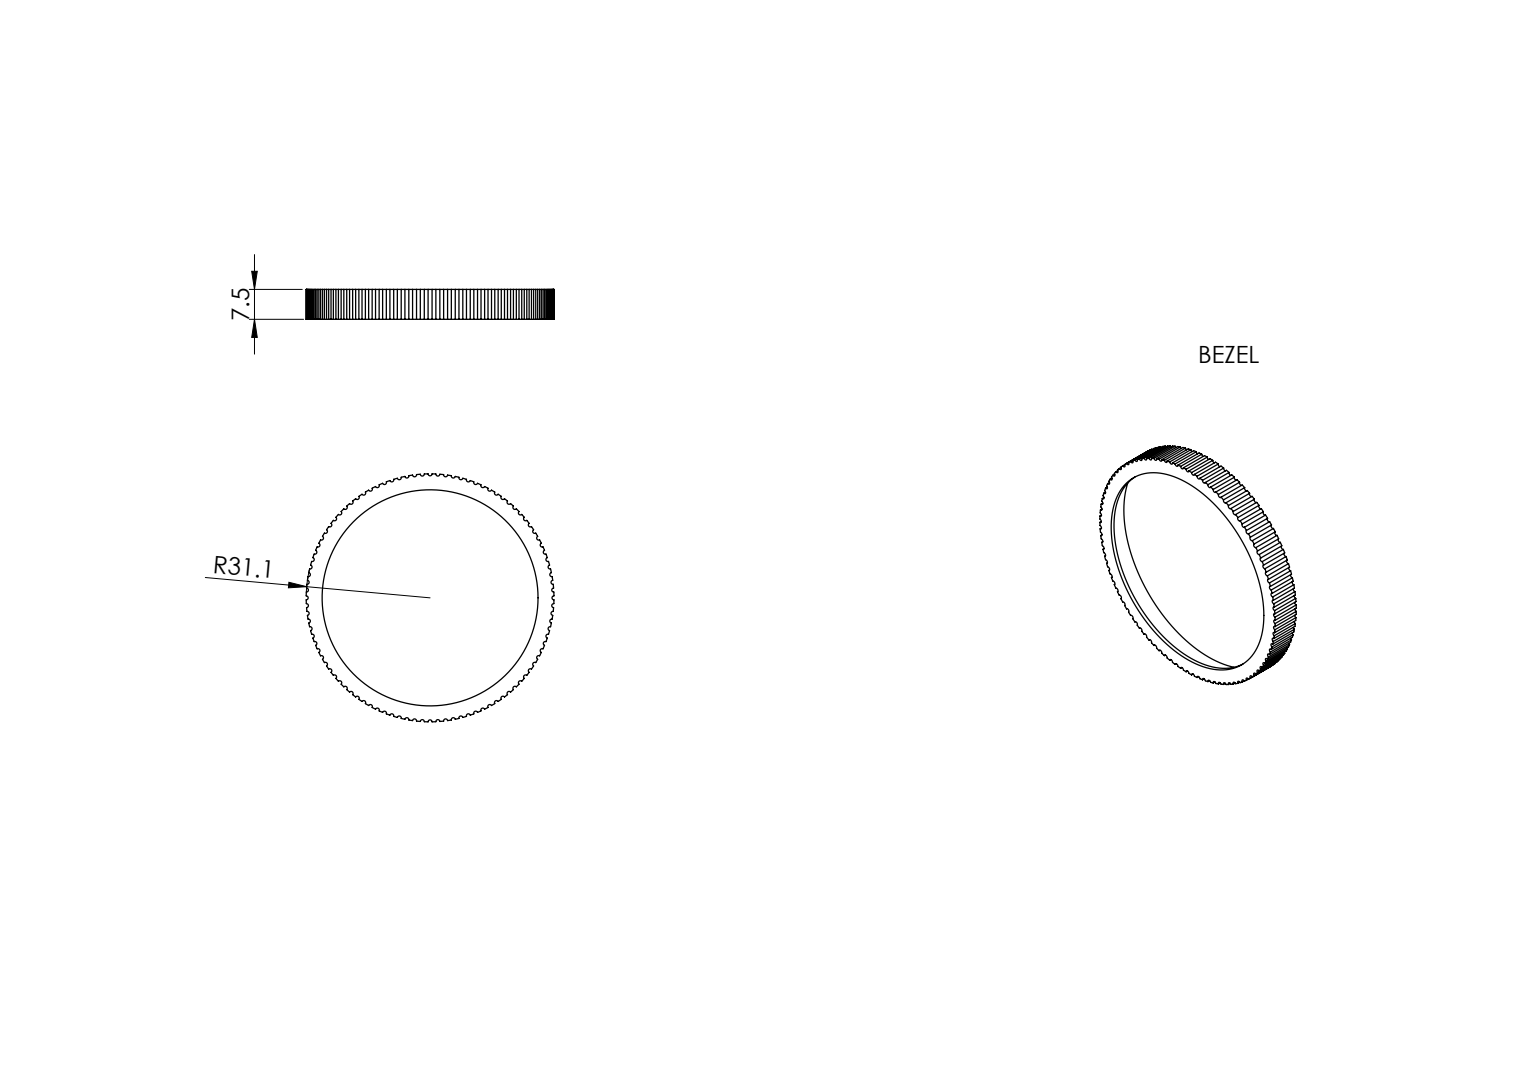
ISO-10303-21;
HEADER;
FILE_DESCRIPTION (('STEP AP214'),
    '1' );
FILE_NAME ('bezel.step',
    '2026-10-26T12:50:16',
    ( '' ),
    ( '' ),
    'SwSTEP 2.0',
    'SolidWorks 2026',
    '' );
FILE_SCHEMA (( 'AUTOMOTIVE_DESIGN' ));
ENDSEC;

DATA;
#1=AXIS2_PLACEMENT_3D ( 'NONE', #24942, #2719, #13181 ) ;
#6=AXIS2_PLACEMENT_3D ( 'NONE', #4398, #870, #8851 ) ;
#12=DIRECTION ( 'NONE',  ( 1.000000000000000000, 0.000000000000000000, 0.000000000000000000 ) ) ;
#17=CIRCLE ( 'NONE', #17974, 0.5000000000000003331 ) ;
#18=CARTESIAN_POINT ( 'NONE',  ( 0.000000000000000000, 0.000000000000000000, 1.000000000000000000 ) ) ;
#20=ORIENTED_EDGE ( 'NONE', *, *, #7327, .F. ) ;
#25=ORIENTED_EDGE ( 'NONE', *, *, #21709, .F. ) ;
#27=VERTEX_POINT ( 'NONE', #19559 ) ;
#31=AXIS2_PLACEMENT_3D ( 'NONE', #2511, #8267, #24218 ) ;
#35=CIRCLE ( 'NONE', #17990, 0.5000000000000006661 ) ;
#39=CIRCLE ( 'NONE', #22153, 31.10000000000000142 ) ;
#47=CIRCLE ( 'NONE', #3373, 31.10000000000000142 ) ;
#49=CARTESIAN_POINT ( 'NONE',  ( -10.98232076577242466, -29.09636799667071116, 1.000000000000000000 ) ) ;
#51=VERTEX_POINT ( 'NONE', #10384 ) ;
#54=EDGE_CURVE ( 'NONE', #21865, #6150, #14230, .T. ) ;
#55=CIRCLE ( 'NONE', #14670, 0.5000000000000005551 ) ;
#60=CARTESIAN_POINT ( 'NONE',  ( -9.610428525061097460, -29.57785765677920509, -6.500000000000000000 ) ) ;
#63=VECTOR ( 'NONE', #7567, 1000.000000000000000 ) ;
#66=DIRECTION ( 'NONE',  ( 0.000000000000000000, 0.000000000000000000, 1.000000000000000000 ) ) ;
#70=AXIS2_PLACEMENT_3D ( 'NONE', #11835, #22027, #12224 ) ;
#72=DIRECTION ( 'NONE',  ( 1.000000000000000000, 0.000000000000000000, 0.000000000000000000 ) ) ;
#79=AXIS2_PLACEMENT_3D ( 'NONE', #15726, #13515, #3680 ) ;
#81=DIRECTION ( 'NONE',  ( 0.000000000000000000, 0.000000000000000000, 1.000000000000000000 ) ) ;
#83=CARTESIAN_POINT ( 'NONE',  ( -23.01025686871652809, -20.92219106202034595, 1.000000000000000000 ) ) ;
#86=CIRCLE ( 'NONE', #1339, 31.10000000000000142 ) ;
#89=VERTEX_POINT ( 'NONE', #21923 ) ;
#95=AXIS2_PLACEMENT_3D ( 'NONE', #9918, #10180, #22078 ) ;
#97=CYLINDRICAL_SURFACE ( 'NONE', #3366, 0.5000000000000004441 ) ;
#98=ORIENTED_EDGE ( 'NONE', *, *, #19921, .T. ) ;
#99=ORIENTED_EDGE ( 'NONE', *, *, #21927, .F. ) ;
#100=ADVANCED_FACE ( 'NONE', ( #14466 ), #6356, .T. ) ;
#105=EDGE_CURVE ( 'NONE', #8835, #13216, #4631, .T. ) ;
#106=CIRCLE ( 'NONE', #18070, 0.4999999999999998890 ) ;
#107=EDGE_CURVE ( 'NONE', #585, #4269, #18005, .T. ) ;
#112=AXIS2_PLACEMENT_3D ( 'NONE', #10691, #2608, #22745 ) ;
#117=ORIENTED_EDGE ( 'NONE', *, *, #18852, .F. ) ;
#129=DIRECTION ( 'NONE',  ( 1.000000000000000000, 0.000000000000000000, 0.000000000000000000 ) ) ;
#131=ORIENTED_EDGE ( 'NONE', *, *, #19522, .T. ) ;
#132=VERTEX_POINT ( 'NONE', #22432 ) ;
#134=DIRECTION ( 'NONE',  ( 0.2486898871648519360, -0.9685831611286318532, 0.000000000000000000 ) ) ;
#135=LINE ( 'NONE', #23787, #14039 ) ;
#136=EDGE_CURVE ( 'NONE', #11885, #9403, #6717, .T. ) ;
#138=CARTESIAN_POINT ( 'NONE',  ( 22.67092431280594056, 21.28941499438218088, 1.000000000000000000 ) ) ;
#145=DIRECTION ( 'NONE',  ( 0.000000000000000000, 0.000000000000000000, -1.000000000000000000 ) ) ;
#146=LINE ( 'NONE', #8118, #8436 ) ;
#147=CIRCLE ( 'NONE', #18512, 0.4999999999999997224 ) ;
#151=DIRECTION ( 'NONE',  ( -0.000000000000000000, 0.000000000000000000, 1.000000000000000000 ) ) ;
#154=AXIS2_PLACEMENT_3D ( 'NONE', #12888, #20866, #10658 ) ;
#157=ORIENTED_EDGE ( 'NONE', *, *, #19996, .F. ) ;
#158=DIRECTION ( 'NONE',  ( 0.4817536741017267032, 0.8763066800438573667, 0.000000000000000000 ) ) ;
#161=VERTEX_POINT ( 'NONE', #10530 ) ;
#163=ORIENTED_EDGE ( 'NONE', *, *, #23989, .T. ) ;
#164=ORIENTED_EDGE ( 'NONE', *, *, #21623, .F. ) ;
#169=CIRCLE ( 'NONE', #23535, 31.10000000000000142 ) ;
#170=EDGE_CURVE ( 'NONE', #5115, #14942, #12104, .T. ) ;
#179=DIRECTION ( 'NONE',  ( -0.000000000000000000, 0.000000000000000000, -1.000000000000000000 ) ) ;
#183=ORIENTED_EDGE ( 'NONE', *, *, #8865, .T. ) ;
#184=VERTEX_POINT ( 'NONE', #16301 ) ;
#187=DIRECTION ( 'NONE',  ( -0.000000000000000000, -0.000000000000000000, 1.000000000000000000 ) ) ;
#190=DIRECTION ( 'NONE',  ( -0.2486898871648584586, -0.9685831611286301879, 0.000000000000000000 ) ) ;
#191=ORIENTED_EDGE ( 'NONE', *, *, #21291, .T. ) ;
#193=ORIENTED_EDGE ( 'NONE', *, *, #13144, .T. ) ;
#199=DIRECTION ( 'NONE',  ( 0.000000000000000000, 0.000000000000000000, 1.000000000000000000 ) ) ;
#207=CARTESIAN_POINT ( 'NONE',  ( -30.85476721088022600, 3.897863563850190616, 1.000000000000000000 ) ) ;
#208=EDGE_CURVE ( 'NONE', #13339, #3186, #993, .T. ) ;
#209=DIRECTION ( 'NONE',  ( 0.000000000000000000, -0.000000000000000000, -1.000000000000000000 ) ) ;
#211=DIRECTION ( 'NONE',  ( 0.000000000000000000, -0.000000000000000000, 1.000000000000000000 ) ) ;
#226=DIRECTION ( 'NONE',  ( 0.000000000000000000, 0.000000000000000000, 1.000000000000000000 ) ) ;
#232=CARTESIAN_POINT ( 'NONE',  ( -30.12293631110050995, -7.734255490826679846, 1.000000000000000000 ) ) ;
#233=DIRECTION ( 'NONE',  ( 1.000000000000000000, 0.000000000000000000, 0.000000000000000000 ) ) ;
#239=EDGE_CURVE ( 'NONE', #21040, #20500, #15911, .T. ) ;
#240=ORIENTED_EDGE ( 'NONE', *, *, #11799, .T. ) ;
#242=FACE_OUTER_BOUND ( 'NONE', #14530, .T. ) ;
#244=ADVANCED_FACE ( 'NONE', ( #5041 ), #15120, .T. ) ;
#246=VERTEX_POINT ( 'NONE', #19148 ) ;
#250=ORIENTED_EDGE ( 'NONE', *, *, #20339, .T. ) ;
#252=CARTESIAN_POINT ( 'NONE',  ( 13.69242354489153080, 27.92360179968372691, -6.500000000000000000 ) ) ;
#254=DIRECTION ( 'NONE',  ( 0.000000000000000000, 0.000000000000000000, 1.000000000000000000 ) ) ;
#255=ORIENTED_EDGE ( 'NONE', *, *, #13059, .F. ) ;
#257=ORIENTED_EDGE ( 'NONE', *, *, #741, .T. ) ;
#259=CIRCLE ( 'NONE', #6931, 0.4999999999999998335 ) ;
#260=ORIENTED_EDGE ( 'NONE', *, *, #5301, .F. ) ;
#261=CARTESIAN_POINT ( 'NONE',  ( -10.08469938919519926, -29.41953157733083302, -6.500000000000000000 ) ) ;
#268=CARTESIAN_POINT ( 'NONE',  ( -29.57785765677917311, 9.610428525061202265, -6.500000000000000000 ) ) ;
#272=CARTESIAN_POINT ( 'NONE',  ( -23.96296185032681336, 19.82388608118453632, 1.000000000000000000 ) ) ;
#273=CARTESIAN_POINT ( 'NONE',  ( -19.82388608118446527, -23.96296185032687376, -6.500000000000000000 ) ) ;
#276=DIRECTION ( 'NONE',  ( 1.000000000000000000, 0.000000000000000000, 0.000000000000000000 ) ) ;
#281=ORIENTED_EDGE ( 'NONE', *, *, #13641, .F. ) ;
#286=ORIENTED_EDGE ( 'NONE', *, *, #2780, .F. ) ;
#289=CARTESIAN_POINT ( 'NONE',  ( 29.09636799667075024, -10.98232076577232519, -2.750000000000000000 ) ) ;
#296=LINE ( 'NONE', #16630, #5040 ) ;
#297=DIRECTION ( 'NONE',  ( 0.000000000000000000, -0.000000000000000000, 1.000000000000000000 ) ) ;
#299=DIRECTION ( 'NONE',  ( 1.000000000000000000, 0.000000000000000000, 0.000000000000000000 ) ) ;
#303=DIRECTION ( 'NONE',  ( 1.000000000000000000, 0.000000000000000000, 0.000000000000000000 ) ) ;
#306=EDGE_LOOP ( 'NONE', ( #6770, #6578, #10344, #18560 ) ) ;
#308=EDGE_CURVE ( 'NONE', #5737, #11616, #8580, .T. ) ;
#309=ORIENTED_EDGE ( 'NONE', *, *, #9443, .F. ) ;
#310=DIRECTION ( 'NONE',  ( 0.000000000000000000, -0.000000000000000000, 1.000000000000000000 ) ) ;
#313=ORIENTED_EDGE ( 'NONE', *, *, #21775, .T. ) ;
#317=DIRECTION ( 'NONE',  ( -0.000000000000000000, -0.000000000000000000, 1.000000000000000000 ) ) ;
#320=DIRECTION ( 'NONE',  ( 0.000000000000000000, 0.000000000000000000, 1.000000000000000000 ) ) ;
#321=FACE_OUTER_BOUND ( 'NONE', #5229, .T. ) ;
#326=CYLINDRICAL_SURFACE ( 'NONE', #16421, 0.5000000000000004441 ) ;
#327=DIRECTION ( 'NONE',  ( -0.000000000000000000, -0.000000000000000000, 1.000000000000000000 ) ) ;
#330=EDGE_CURVE ( 'NONE', #22681, #23712, #2540, .T. ) ;
#332=CARTESIAN_POINT ( 'NONE',  ( 0.000000000000000000, 0.000000000000000000, -6.500000000000000000 ) ) ;
#343=AXIS2_PLACEMENT_3D ( 'NONE', #22234, #14397, #10312 ) ;
#346=ORIENTED_EDGE ( 'NONE', *, *, #25545, .F. ) ;
#349=DIRECTION ( 'NONE',  ( -0.000000000000000000, -0.000000000000000000, 1.000000000000000000 ) ) ;
#351=ADVANCED_FACE ( 'NONE', ( #18768 ), #8839, .F. ) ;
#354=CARTESIAN_POINT ( 'NONE',  ( 18.68225429291731743, 24.86329371854767700, -2.750000000000000000 ) ) ;
#357=CARTESIAN_POINT ( 'NONE',  ( 0.000000000000000000, 0.000000000000000000, 0.000000000000000000 ) ) ;
#359=CARTESIAN_POINT ( 'NONE',  ( -28.41604871112473418, -11.44867358849319849, 1.000000000000000000 ) ) ;
#362=EDGE_CURVE ( 'NONE', #3397, #1343, #25563, .T. ) ;
#364=VERTEX_POINT ( 'NONE', #23208 ) ;
#366=CYLINDRICAL_SURFACE ( 'NONE', #12999, 31.10000000000000142 ) ;
#372=ORIENTED_EDGE ( 'NONE', *, *, #5336, .T. ) ;
#376=CARTESIAN_POINT ( 'NONE',  ( 0.000000000000000000, 0.000000000000000000, 1.000000000000000000 ) ) ;
#379=AXIS2_PLACEMENT_3D ( 'NONE', #21267, #11325, #1788 ) ;
#382=AXIS2_PLACEMENT_3D ( 'NONE', #14480, #16700, #6759 ) ;
#383=VERTEX_POINT ( 'NONE', #19283 ) ;
#387=CIRCLE ( 'NONE', #2056, 31.10000000000000142 ) ;
#390=EDGE_CURVE ( 'NONE', #22273, #20492, #21386, .T. ) ;
#394=CARTESIAN_POINT ( 'NONE',  ( 15.41874213889396117, -27.00874656207311020, 1.000000000000000000 ) ) ;
#395=AXIS2_PLACEMENT_3D ( 'NONE', #11615, #6002, #7707 ) ;
#396=CARTESIAN_POINT ( 'NONE',  ( 0.000000000000000000, 31.10000000000000142, -6.500000000000000000 ) ) ;
#399=DIRECTION ( 'NONE',  ( 1.000000000000000000, 0.000000000000000000, 0.000000000000000000 ) ) ;
#402=FACE_OUTER_BOUND ( 'NONE', #9294, .T. ) ;
#403=AXIS2_PLACEMENT_3D ( 'NONE', #22410, #18239, #9988 ) ;
#405=AXIS2_PLACEMENT_3D ( 'NONE', #13535, #2006, #15875 ) ;
#406=LINE ( 'NONE', #6283, #17518 ) ;
#407=CARTESIAN_POINT ( 'NONE',  ( -22.17092431280563503, 21.28941499438250062, -6.500000000000000000 ) ) ;
#411=ORIENTED_EDGE ( 'NONE', *, *, #12740, .F. ) ;
#414=VERTEX_POINT ( 'NONE', #11303 ) ;
#416=ORIENTED_EDGE ( 'NONE', *, *, #10693, .T. ) ;
#417=ORIENTED_EDGE ( 'NONE', *, *, #13846, .T. ) ;
#419=CIRCLE ( 'NONE', #13349, 31.10000000000000142 ) ;
#420=AXIS2_PLACEMENT_3D ( 'NONE', #4845, #24723, #6933 ) ;
#422=EDGE_CURVE ( 'NONE', #16170, #9403, #21906, .T. ) ;
#425=AXIS2_PLACEMENT_3D ( 'NONE', #20340, #2434, #1117 ) ;
#427=AXIS2_PLACEMENT_3D ( 'NONE', #1473, #13891, #21596 ) ;
#431=EDGE_CURVE ( 'NONE', #13647, #11427, #23332, .T. ) ;
#432=DIRECTION ( 'NONE',  ( -0.000000000000000000, -0.000000000000000000, 1.000000000000000000 ) ) ;
#433=AXIS2_PLACEMENT_3D ( 'NONE', #24646, #6868, #8833 ) ;
#436=LINE ( 'NONE', #14425, #4662 ) ;
#438=CIRCLE ( 'NONE', #9607, 0.4999999999999996114 ) ;
#441=VECTOR ( 'NONE', #4538, 1000.000000000000000 ) ;
#442=CARTESIAN_POINT ( 'NONE',  ( -3.897863563849436552, 30.85476721088031482, -6.500000000000000000 ) ) ;
#443=ORIENTED_EDGE ( 'NONE', *, *, #15873, .T. ) ;
#444=ORIENTED_EDGE ( 'NONE', *, *, #3058, .F. ) ;
#448=EDGE_LOOP ( 'NONE', ( #16828, #9714, #24335, #4332 ) ) ;
#450=ORIENTED_EDGE ( 'NONE', *, *, #18741, .F. ) ;
#451=DIRECTION ( 'NONE',  ( 0.7705132427757999114, 0.6374239897486768669, 0.000000000000000000 ) ) ;
#452=CARTESIAN_POINT ( 'NONE',  ( -31.03863125411922752, 1.952785157361987878, -6.500000000000000000 ) ) ;
#453=AXIS2_PLACEMENT_3D ( 'NONE', #20208, #10264, #5925 ) ;
#456=ADVANCED_FACE ( 'NONE', ( #9600 ), #3466, .T. ) ;
#460=EDGE_CURVE ( 'NONE', #51, #5651, #19861, .T. ) ;
#464=DIRECTION ( 'NONE',  ( -0.000000000000000000, -0.000000000000000000, 1.000000000000000000 ) ) ;
#472=VECTOR ( 'NONE', #23351, 1000.000000000000000 ) ;
#474=CIRCLE ( 'NONE', #15093, 0.4999999999999989453 ) ;
#480=ORIENTED_EDGE ( 'NONE', *, *, #22688, .F. ) ;
#483=CIRCLE ( 'NONE', #7586, 0.4999999999999987232 ) ;
#484=DIRECTION ( 'NONE',  ( -0.9685831611286283005, 0.2486898871648657861, 0.000000000000000000 ) ) ;
#485=VERTEX_POINT ( 'NONE', #25421 ) ;
#489=FACE_OUTER_BOUND ( 'NONE', #1615, .T. ) ;
#490=CYLINDRICAL_SURFACE ( 'NONE', #24782, 0.5000000000000004441 ) ;
#491=AXIS2_PLACEMENT_3D ( 'NONE', #8684, #8567, #22819 ) ;
#492=CIRCLE ( 'NONE', #3822, 0.5000000000000004441 ) ;
#493=ADVANCED_FACE ( 'NONE', ( #21765 ), #11688, .F. ) ;
#497=VECTOR ( 'NONE', #179, 1000.000000000000000 ) ;
#498=DIRECTION ( 'NONE',  ( 1.000000000000000000, 0.000000000000000000, 0.000000000000000000 ) ) ;
#500=CARTESIAN_POINT ( 'NONE',  ( -10.08469938919507847, -29.41953157733087565, 1.000000000000000000 ) ) ;
#507=ORIENTED_EDGE ( 'NONE', *, *, #9146, .T. ) ;
#510=EDGE_LOOP ( 'NONE', ( #14113, #25279, #16262, #2593 ) ) ;
#512=LINE ( 'NONE', #2595, #15256 ) ;
#515=ORIENTED_EDGE ( 'NONE', *, *, #15269, .F. ) ;
#516=AXIS2_PLACEMENT_3D ( 'NONE', #10572, #16873, #22870 ) ;
#519=ORIENTED_EDGE ( 'NONE', *, *, #19200, .F. ) ;
#521=ORIENTED_EDGE ( 'NONE', *, *, #2339, .F. ) ;
#527=CIRCLE ( 'NONE', #22224, 31.10000000000000142 ) ;
#532=EDGE_CURVE ( 'NONE', #18639, #8603, #9423, .T. ) ;
#533=DIRECTION ( 'NONE',  ( 1.000000000000000000, 0.000000000000000000, 0.000000000000000000 ) ) ;
#534=CARTESIAN_POINT ( 'NONE',  ( -6.317933499822993682, 30.45149776762736593, -6.500000000000000000 ) ) ;
#538=DIRECTION ( 'NONE',  ( 0.000000000000000000, 0.000000000000000000, 1.000000000000000000 ) ) ;
#539=EDGE_CURVE ( 'NONE', #19632, #14821, #9847, .T. ) ;
#541=CARTESIAN_POINT ( 'NONE',  ( -25.75859848311247902, 16.66421332384710752, -6.500000000000000000 ) ) ;
#547=CARTESIAN_POINT ( 'NONE',  ( -3.401318489840662540, 30.91344420362552015, -2.750000000000000000 ) ) ;
#549=ORIENTED_EDGE ( 'NONE', *, *, #7631, .F. ) ;
#550=ORIENTED_EDGE ( 'NONE', *, *, #1133, .T. ) ;
#552=ORIENTED_EDGE ( 'NONE', *, *, #7442, .T. ) ;
#553=ORIENTED_EDGE ( 'NONE', *, *, #15758, .T. ) ;
#554=ORIENTED_EDGE ( 'NONE', *, *, #16174, .F. ) ;
#560=CIRCLE ( 'NONE', #21439, 0.5000000000000005551 ) ;
#562=CARTESIAN_POINT ( 'NONE',  ( -8.217531866530787710, 29.99470236596041772, -2.750000000000000000 ) ) ;
#564=CARTESIAN_POINT ( 'NONE',  ( -28.91604871112448549, 11.44867358849382910, -6.500000000000000000 ) ) ;
#565=AXIS2_PLACEMENT_3D ( 'NONE', #15634, #17845, #20049 ) ;
#571=DIRECTION ( 'NONE',  ( 1.000000000000000000, 0.000000000000000000, 0.000000000000000000 ) ) ;
#575=ORIENTED_EDGE ( 'NONE', *, *, #4755, .F. ) ;
#576=EDGE_CURVE ( 'NONE', #5530, #3462, #15285, .T. ) ;
#577=EDGE_LOOP ( 'NONE', ( #12034, #4407, #15009, #19434 ) ) ;
#579=EDGE_CURVE ( 'NONE', #21691, #25452, #21965, .T. ) ;
#583=VERTEX_POINT ( 'NONE', #20304 ) ;
#585=VERTEX_POINT ( 'NONE', #10235 ) ;
#588=CARTESIAN_POINT ( 'NONE',  ( 22.67092431280578779, -21.28941499438234786, -6.500000000000000000 ) ) ;
#593=DIRECTION ( 'NONE',  ( -0.000000000000000000, 0.000000000000000000, 1.000000000000000000 ) ) ;
#595=( GEOMETRIC_REPRESENTATION_CONTEXT ( 3 ) GLOBAL_UNCERTAINTY_ASSIGNED_CONTEXT ( ( #8894 ) ) GLOBAL_UNIT_ASSIGNED_CONTEXT ( ( #1543, #19329, #25603 ) ) REPRESENTATION_CONTEXT ( 'NONE', 'WORKASPACE' ) );
#606=ORIENTED_EDGE ( 'NONE', *, *, #13099, .F. ) ;
#610=ORIENTED_EDGE ( 'NONE', *, *, #15078, .F. ) ;
#612=DIRECTION ( 'NONE',  ( 0.000000000000000000, 0.000000000000000000, 1.000000000000000000 ) ) ;
#615=ORIENTED_EDGE ( 'NONE', *, *, #13996, .T. ) ;
#616=ORIENTED_EDGE ( 'NONE', *, *, #17721, .F. ) ;
#624=FACE_OUTER_BOUND ( 'NONE', #15797, .T. ) ;
#625=DIRECTION ( 'NONE',  ( 1.000000000000000000, 0.000000000000000000, 0.000000000000000000 ) ) ;
#634=CARTESIAN_POINT ( 'NONE',  ( -18.68225429291695860, 24.86329371854795056, -2.750000000000000000 ) ) ;
#635=ORIENTED_EDGE ( 'NONE', *, *, #10538, .T. ) ;
#641=CYLINDRICAL_SURFACE ( 'NONE', #13338, 0.5000000000000004441 ) ;
#642=EDGE_CURVE ( 'NONE', #8421, #20150, #12769, .T. ) ;
#643=ORIENTED_EDGE ( 'NONE', *, *, #9008, .T. ) ;
#647=DIRECTION ( 'NONE',  ( -0.000000000000000000, 0.000000000000000000, -1.000000000000000000 ) ) ;
#648=DIRECTION ( 'NONE',  ( -0.000000000000000000, -0.000000000000000000, 1.000000000000000000 ) ) ;
#650=CIRCLE ( 'NONE', #19423, 31.10000000000000142 ) ;
#655=LINE ( 'NONE', #10968, #1709 ) ;
#659=CARTESIAN_POINT ( 'NONE',  ( -28.91604871112473418, -11.44867358849319849, -6.500000000000000000 ) ) ;
#662=DIRECTION ( 'NONE',  ( -0.000000000000000000, -0.000000000000000000, 1.000000000000000000 ) ) ;
#666=ORIENTED_EDGE ( 'NONE', *, *, #17227, .T. ) ;
#672=VERTEX_POINT ( 'NONE', #12072 ) ;
#674=VERTEX_POINT ( 'NONE', #20047 ) ;
#675=CARTESIAN_POINT ( 'NONE',  ( 0.000000000000000000, 0.000000000000000000, -6.500000000000000000 ) ) ;
#678=AXIS2_PLACEMENT_3D ( 'NONE', #25811, #10355, #2014 ) ;
#679=ADVANCED_FACE ( 'NONE', ( #8163 ), #16144, .T. ) ;
#680=CARTESIAN_POINT ( 'NONE',  ( 0.000000000000000000, 0.000000000000000000, -6.500000000000000000 ) ) ;
#685=ADVANCED_FACE ( 'NONE', ( #14177 ), #22147, .F. ) ;
#690=FACE_OUTER_BOUND ( 'NONE', #16797, .T. ) ;
#691=CARTESIAN_POINT ( 'NONE',  ( -18.28012134629613783, -25.16042852506070560, -6.500000000000000000 ) ) ;
#692=CYLINDRICAL_SURFACE ( 'NONE', #17204, 0.5000000000000002220 ) ;
#693=DIRECTION ( 'NONE',  ( 0.000000000000000000, 0.000000000000000000, 1.000000000000000000 ) ) ;
#700=EDGE_LOOP ( 'NONE', ( #21687, #12958, #18424, #6447 ) ) ;
#701=DIRECTION ( 'NONE',  ( 0.06279051952932236669, 0.9980267284282710039, 0.000000000000000000 ) ) ;
#703=ORIENTED_EDGE ( 'NONE', *, *, #17786, .T. ) ;
#707=EDGE_CURVE ( 'NONE', #19701, #5616, #22374, .T. ) ;
#722=EDGE_LOOP ( 'NONE', ( #1470, #16759, #21538, #23056 ) ) ;
#725=DIRECTION ( 'NONE',  ( -0.000000000000000000, -0.000000000000000000, -1.000000000000000000 ) ) ;
#726=ORIENTED_EDGE ( 'NONE', *, *, #19375, .T. ) ;
#727=ORIENTED_EDGE ( 'NONE', *, *, #13164, .F. ) ;
#730=ORIENTED_EDGE ( 'NONE', *, *, #5993, .T. ) ;
#732=LINE ( 'NONE', #6998, #10114 ) ;
#733=DIRECTION ( 'NONE',  ( 0.000000000000000000, 0.000000000000000000, 1.000000000000000000 ) ) ;
#736=ADVANCED_FACE ( 'NONE', ( #18500 ), #8555, .F. ) ;
#740=CARTESIAN_POINT ( 'NONE',  ( -28.91604871112473418, -11.44867358849319849, -6.500000000000000000 ) ) ;
#741=EDGE_CURVE ( 'NONE', #14667, #12275, #23629, .T. ) ;
#742=CARTESIAN_POINT ( 'NONE',  ( -30.54913349766215802, 5.827558883616378083, -6.500000000000000000 ) ) ;
#743=FACE_OUTER_BOUND ( 'NONE', #23538, .T. ) ;
#750=DIRECTION ( 'NONE',  ( 0.000000000000000000, 0.000000000000000000, -1.000000000000000000 ) ) ;
#754=DIRECTION ( 'NONE',  ( 0.9921147013144777649, -0.1253332335643050077, 0.000000000000000000 ) ) ;
#757=CARTESIAN_POINT ( 'NONE',  ( -23.96296185032722548, -19.82388608118403539, -6.500000000000000000 ) ) ;
#758=EDGE_LOOP ( 'NONE', ( #1820, #6628, #21819, #13928 ) ) ;
#762=EDGE_LOOP ( 'NONE', ( #22709, #20677, #24398, #5708 ) ) ;
#766=AXIS2_PLACEMENT_3D ( 'NONE', #19619, #9699, #1586 ) ;
#771=LINE ( 'NONE', #23004, #7188 ) ;
#773=DIRECTION ( 'NONE',  ( 0.000000000000000000, 0.000000000000000000, 1.000000000000000000 ) ) ;
#781=DIRECTION ( 'NONE',  ( -0.8763066800438602533, 0.4817536741017213187, 0.000000000000000000 ) ) ;
#782=EDGE_CURVE ( 'NONE', #17013, #7673, #14861, .T. ) ;
#787=DIRECTION ( 'NONE',  ( 0.000000000000000000, 0.000000000000000000, 1.000000000000000000 ) ) ;
#788=DIRECTION ( 'NONE',  ( -0.000000000000000000, -0.000000000000000000, 1.000000000000000000 ) ) ;
#789=VERTEX_POINT ( 'NONE', #1451 ) ;
#791=ORIENTED_EDGE ( 'NONE', *, *, #22163, .F. ) ;
#793=ORIENTED_EDGE ( 'NONE', *, *, #4739, .F. ) ;
#795=ORIENTED_EDGE ( 'NONE', *, *, #23095, .F. ) ;
#800=AXIS2_PLACEMENT_3D ( 'NONE', #15650, #15525, #5578 ) ;
#802=AXIS2_PLACEMENT_3D ( 'NONE', #2935, #3450, #11424 ) ;
#807=AXIS2_PLACEMENT_3D ( 'NONE', #14101, #23650, #10169 ) ;
#812=CARTESIAN_POINT ( 'NONE',  ( 0.000000000000000000, 0.000000000000000000, -6.500000000000000000 ) ) ;
#817=ORIENTED_EDGE ( 'NONE', *, *, #17018, .F. ) ;
#818=ORIENTED_EDGE ( 'NONE', *, *, #7336, .T. ) ;
#821=AXIS2_PLACEMENT_3D ( 'NONE', #376, #22462, #6254 ) ;
#822=VERTEX_POINT ( 'NONE', #12458 ) ;
#823=DIRECTION ( 'NONE',  ( -0.1873813145857119722, 0.9822872507286911636, 0.000000000000000000 ) ) ;
#824=ORIENTED_EDGE ( 'NONE', *, *, #17375, .F. ) ;
#826=EDGE_LOOP ( 'NONE', ( #3312, #6963, #2563, #11339 ) ) ;
#829=VECTOR ( 'NONE', #20995, 1000.000000000000000 ) ;
#831=FACE_OUTER_BOUND ( 'NONE', #14793, .T. ) ;
#838=AXIS2_PLACEMENT_3D ( 'NONE', #8930, #15201, #10864 ) ;
#840=AXIS2_PLACEMENT_3D ( 'NONE', #2316, #10272, #20617 ) ;
#844=ORIENTED_EDGE ( 'NONE', *, *, #18813, .T. ) ;
#846=EDGE_CURVE ( 'NONE', #3229, #3397, #21536, .T. ) ;
#853=EDGE_CURVE ( 'NONE', #12237, #5263, #24888, .T. ) ;
#854=DIRECTION ( 'NONE',  ( 0.000000000000000000, 0.000000000000000000, 1.000000000000000000 ) ) ;
#858=AXIS2_PLACEMENT_3D ( 'NONE', #20378, #18188, #10066 ) ;
#859=AXIS2_PLACEMENT_3D ( 'NONE', #19011, #19263, #3062 ) ;
#868=CARTESIAN_POINT ( 'NONE',  ( -29.07785765677936851, -9.610428525060582317, 1.000000000000000000 ) ) ;
#869=AXIS2_PLACEMENT_3D ( 'NONE', #5265, #13243, #18616 ) ;
#870=DIRECTION ( 'NONE',  ( -0.000000000000000000, -0.000000000000000000, 1.000000000000000000 ) ) ;
#873=CARTESIAN_POINT ( 'NONE',  ( 0.000000000000000000, 0.000000000000000000, -6.500000000000000000 ) ) ;
#875=DIRECTION ( 'NONE',  ( 0.000000000000000000, 0.000000000000000000, 1.000000000000000000 ) ) ;
#878=VECTOR ( 'NONE', #2181, 1000.000000000000000 ) ;
#880=CYLINDRICAL_SURFACE ( 'NONE', #7552, 0.5000000000000000000 ) ;
#886=ORIENTED_EDGE ( 'NONE', *, *, #2903, .T. ) ;
#887=CARTESIAN_POINT ( 'NONE',  ( -25.75859848311247902, 16.66421332384710752, -6.500000000000000000 ) ) ;
#890=ADVANCED_FACE ( 'NONE', ( #11377 ), #19355, .T. ) ;
#892=ORIENTED_EDGE ( 'NONE', *, *, #8937, .F. ) ;
#893=DIRECTION ( 'NONE',  ( -0.000000000000000000, 0.000000000000000000, 1.000000000000000000 ) ) ;
#894=ADVANCED_FACE ( 'NONE', ( #19093 ), #20431, .F. ) ;
#895=EDGE_LOOP ( 'NONE', ( #13145, #10145, #12923, #16753 ) ) ;
#898=ORIENTED_EDGE ( 'NONE', *, *, #3464, .T. ) ;
#899=DIRECTION ( 'NONE',  ( 1.000000000000000000, 0.000000000000000000, 0.000000000000000000 ) ) ;
#900=EDGE_CURVE ( 'NONE', #1141, #6126, #5120, .T. ) ;
#901=CIRCLE ( 'NONE', #10903, 0.5000000000000009992 ) ;
#903=VECTOR ( 'NONE', #4470, 1000.000000000000000 ) ;
#904=DIRECTION ( 'NONE',  ( 0.000000000000000000, 0.000000000000000000, 1.000000000000000000 ) ) ;
#906=VECTOR ( 'NONE', #5433, 1000.000000000000000 ) ;
#907=EDGE_CURVE ( 'NONE', #21795, #24486, #23214, .T. ) ;
#915=DIRECTION ( 'NONE',  ( 0.000000000000000000, -0.000000000000000000, -1.000000000000000000 ) ) ;
#922=AXIS2_PLACEMENT_3D ( 'NONE', #15072, #2899, #7219 ) ;
#923=DIRECTION ( 'NONE',  ( -0.000000000000000000, -0.000000000000000000, 1.000000000000000000 ) ) ;
#928=LINE ( 'NONE', #2364, #18787 ) ;
#929=CARTESIAN_POINT ( 'NONE',  ( 23.96296185032708337, 19.82388608118420237, -6.500000000000000000 ) ) ;
#931=CIRCLE ( 'NONE', #15119, 0.5000000000000019984 ) ;
#932=EDGE_CURVE ( 'NONE', #17398, #3560, #135, .T. ) ;
#937=CARTESIAN_POINT ( 'NONE',  ( 0.000000000000000000, 0.000000000000000000, -6.500000000000000000 ) ) ;
#938=CIRCLE ( 'NONE', #13461, 31.10000000000000142 ) ;
#942=AXIS2_PLACEMENT_3D ( 'NONE', #11479, #21672, #15167 ) ;
#943=CIRCLE ( 'NONE', #12616, 0.4999999999999999445 ) ;
#944=ADVANCED_FACE ( 'NONE', ( #7714 ), #1569, .T. ) ;
#955=CARTESIAN_POINT ( 'NONE',  ( -8.217531866530787710, 29.99470236596041772, 1.000000000000000000 ) ) ;
#956=CARTESIAN_POINT ( 'NONE',  ( 0.000000000000000000, 0.000000000000000000, 1.000000000000000000 ) ) ;
#959=DIRECTION ( 'NONE',  ( 1.000000000000000000, 0.000000000000000000, 0.000000000000000000 ) ) ;
#962=VERTEX_POINT ( 'NONE', #2085 ) ;
#964=ORIENTED_EDGE ( 'NONE', *, *, #14508, .T. ) ;
#968=CIRCLE ( 'NONE', #10980, 0.5000000000000004441 ) ;
#974=DIRECTION ( 'NONE',  ( 0.000000000000000000, 0.000000000000000000, -1.000000000000000000 ) ) ;
#975=CARTESIAN_POINT ( 'NONE',  ( 0.000000000000000000, 0.000000000000000000, -6.500000000000000000 ) ) ;
#977=DIRECTION ( 'NONE',  ( -0.000000000000000000, 0.000000000000000000, 1.000000000000000000 ) ) ;
#980=DIRECTION ( 'NONE',  ( 0.000000000000000000, 0.000000000000000000, 1.000000000000000000 ) ) ;
#985=DIRECTION ( 'NONE',  ( -0.000000000000000000, -0.000000000000000000, 1.000000000000000000 ) ) ;
#989=ORIENTED_EDGE ( 'NONE', *, *, #6792, .F. ) ;
#992=ADVANCED_FACE ( 'NONE', ( #17662 ), #3650, .T. ) ;
#993=LINE ( 'NONE', #11166, #22178 ) ;
#997=CARTESIAN_POINT ( 'NONE',  ( -3.897863563850083146, -30.85476721088024021, 1.000000000000000000 ) ) ;
#998=EDGE_CURVE ( 'NONE', #132, #22067, #11624, .T. ) ;
#999=DIRECTION ( 'NONE',  ( 0.000000000000000000, 0.000000000000000000, 1.000000000000000000 ) ) ;
#1001=EDGE_CURVE ( 'NONE', #24168, #16234, #15818, .T. ) ;
#1002=CIRCLE ( 'NONE', #15623, 0.4999999999999998335 ) ;
#1006=DIRECTION ( 'NONE',  ( -0.000000000000000000, -0.000000000000000000, 1.000000000000000000 ) ) ;
#1007=CARTESIAN_POINT ( 'NONE',  ( 27.25313774936409317, -14.98253926456347074, -6.500000000000000000 ) ) ;
#1012=CARTESIAN_POINT ( 'NONE',  ( -14.48253926456356666, -27.25313774936403988, 1.000000000000000000 ) ) ;
#1014=CARTESIAN_POINT ( 'NONE',  ( -15.41874213889422940, -27.00874656207295743, 1.000000000000000000 ) ) ;
#1018=DIRECTION ( 'NONE',  ( -0.000000000000000000, -0.000000000000000000, 1.000000000000000000 ) ) ;
#1023=DIRECTION ( 'NONE',  ( 0.000000000000000000, 0.000000000000000000, 1.000000000000000000 ) ) ;
#1024=ORIENTED_EDGE ( 'NONE', *, *, #18629, .T. ) ;
#1032=ADVANCED_FACE ( 'NONE', ( #13862, #15695 ), #16085, .F. ) ;
#1033=LINE ( 'NONE', #20513, #7659 ) ;
#1038=ADVANCED_FACE ( 'NONE', ( #8228 ), #2609, .F. ) ;
#1039=DIRECTION ( 'NONE',  ( 1.000000000000000000, 0.000000000000000000, 0.000000000000000000 ) ) ;
#1043=CARTESIAN_POINT ( 'NONE',  ( -5.827558883615604479, 30.54913349766230724, -6.500000000000000000 ) ) ;
#1045=DIRECTION ( 'NONE',  ( 0.000000000000000000, 0.000000000000000000, 1.000000000000000000 ) ) ;
#1050=DIRECTION ( 'NONE',  ( 0.000000000000000000, 0.000000000000000000, 1.000000000000000000 ) ) ;
#1051=VERTEX_POINT ( 'NONE', #12533 ) ;
#1052=CARTESIAN_POINT ( 'NONE',  ( -21.28941499438192864, 22.67092431280617859, -6.500000000000000000 ) ) ;
#1053=LINE ( 'NONE', #8910, #8748 ) ;
#1055=VERTEX_POINT ( 'NONE', #16202 ) ;
#1056=EDGE_LOOP ( 'NONE', ( #14111, #12304, #8307, #3326 ) ) ;
#1058=ORIENTED_EDGE ( 'NONE', *, *, #2728, .F. ) ;
#1060=CARTESIAN_POINT ( 'NONE',  ( 0.000000000000000000, 0.000000000000000000, -6.500000000000000000 ) ) ;
#1061=ORIENTED_EDGE ( 'NONE', *, *, #5924, .T. ) ;
#1069=CARTESIAN_POINT ( 'NONE',  ( 3.401318489840877923, -30.91344420362549528, -6.500000000000000000 ) ) ;
#1071=DIRECTION ( 'NONE',  ( 0.9048270524660195768, -0.4257792915650726040, 0.000000000000000000 ) ) ;
#1076=DIRECTION ( 'NONE',  ( 0.000000000000000000, 0.000000000000000000, 1.000000000000000000 ) ) ;
#1078=EDGE_LOOP ( 'NONE', ( #22669, #22210, #8277, #12671 ) ) ;
#1080=EDGE_LOOP ( 'NONE', ( #4196, #7067, #16369, #11365 ) ) ;
#1081=DIRECTION ( 'NONE',  ( 0.000000000000000000, 0.000000000000000000, 1.000000000000000000 ) ) ;
#1083=AXIS2_PLACEMENT_3D ( 'NONE', #15502, #9739, #17213 ) ;
#1086=DIRECTION ( 'NONE',  ( 1.000000000000000000, 0.000000000000000000, 0.000000000000000000 ) ) ;
#1088=CARTESIAN_POINT ( 'NONE',  ( 18.28012134629577190, -25.16042852506097205, 1.000000000000000000 ) ) ;
#1090=CARTESIAN_POINT ( 'NONE',  ( -31.03863125411927371, -1.952785157361310198, -6.500000000000000000 ) ) ;
#1099=ORIENTED_EDGE ( 'NONE', *, *, #1162, .T. ) ;
#1102=ADVANCED_FACE ( 'NONE', ( #24794 ), #25186, .F. ) ;
#1107=ORIENTED_EDGE ( 'NONE', *, *, #2812, .T. ) ;
#1109=LINE ( 'NONE', #15243, #13742 ) ;
#1117=DIRECTION ( 'NONE',  ( 0.9685831611286301879, -0.2486898871648584586, 0.000000000000000000 ) ) ;
#1121=LINE ( 'NONE', #3476, #23861 ) ;
#1122=EDGE_CURVE ( 'NONE', #18910, #5387, #12620, .T. ) ;
#1133=EDGE_CURVE ( 'NONE', #25152, #672, #3440, .T. ) ;
#1134=ORIENTED_EDGE ( 'NONE', *, *, #19392, .F. ) ;
#1141=VERTEX_POINT ( 'NONE', #3084 ) ;
#1145=ORIENTED_EDGE ( 'NONE', *, *, #19132, .F. ) ;
#1149=DIRECTION ( 'NONE',  ( 1.000000000000000000, 0.000000000000000000, 0.000000000000000000 ) ) ;
#1157=CYLINDRICAL_SURFACE ( 'NONE', #15557, 0.5000000000000004441 ) ;
#1158=DIRECTION ( 'NONE',  ( 0.8443279255020205154, 0.5358267949789882190, 0.000000000000000000 ) ) ;
#1162=EDGE_CURVE ( 'NONE', #7703, #23505, #732, .T. ) ;
#1165=ORIENTED_EDGE ( 'NONE', *, *, #15711, .T. ) ;
#1166=DIRECTION ( 'NONE',  ( 0.000000000000000000, 0.000000000000000000, 1.000000000000000000 ) ) ;
#1167=DIRECTION ( 'NONE',  ( 0.000000000000000000, 0.000000000000000000, 1.000000000000000000 ) ) ;
#1176=LINE ( 'NONE', #19354, #17236 ) ;
#1178=EDGE_CURVE ( 'NONE', #12169, #3229, #4908, .T. ) ;
#1179=AXIS2_PLACEMENT_3D ( 'NONE', #659, #8628, #6530 ) ;
#1186=VECTOR ( 'NONE', #9407, 1000.000000000000000 ) ;
#1189=CIRCLE ( 'NONE', #25014, 0.5000000000000002220 ) ;
#1190=DIRECTION ( 'NONE',  ( 0.000000000000000000, 0.000000000000000000, -1.000000000000000000 ) ) ;
#1195=AXIS2_PLACEMENT_3D ( 'NONE', #2275, #8944, #823 ) ;
#1196=DIRECTION ( 'NONE',  ( 1.000000000000000000, 0.000000000000000000, 0.000000000000000000 ) ) ;
#1200=DIRECTION ( 'NONE',  ( -0.000000000000000000, -0.000000000000000000, 1.000000000000000000 ) ) ;
#1202=ORIENTED_EDGE ( 'NONE', *, *, #12840, .F. ) ;
#1203=CARTESIAN_POINT ( 'NONE',  ( -30.63887302793240508, 5.335677986745117174, -6.500000000000000000 ) ) ;
#1204=ORIENTED_EDGE ( 'NONE', *, *, #21065, .F. ) ;
#1206=EDGE_CURVE ( 'NONE', #10563, #17279, #13544, .T. ) ;
#1207=EDGE_LOOP ( 'NONE', ( #8391, #20008, #11792, #25836 ) ) ;
#1211=VECTOR ( 'NONE', #750, 1000.000000000000000 ) ;
#1212=ORIENTED_EDGE ( 'NONE', *, *, #17247, .T. ) ;
#1213=FACE_OUTER_BOUND ( 'NONE', #5482, .T. ) ;
#1215=EDGE_CURVE ( 'NONE', #17650, #15811, #15635, .T. ) ;
#1220=DIRECTION ( 'NONE',  ( 0.000000000000000000, -0.000000000000000000, 1.000000000000000000 ) ) ;
#1222=DIRECTION ( 'NONE',  ( 0.000000000000000000, 0.000000000000000000, 1.000000000000000000 ) ) ;
#1226=AXIS2_PLACEMENT_3D ( 'NONE', #21445, #15428, #23533 ) ;
#1227=ORIENTED_EDGE ( 'NONE', *, *, #15608, .T. ) ;
#1230=AXIS2_PLACEMENT_3D ( 'NONE', #16542, #15612, #7365 ) ;
#1231=DIRECTION ( 'NONE',  ( 1.000000000000000000, 0.000000000000000000, 0.000000000000000000 ) ) ;
#1232=AXIS2_PLACEMENT_3D ( 'NONE', #10906, #22821, #1231 ) ;
#1236=EDGE_LOOP ( 'NONE', ( #16558, #5111, #1058, #21230 ) ) ;
#1237=CARTESIAN_POINT ( 'NONE',  ( -3.397863563850083146, -30.85476721088024021, 1.000000000000000000 ) ) ;
#1239=CARTESIAN_POINT ( 'NONE',  ( 0.000000000000000000, 0.000000000000000000, 1.000000000000000000 ) ) ;
#1243=CARTESIAN_POINT ( 'NONE',  ( -27.25313774936397948, 14.98253926456367502, -6.500000000000000000 ) ) ;
#1246=VECTOR ( 'NONE', #15657, 1000.000000000000000 ) ;
#1250=EDGE_CURVE ( 'NONE', #6185, #21954, #25154, .T. ) ;
#1251=DIRECTION ( 'NONE',  ( -0.000000000000000000, 0.000000000000000000, 1.000000000000000000 ) ) ;
#1253=CARTESIAN_POINT ( 'NONE',  ( -9.610428525061097460, -29.57785765677920509, 1.000000000000000000 ) ) ;
#1254=DIRECTION ( 'NONE',  ( 1.000000000000000000, 0.000000000000000000, 0.000000000000000000 ) ) ;
#1256=CIRCLE ( 'NONE', #21720, 0.5000000000000002220 ) ;
#1260=CARTESIAN_POINT ( 'NONE',  ( 31.06601413805602263, -1.453535542772716793, -2.750000000000000000 ) ) ;
#1262=CIRCLE ( 'NONE', #5428, 0.5000000000000003331 ) ;
#1264=AXIS2_PLACEMENT_3D ( 'NONE', #25584, #5697, #1523 ) ;
#1267=ORIENTED_EDGE ( 'NONE', *, *, #17537, .T. ) ;
#1271=DIRECTION ( 'NONE',  ( 0.000000000000000000, 0.000000000000000000, 1.000000000000000000 ) ) ;
#1272=ORIENTED_EDGE ( 'NONE', *, *, #18531, .T. ) ;
#1281=CIRCLE ( 'NONE', #10881, 0.5000000000000002220 ) ;
#1282=ADVANCED_FACE ( 'NONE', ( #25814 ), #7386, .T. ) ;
#1286=DIRECTION ( 'NONE',  ( 0.000000000000000000, 0.000000000000000000, 1.000000000000000000 ) ) ;
#1289=AXIS2_PLACEMENT_3D ( 'NONE', #7040, #4829, #16993 ) ;
#1295=CARTESIAN_POINT ( 'NONE',  ( 9.610428525060671134, -29.57785765677934009, -6.500000000000000000 ) ) ;
#1304=CARTESIAN_POINT ( 'NONE',  ( -29.41953157733080104, 10.08469938919530584, -2.750000000000000000 ) ) ;
#1307=FACE_OUTER_BOUND ( 'NONE', #12729, .T. ) ;
#1309=VERTEX_POINT ( 'NONE', #5680 ) ;
#1311=EDGE_LOOP ( 'NONE', ( #346, #6595, #13086, #8643 ) ) ;
#1314=EDGE_CURVE ( 'NONE', #16500, #21799, #19529, .T. ) ;
#1315=VERTEX_POINT ( 'NONE', #13659 ) ;
#1317=CIRCLE ( 'NONE', #12586, 0.4999999999999993894 ) ;
#1319=EDGE_CURVE ( 'NONE', #14821, #23630, #19800, .T. ) ;
#1329=CIRCLE ( 'NONE', #21778, 0.5000000000000003331 ) ;
#1330=FACE_OUTER_BOUND ( 'NONE', #4234, .T. ) ;
#1335=DIRECTION ( 'NONE',  ( -0.000000000000000000, -0.000000000000000000, 1.000000000000000000 ) ) ;
#1336=ADVANCED_FACE ( 'NONE', ( #1988 ), #4458, .F. ) ;
#1339=AXIS2_PLACEMENT_3D ( 'NONE', #7048, #20294, #10224 ) ;
#1343=VERTEX_POINT ( 'NONE', #15994 ) ;
#1344=CARTESIAN_POINT ( 'NONE',  ( 16.66421332384682685, 26.25859848311265310, -6.500000000000000000 ) ) ;
#1345=VERTEX_POINT ( 'NONE', #15853 ) ;
#1346=ORIENTED_EDGE ( 'NONE', *, *, #22021, .T. ) ;
#1347=FACE_OUTER_BOUND ( 'NONE', #5617, .T. ) ;
#1354=ORIENTED_EDGE ( 'NONE', *, *, #17162, .T. ) ;
#1355=AXIS2_PLACEMENT_3D ( 'NONE', #6744, #12886, #22834 ) ;
#1361=CARTESIAN_POINT ( 'NONE',  ( -22.17092431280609333, -21.28941499438201745, 1.000000000000000000 ) ) ;
#1364=AXIS2_PLACEMENT_3D ( 'NONE', #21070, #13486, #3400 ) ;
#1369=DIRECTION ( 'NONE',  ( 1.000000000000000000, 0.000000000000000000, 0.000000000000000000 ) ) ;
#1370=ORIENTED_EDGE ( 'NONE', *, *, #24143, .T. ) ;
#1375=DIRECTION ( 'NONE',  ( 0.000000000000000000, 0.000000000000000000, 1.000000000000000000 ) ) ;
#1379=ORIENTED_EDGE ( 'NONE', *, *, #17227, .F. ) ;
#1380=DIRECTION ( 'NONE',  ( 0.000000000000000000, 0.000000000000000000, 1.000000000000000000 ) ) ;
#1387=VECTOR ( 'NONE', #11364, 1000.000000000000000 ) ;
#1388=DIRECTION ( 'NONE',  ( -0.000000000000000000, -0.000000000000000000, 1.000000000000000000 ) ) ;
#1390=CIRCLE ( 'NONE', #16014, 31.10000000000000142 ) ;
#1391=EDGE_CURVE ( 'NONE', #132, #18031, #4665, .T. ) ;
#1393=CARTESIAN_POINT ( 'NONE',  ( 1.453535542772391942, -31.06601413805603329, -2.750000000000000000 ) ) ;
#1401=CARTESIAN_POINT ( 'NONE',  ( -27.49048467073869517, -14.54246377227329212, -2.750000000000000000 ) ) ;
#1413=ADVANCED_FACE ( 'NONE', ( #20019 ), #14291, .F. ) ;
#1421=DIRECTION ( 'NONE',  ( 1.000000000000000000, 0.000000000000000000, 0.000000000000000000 ) ) ;
#1428=DIRECTION ( 'NONE',  ( 0.9297764858882561212, 0.3681245526846659843, 0.000000000000000000 ) ) ;
#1429=DIRECTION ( 'NONE',  ( -0.000000000000000000, -0.000000000000000000, 1.000000000000000000 ) ) ;
#1432=DIRECTION ( 'NONE',  ( -0.8090169943749498938, -0.5877852522924696954, 0.000000000000000000 ) ) ;
#1441=CARTESIAN_POINT ( 'NONE',  ( -23.46296185032681336, 19.82388608118453632, -6.500000000000000000 ) ) ;
#1442=DIRECTION ( 'NONE',  ( -0.000000000000000000, -0.000000000000000000, 1.000000000000000000 ) ) ;
#1444=ADVANCED_FACE ( 'NONE', ( #12962 ), #2501, .F. ) ;
#1446=VERTEX_POINT ( 'NONE', #22777 ) ;
#1447=ORIENTED_EDGE ( 'NONE', *, *, #54, .T. ) ;
#1451=CARTESIAN_POINT ( 'NONE',  ( -20.78941499438242246, -22.67092431280570963, -6.500000000000000000 ) ) ;
#1452=FACE_OUTER_BOUND ( 'NONE', #21387, .T. ) ;
#1457=DIRECTION ( 'NONE',  ( 1.000000000000000000, 0.000000000000000000, 0.000000000000000000 ) ) ;
#1461=FACE_OUTER_BOUND ( 'NONE', #21531, .T. ) ;
#1467=CARTESIAN_POINT ( 'NONE',  ( 0.000000000000000000, 0.000000000000000000, -6.500000000000000000 ) ) ;
#1470=ORIENTED_EDGE ( 'NONE', *, *, #18126, .F. ) ;
#1473=CARTESIAN_POINT ( 'NONE',  ( 29.57785765677931167, 9.610428525060783045, -6.500000000000000000 ) ) ;
#1474=ORIENTED_EDGE ( 'NONE', *, *, #20091, .T. ) ;
#1476=ORIENTED_EDGE ( 'NONE', *, *, #12495, .F. ) ;
#1479=EDGE_CURVE ( 'NONE', #12855, #15503, #7340, .T. ) ;
#1483=CARTESIAN_POINT ( 'NONE',  ( -19.43607991388954304, 24.27856662945528399, -6.500000000000000000 ) ) ;
#1491=ORIENTED_EDGE ( 'NONE', *, *, #14009, .T. ) ;
#1492=VERTEX_POINT ( 'NONE', #8776 ) ;
#1495=ORIENTED_EDGE ( 'NONE', *, *, #8498, .T. ) ;
#1498=CARTESIAN_POINT ( 'NONE',  ( 1.453535542772518951, -31.06601413805602618, 1.000000000000000000 ) ) ;
#1499=EDGE_LOOP ( 'NONE', ( #15805, #18809, #521, #10617 ) ) ;
#1501=ORIENTED_EDGE ( 'NONE', *, *, #9500, .F. ) ;
#1508=EDGE_CURVE ( 'NONE', #21865, #6673, #1909, .T. ) ;
#1509=VECTOR ( 'NONE', #25750, 1000.000000000000000 ) ;
#1510=CARTESIAN_POINT ( 'NONE',  ( 31.00322564728513086, -2.451530025009243108, -6.500000000000000000 ) ) ;
#1513=CARTESIAN_POINT ( 'NONE',  ( 0.000000000000000000, 0.000000000000000000, 1.000000000000000000 ) ) ;
#1519=CYLINDRICAL_SURFACE ( 'NONE', #14271, 31.10000000000000142 ) ;
#1523=DIRECTION ( 'NONE',  ( 1.000000000000000000, 0.000000000000000000, 0.000000000000000000 ) ) ;
#1524=VERTEX_POINT ( 'NONE', #6549 ) ;
#1539=ADVANCED_FACE ( 'NONE', ( #20678 ), #14668, .T. ) ;
#1540=LINE ( 'NONE', #25464, #24379 ) ;
#1541=EDGE_CURVE ( 'NONE', #17200, #10079, #20708, .T. ) ;
#1543=( LENGTH_UNIT ( ) NAMED_UNIT ( * ) SI_UNIT ( .MILLI., .METRE. ) );
#1544=DIRECTION ( 'NONE',  ( 0.000000000000000000, 0.000000000000000000, 1.000000000000000000 ) ) ;
#1547=CARTESIAN_POINT ( 'NONE',  ( -28.34936733434208733, -12.78762572734038727, 1.000000000000000000 ) ) ;
#1548=CYLINDRICAL_SURFACE ( 'NONE', #6201, 31.10000000000000142 ) ;
#1551=ORIENTED_EDGE ( 'NONE', *, *, #2804, .T. ) ;
#1553=CARTESIAN_POINT ( 'NONE',  ( 9.133673601486252736, -29.72853858738288935, -2.750000000000000000 ) ) ;
#1560=CYLINDRICAL_SURFACE ( 'NONE', #1671, 31.10000000000000142 ) ;
#1561=CARTESIAN_POINT ( 'NONE',  ( 10.08469938919487419, 29.41953157733095026, 1.000000000000000000 ) ) ;
#1562=ORIENTED_EDGE ( 'NONE', *, *, #23060, .F. ) ;
#1563=ORIENTED_EDGE ( 'NONE', *, *, #22830, .F. ) ;
#1565=ORIENTED_EDGE ( 'NONE', *, *, #10538, .F. ) ;
#1566=ORIENTED_EDGE ( 'NONE', *, *, #6970, .T. ) ;
#1567=EDGE_CURVE ( 'NONE', #21040, #583, #8647, .T. ) ;
#1568=CARTESIAN_POINT ( 'NONE',  ( 0.000000000000000000, 0.000000000000000000, 1.000000000000000000 ) ) ;
#1569=CYLINDRICAL_SURFACE ( 'NONE', #24050, 31.10000000000000142 ) ;
#1570=EDGE_CURVE ( 'NONE', #23781, #19322, #259, .T. ) ;
#1575=EDGE_CURVE ( 'NONE', #17398, #7608, #650, .T. ) ;
#1577=CARTESIAN_POINT ( 'NONE',  ( -25.45105997952938637, -17.87326343783915306, -6.500000000000000000 ) ) ;
#1580=DIRECTION ( 'NONE',  ( 0.9685831611286337406, 0.2486898871648445808, 0.000000000000000000 ) ) ;
#1581=CARTESIAN_POINT ( 'NONE',  ( -23.46296185032681336, 19.82388608118453632, -6.500000000000000000 ) ) ;
#1582=DIRECTION ( 'NONE',  ( 1.000000000000000000, 0.000000000000000000, 0.000000000000000000 ) ) ;
#1586=DIRECTION ( 'NONE',  ( -0.5358267949789882190, 0.8443279255020205154, 0.000000000000000000 ) ) ;
#1587=VECTOR ( 'NONE', #14038, 1000.000000000000000 ) ;
#1588=DIRECTION ( 'NONE',  ( 0.000000000000000000, 0.000000000000000000, 1.000000000000000000 ) ) ;
#1590=VERTEX_POINT ( 'NONE', #18171 ) ;
#1592=ORIENTED_EDGE ( 'NONE', *, *, #22431, .T. ) ;
#1595=CARTESIAN_POINT ( 'NONE',  ( 11.44867358849329619, -28.91604871112469510, -6.500000000000000000 ) ) ;
#1596=CIRCLE ( 'NONE', #343, 0.5000000000000002220 ) ;
#1601=DIRECTION ( 'NONE',  ( 0.000000000000000000, 0.000000000000000000, 1.000000000000000000 ) ) ;
#1609=AXIS2_PLACEMENT_3D ( 'NONE', #14552, #22398, #2146 ) ;
#1615=EDGE_LOOP ( 'NONE', ( #1947, #4726, #1491, #22145 ) ) ;
#1622=DIRECTION ( 'NONE',  ( 1.000000000000000000, 0.000000000000000000, 0.000000000000000000 ) ) ;
#1624=ORIENTED_EDGE ( 'NONE', *, *, #20661, .F. ) ;
#1626=CIRCLE ( 'NONE', #4553, 31.10000000000000142 ) ;
#1627=VERTEX_POINT ( 'NONE', #252 ) ;
#1628=EDGE_CURVE ( 'NONE', #22817, #8694, #10042, .T. ) ;
#1632=CARTESIAN_POINT ( 'NONE',  ( 25.16042852506090810, 18.28012134629586072, 1.000000000000000000 ) ) ;
#1634=EDGE_CURVE ( 'NONE', #16116, #24580, #512, .T. ) ;
#1639=CIRCLE ( 'NONE', #19592, 31.10000000000000142 ) ;
#1642=AXIS2_PLACEMENT_3D ( 'NONE', #24457, #22361, #22882 ) ;
#1646=EDGE_CURVE ( 'NONE', #3229, #12524, #24873, .T. ) ;
#1647=DIRECTION ( 'NONE',  ( 1.000000000000000000, 0.000000000000000000, 0.000000000000000000 ) ) ;
#1650=DIRECTION ( 'NONE',  ( 1.000000000000000000, 0.000000000000000000, 0.000000000000000000 ) ) ;
#1651=VECTOR ( 'NONE', #15719, 1000.000000000000000 ) ;
#1656=CARTESIAN_POINT ( 'NONE',  ( 0.000000000000000000, 0.000000000000000000, -6.500000000000000000 ) ) ;
#1659=CIRCLE ( 'NONE', #10826, 31.10000000000000142 ) ;
#1660=ADVANCED_FACE ( 'NONE', ( #10583 ), #20663, .F. ) ;
#1662=AXIS2_PLACEMENT_3D ( 'NONE', #11194, #1271, #8727 ) ;
#1663=ORIENTED_EDGE ( 'NONE', *, *, #22246, .F. ) ;
#1664=CARTESIAN_POINT ( 'NONE',  ( -8.217531866531306406, -29.99470236596026851, 1.000000000000000000 ) ) ;
#1666=VERTEX_POINT ( 'NONE', #16745 ) ;
#1669=AXIS2_PLACEMENT_3D ( 'NONE', #5031, #11432, #22947 ) ;
#1671=AXIS2_PLACEMENT_3D ( 'NONE', #23266, #1166, #21180 ) ;
#1672=DIRECTION ( 'NONE',  ( 1.000000000000000000, 0.000000000000000000, 0.000000000000000000 ) ) ;
#1673=SURFACE_SIDE_STYLE ('',( #11477 ) ) ;
#1674=CARTESIAN_POINT ( 'NONE',  ( 16.23990935651698564, -26.52310962334756184, -6.500000000000000000 ) ) ;
#1678=DIRECTION ( 'NONE',  ( 0.000000000000000000, 0.000000000000000000, 1.000000000000000000 ) ) ;
#1681=CARTESIAN_POINT ( 'NONE',  ( 30.12293631110040693, -7.734255490827107948, 1.000000000000000000 ) ) ;
#1682=EDGE_CURVE ( 'NONE', #8556, #23396, #14649, .T. ) ;
#1683=VERTEX_POINT ( 'NONE', #22237 ) ;
#1684=DIRECTION ( 'NONE',  ( 0.000000000000000000, 0.000000000000000000, 1.000000000000000000 ) ) ;
#1687=CIRCLE ( 'NONE', #2119, 31.10000000000000142 ) ;
#1692=ORIENTED_EDGE ( 'NONE', *, *, #9696, .F. ) ;
#1693=DIRECTION ( 'NONE',  ( 0.000000000000000000, 0.000000000000000000, 1.000000000000000000 ) ) ;
#1694=CARTESIAN_POINT ( 'NONE',  ( -23.46296185032722548, -19.82388608118403539, -6.500000000000000000 ) ) ;
#1696=EDGE_LOOP ( 'NONE', ( #4976, #21317, #11139, #14311 ) ) ;
#1697=EDGE_CURVE ( 'NONE', #25550, #4816, #12338, .T. ) ;
#1698=ORIENTED_EDGE ( 'NONE', *, *, #1206, .F. ) ;
#1699=CIRCLE ( 'NONE', #20903, 0.4999999999999992784 ) ;
#1700=ORIENTED_EDGE ( 'NONE', *, *, #14006, .F. ) ;
#1701=VERTEX_POINT ( 'NONE', #24190 ) ;
#1703=DIRECTION ( 'NONE',  ( 1.000000000000000000, 0.000000000000000000, 0.000000000000000000 ) ) ;
#1704=DIRECTION ( 'NONE',  ( -0.000000000000000000, -0.000000000000000000, 1.000000000000000000 ) ) ;
#1705=VECTOR ( 'NONE', #15383, 1000.000000000000000 ) ;
#1706=DIRECTION ( 'NONE',  ( 1.000000000000000000, 0.000000000000000000, 0.000000000000000000 ) ) ;
#1709=VECTOR ( 'NONE', #10698, 1000.000000000000000 ) ;
#1714=DIRECTION ( 'NONE',  ( 1.000000000000000000, 0.000000000000000000, 0.000000000000000000 ) ) ;
#1715=VECTOR ( 'NONE', #7862, 1000.000000000000000 ) ;
#1716=EDGE_CURVE ( 'NONE', #24486, #19788, #12550, .T. ) ;
#1719=DIRECTION ( 'NONE',  ( -0.7705132427757840352, 0.6374239897486960738, 0.000000000000000000 ) ) ;
#1722=AXIS2_PLACEMENT_3D ( 'NONE', #7012, #2971, #10938 ) ;
#1724=EDGE_CURVE ( 'NONE', #364, #9403, #2359, .T. ) ;
#1725=CIRCLE ( 'NONE', #17586, 0.5000000000000001110 ) ;
#1732=AXIS2_PLACEMENT_3D ( 'NONE', #24806, #16316, #18922 ) ;
#1733=ORIENTED_EDGE ( 'NONE', *, *, #2952, .T. ) ;
#1735=ORIENTED_EDGE ( 'NONE', *, *, #14508, .F. ) ;
#1737=ORIENTED_EDGE ( 'NONE', *, *, #16361, .T. ) ;
#1744=DIRECTION ( 'NONE',  ( 0.000000000000000000, 0.000000000000000000, 1.000000000000000000 ) ) ;
#1759=CIRCLE ( 'NONE', #16381, 0.5000000000000002220 ) ;
#1760=ORIENTED_EDGE ( 'NONE', *, *, #15178, .F. ) ;
#1763=ADVANCED_FACE ( 'NONE', ( #402 ), #8371, .F. ) ;
#1765=EDGE_LOOP ( 'NONE', ( #24272, #20790, #5968, #16322 ) ) ;
#1766=CARTESIAN_POINT ( 'NONE',  ( -26.25859848311282363, -16.66421332384654974, -6.500000000000000000 ) ) ;
#1774=CYLINDRICAL_SURFACE ( 'NONE', #5980, 31.10000000000000142 ) ;
#1775=CARTESIAN_POINT ( 'NONE',  ( 0.000000000000000000, 0.000000000000000000, -6.500000000000000000 ) ) ;
#1777=DIRECTION ( 'NONE',  ( 0.000000000000000000, 0.000000000000000000, 1.000000000000000000 ) ) ;
#1779=AXIS2_PLACEMENT_3D ( 'NONE', #11090, #1544, #9511 ) ;
#1780=AXIS2_PLACEMENT_3D ( 'NONE', #1681, #25346, #11485 ) ;
#1781=DIRECTION ( 'NONE',  ( 0.8090169943749474513, -0.5877852522924730261, 0.000000000000000000 ) ) ;
#1782=DIRECTION ( 'NONE',  ( -0.4257792915650642218, 0.9048270524660235736, 0.000000000000000000 ) ) ;
#1783=CARTESIAN_POINT ( 'NONE',  ( 0.000000000000000000, 0.000000000000000000, -6.500000000000000000 ) ) ;
#1784=DIRECTION ( 'NONE',  ( 1.000000000000000000, 0.000000000000000000, 0.000000000000000000 ) ) ;
#1787=CARTESIAN_POINT ( 'NONE',  ( -2.451530025009351910, -31.00322564728512020, -2.750000000000000000 ) ) ;
#1788=DIRECTION ( 'NONE',  ( 1.000000000000000000, 0.000000000000000000, 0.000000000000000000 ) ) ;
#1790=CYLINDRICAL_SURFACE ( 'NONE', #9593, 31.10000000000000142 ) ;
#1791=CARTESIAN_POINT ( 'NONE',  ( 20.20656826142283435, 23.64116323484230975, -6.500000000000000000 ) ) ;
#1795=DIRECTION ( 'NONE',  ( -0.9980267284282718920, -0.06279051952930848890, 0.000000000000000000 ) ) ;
#1796=VERTEX_POINT ( 'NONE', #541 ) ;
#1802=ORIENTED_EDGE ( 'NONE', *, *, #22163, .T. ) ;
#1803=ORIENTED_EDGE ( 'NONE', *, *, #15696, .F. ) ;
#1807=AXIS2_PLACEMENT_3D ( 'NONE', #12216, #16416, #18236 ) ;
#1810=CIRCLE ( 'NONE', #2223, 0.5000000000000007772 ) ;
#1812=( NAMED_UNIT ( * ) PLANE_ANGLE_UNIT ( ) SI_UNIT ( $, .RADIAN. ) );
#1813=CARTESIAN_POINT ( 'NONE',  ( -18.28012134629613783, -25.16042852506070560, 1.000000000000000000 ) ) ;
#1820=ORIENTED_EDGE ( 'NONE', *, *, #932, .T. ) ;
#1822=CARTESIAN_POINT ( 'NONE',  ( 0.000000000000000000, 0.000000000000000000, -6.500000000000000000 ) ) ;
#1824=CARTESIAN_POINT ( 'NONE',  ( -30.91344420362543843, 3.401318489841417048, -2.750000000000000000 ) ) ;
#1827=CARTESIAN_POINT ( 'NONE',  ( 0.000000000000000000, 0.000000000000000000, 1.000000000000000000 ) ) ;
#1830=LINE ( 'NONE', #7575, #21316 ) ;
#1831=DIRECTION ( 'NONE',  ( -0.6374239897486843054, 0.7705132427757935831, 0.000000000000000000 ) ) ;
#1832=ORIENTED_EDGE ( 'NONE', *, *, #6525, .F. ) ;
#1833=AXIS2_PLACEMENT_3D ( 'NONE', #14255, #20249, #2087 ) ;
#1834=ORIENTED_EDGE ( 'NONE', *, *, #13308, .F. ) ;
#1835=EDGE_CURVE ( 'NONE', #3169, #383, #19018, .T. ) ;
#1836=ORIENTED_EDGE ( 'NONE', *, *, #17614, .T. ) ;
#1837=ORIENTED_EDGE ( 'NONE', *, *, #14330, .T. ) ;
#1840=CARTESIAN_POINT ( 'NONE',  ( 30.54913349766223973, 5.827558883615938434, 1.000000000000000000 ) ) ;
#1841=DIRECTION ( 'NONE',  ( 1.000000000000000000, 0.000000000000000000, 0.000000000000000000 ) ) ;
#1842=EDGE_CURVE ( 'NONE', #7738, #14582, #13104, .T. ) ;
#1844=EDGE_CURVE ( 'NONE', #23396, #4202, #5165, .T. ) ;
#1850=DIRECTION ( 'NONE',  ( 1.000000000000000000, 0.000000000000000000, 0.000000000000000000 ) ) ;
#1852=DIRECTION ( 'NONE',  ( 1.000000000000000000, 0.000000000000000000, 0.000000000000000000 ) ) ;
#1854=LINE ( 'NONE', #9815, #15968 ) ;
#1860=ORIENTED_EDGE ( 'NONE', *, *, #20590, .T. ) ;
#1868=ORIENTED_EDGE ( 'NONE', *, *, #2700, .T. ) ;
#1870=EDGE_CURVE ( 'NONE', #14796, #13703, #23548, .T. ) ;
#1871=ORIENTED_EDGE ( 'NONE', *, *, #10098, .F. ) ;
#1873=DIRECTION ( 'NONE',  ( 0.000000000000000000, 0.000000000000000000, 1.000000000000000000 ) ) ;
#1876=CARTESIAN_POINT ( 'NONE',  ( -30.12293631110050995, -7.734255490826679846, -6.500000000000000000 ) ) ;
#1878=DIRECTION ( 'NONE',  ( 0.000000000000000000, 0.000000000000000000, 1.000000000000000000 ) ) ;
#1884=DIRECTION ( 'NONE',  ( 0.000000000000000000, 0.000000000000000000, 1.000000000000000000 ) ) ;
#1889=DIRECTION ( 'NONE',  ( -0.1253332335643051187, -0.9921147013144777649, 0.000000000000000000 ) ) ;
#1891=CARTESIAN_POINT ( 'NONE',  ( 0.000000000000000000, 0.000000000000000000, -6.500000000000000000 ) ) ;
#1892=FACE_OUTER_BOUND ( 'NONE', #19692, .T. ) ;
#1896=EDGE_LOOP ( 'NONE', ( #5864, #2010, #1837, #5903 ) ) ;
#1897=FACE_OUTER_BOUND ( 'NONE', #3841, .T. ) ;
#1898=EDGE_CURVE ( 'NONE', #6457, #14723, #11710, .T. ) ;
#1908=CYLINDRICAL_SURFACE ( 'NONE', #70, 31.10000000000000142 ) ;
#1909=CIRCLE ( 'NONE', #25701, 31.10000000000000142 ) ;
#1920=CARTESIAN_POINT ( 'NONE',  ( 8.217531866530997320, -29.99470236596036088, 1.000000000000000000 ) ) ;
#1921=ORIENTED_EDGE ( 'NONE', *, *, #17399, .T. ) ;
#1936=LINE ( 'NONE', #24027, #12005 ) ;
#1939=FACE_OUTER_BOUND ( 'NONE', #16075, .T. ) ;
#1946=DIRECTION ( 'NONE',  ( 1.000000000000000000, 0.000000000000000000, 0.000000000000000000 ) ) ;
#1947=ORIENTED_EDGE ( 'NONE', *, *, #3452, .F. ) ;
#1951=VERTEX_POINT ( 'NONE', #5960 ) ;
#1954=ORIENTED_EDGE ( 'NONE', *, *, #4739, .T. ) ;
#1955=LINE ( 'NONE', #10052, #15962 ) ;
#1957=DIRECTION ( 'NONE',  ( 0.6845471059286901694, -0.7289686274214101092, 0.000000000000000000 ) ) ;
#1968=DIRECTION ( 'NONE',  ( 0.000000000000000000, -0.000000000000000000, 1.000000000000000000 ) ) ;
#1975=DIRECTION ( 'NONE',  ( 1.000000000000000000, 0.000000000000000000, 0.000000000000000000 ) ) ;
#1981=ORIENTED_EDGE ( 'NONE', *, *, #20383, .F. ) ;
#1982=DIRECTION ( 'NONE',  ( 0.000000000000000000, 0.000000000000000000, 1.000000000000000000 ) ) ;
#1988=FACE_OUTER_BOUND ( 'NONE', #18323, .T. ) ;
#1993=DIRECTION ( 'NONE',  ( 1.000000000000000000, 0.000000000000000000, 0.000000000000000000 ) ) ;
#1997=CARTESIAN_POINT ( 'NONE',  ( 24.86329371854774806, 18.68225429291723216, -6.500000000000000000 ) ) ;
#1998=DIRECTION ( 'NONE',  ( -0.000000000000000000, -0.000000000000000000, 1.000000000000000000 ) ) ;
#2000=ORIENTED_EDGE ( 'NONE', *, *, #11892, .F. ) ;
#2002=VERTEX_POINT ( 'NONE', #10132 ) ;
#2005=ORIENTED_EDGE ( 'NONE', *, *, #107, .F. ) ;
#2006=DIRECTION ( 'NONE',  ( 0.000000000000000000, 0.000000000000000000, 1.000000000000000000 ) ) ;
#2010=ORIENTED_EDGE ( 'NONE', *, *, #20661, .T. ) ;
#2012=EDGE_CURVE ( 'NONE', #11918, #25564, #21586, .T. ) ;
#2014=DIRECTION ( 'NONE',  ( -0.9297764858882481276, 0.3681245526846864125, 0.000000000000000000 ) ) ;
#2019=CIRCLE ( 'NONE', #6193, 31.10000000000000142 ) ;
#2020=DIRECTION ( 'NONE',  ( 1.000000000000000000, 0.000000000000000000, 0.000000000000000000 ) ) ;
#2021=FACE_OUTER_BOUND ( 'NONE', #9736, .T. ) ;
#2026=AXIS2_PLACEMENT_3D ( 'NONE', #14786, #18694, #781 ) ;
#2027=AXIS2_PLACEMENT_3D ( 'NONE', #6618, #6887, #2580 ) ;
#2031=DIRECTION ( 'NONE',  ( -0.000000000000000000, 0.000000000000000000, -1.000000000000000000 ) ) ;
#2033=CIRCLE ( 'NONE', #10360, 0.5000000000000003331 ) ;
#2038=ORIENTED_EDGE ( 'NONE', *, *, #14019, .F. ) ;
#2045=CARTESIAN_POINT ( 'NONE',  ( 31.03863125411924173, -1.952785157361756951, 1.000000000000000000 ) ) ;
#2048=VERTEX_POINT ( 'NONE', #16429 ) ;
#2049=DIRECTION ( 'NONE',  ( -0.7289686274214168815, -0.6845471059286831750, 0.000000000000000000 ) ) ;
#2054=AXIS2_PLACEMENT_3D ( 'NONE', #23317, #25026, #25407 ) ;
#2056=AXIS2_PLACEMENT_3D ( 'NONE', #10382, #612, #6602 ) ;
#2067=DIRECTION ( 'NONE',  ( 0.000000000000000000, -0.000000000000000000, 1.000000000000000000 ) ) ;
#2073=ORIENTED_EDGE ( 'NONE', *, *, #8131, .F. ) ;
#2077=CARTESIAN_POINT ( 'NONE',  ( 0.000000000000000000, 0.000000000000000000, -6.500000000000000000 ) ) ;
#2078=VERTEX_POINT ( 'NONE', #2171 ) ;
#2079=AXIS2_PLACEMENT_3D ( 'NONE', #5171, #16819, #2941 ) ;
#2080=ORIENTED_EDGE ( 'NONE', *, *, #18735, .T. ) ;
#2081=ORIENTED_EDGE ( 'NONE', *, *, #7267, .T. ) ;
#2083=VERTEX_POINT ( 'NONE', #16289 ) ;
#2085=CARTESIAN_POINT ( 'NONE',  ( -20.92219106202026069, 23.01025686871660980, 1.000000000000000000 ) ) ;
#2086=CIRCLE ( 'NONE', #4169, 0.5000000000000005551 ) ;
#2087=DIRECTION ( 'NONE',  ( 1.000000000000000000, 0.000000000000000000, 0.000000000000000000 ) ) ;
#2090=CIRCLE ( 'NONE', #3756, 0.4999999999999998890 ) ;
#2096=DIRECTION ( 'NONE',  ( 1.000000000000000000, 0.000000000000000000, 0.000000000000000000 ) ) ;
#2098=CYLINDRICAL_SURFACE ( 'NONE', #17997, 0.5000000000000004441 ) ;
#2100=CARTESIAN_POINT ( 'NONE',  ( 0.000000000000000000, 0.000000000000000000, 1.000000000000000000 ) ) ;
#2103=DIRECTION ( 'NONE',  ( -0.06279051952930156388, 0.9980267284282724471, 0.000000000000000000 ) ) ;
#2106=DIRECTION ( 'NONE',  ( -0.000000000000000000, 0.000000000000000000, 1.000000000000000000 ) ) ;
#2111=AXIS2_PLACEMENT_3D ( 'NONE', #16330, #4155, #8480 ) ;
#2112=ADVANCED_FACE ( 'NONE', ( #10641 ), #21477, .T. ) ;
#2113=EDGE_LOOP ( 'NONE', ( #13094, #10552, #24464, #2081 ) ) ;
#2115=ORIENTED_EDGE ( 'NONE', *, *, #25617, .F. ) ;
#2119=AXIS2_PLACEMENT_3D ( 'NONE', #7456, #13612, #1457 ) ;
#2120=EDGE_CURVE ( 'NONE', #8878, #5837, #20859, .T. ) ;
#2121=EDGE_LOOP ( 'NONE', ( #9027, #1692, #19353, #14919 ) ) ;
#2123=CARTESIAN_POINT ( 'NONE',  ( -25.16042852506104666, -18.28012134629567598, -6.500000000000000000 ) ) ;
#2125=DIRECTION ( 'NONE',  ( -0.3681245526846803617, -0.9297764858882504591, 0.000000000000000000 ) ) ;
#2129=VECTOR ( 'NONE', #20230, 1000.000000000000000 ) ;
#2131=CIRCLE ( 'NONE', #16756, 31.10000000000000142 ) ;
#2136=AXIS2_PLACEMENT_3D ( 'NONE', #11970, #15915, #24406 ) ;
#2144=CIRCLE ( 'NONE', #20503, 0.5000000000000007772 ) ;
#2146=DIRECTION ( 'NONE',  ( 1.000000000000000000, 0.000000000000000000, 0.000000000000000000 ) ) ;
#2151=CIRCLE ( 'NONE', #16363, 30.10000000000000142 ) ;
#2154=DIRECTION ( 'NONE',  ( 0.000000000000000000, -0.000000000000000000, 1.000000000000000000 ) ) ;
#2156=DIRECTION ( 'NONE',  ( 0.9297764858882561212, 0.3681245526846659843, 0.000000000000000000 ) ) ;
#2157=AXIS2_PLACEMENT_3D ( 'NONE', #21135, #23345, #11317 ) ;
#2160=EDGE_CURVE ( 'NONE', #3679, #5799, #13370, .T. ) ;
#2161=EDGE_CURVE ( 'NONE', #17006, #8351, #10005, .T. ) ;
#2165=CIRCLE ( 'NONE', #18881, 31.10000000000000142 ) ;
#2166=CARTESIAN_POINT ( 'NONE',  ( 25.16042852506077665, -18.28012134629603835, -6.500000000000000000 ) ) ;
#2167=DIRECTION ( 'NONE',  ( 0.000000000000000000, 0.000000000000000000, 1.000000000000000000 ) ) ;
#2169=DIRECTION ( 'NONE',  ( -0.000000000000000000, -0.000000000000000000, 1.000000000000000000 ) ) ;
#2170=CARTESIAN_POINT ( 'NONE',  ( -15.41874213889376044, 27.00874656207322388, 1.000000000000000000 ) ) ;
#2171=CARTESIAN_POINT ( 'NONE',  ( -30.63887302793251521, -5.335677986744475021, -6.500000000000000000 ) ) ;
#2172=VECTOR ( 'NONE', #16285, 1000.000000000000000 ) ;
#2173=DIRECTION ( 'NONE',  ( -0.000000000000000000, -0.000000000000000000, 1.000000000000000000 ) ) ;
#2179=ORIENTED_EDGE ( 'NONE', *, *, #17336, .F. ) ;
#2181=DIRECTION ( 'NONE',  ( -0.000000000000000000, -0.000000000000000000, 1.000000000000000000 ) ) ;
#2182=DIRECTION ( 'NONE',  ( 0.000000000000000000, 0.000000000000000000, 1.000000000000000000 ) ) ;
#2183=ORIENTED_EDGE ( 'NONE', *, *, #9367, .F. ) ;
#2184=ORIENTED_EDGE ( 'NONE', *, *, #24522, .F. ) ;
#2186=VECTOR ( 'NONE', #23671, 1000.000000000000000 ) ;
#2190=ADVANCED_FACE ( 'NONE', ( #18636 ), #22697, .F. ) ;
#2192=VECTOR ( 'NONE', #21248, 1000.000000000000000 ) ;
#2198=AXIS2_PLACEMENT_3D ( 'NONE', #18811, #10567, #899 ) ;
#2199=CARTESIAN_POINT ( 'NONE',  ( -19.32388608118395013, 23.96296185032730364, -6.500000000000000000 ) ) ;
#2201=CARTESIAN_POINT ( 'NONE',  ( -5.335677986744340906, 30.63887302793254364, -2.750000000000000000 ) ) ;
#2204=EDGE_CURVE ( 'NONE', #2274, #9390, #19188, .T. ) ;
#2205=ORIENTED_EDGE ( 'NONE', *, *, #4303, .F. ) ;
#2211=CARTESIAN_POINT ( 'NONE',  ( -2.451530025009224456, -31.00322564728513086, 1.000000000000000000 ) ) ;
#2214=CARTESIAN_POINT ( 'NONE',  ( 0.000000000000000000, 0.000000000000000000, -6.500000000000000000 ) ) ;
#2220=VERTEX_POINT ( 'NONE', #21343 ) ;
#2222=DIRECTION ( 'NONE',  ( 1.000000000000000000, 0.000000000000000000, 0.000000000000000000 ) ) ;
#2223=AXIS2_PLACEMENT_3D ( 'NONE', #18502, #16537, #24500 ) ;
#2230=EDGE_CURVE ( 'NONE', #19514, #17747, #25386, .T. ) ;
#2231=LINE ( 'NONE', #16354, #4218 ) ;
#2232=DIRECTION ( 'NONE',  ( 0.000000000000000000, 0.000000000000000000, 1.000000000000000000 ) ) ;
#2235=CARTESIAN_POINT ( 'NONE',  ( -30.12293631110050995, -7.734255490826679846, -6.500000000000000000 ) ) ;
#2240=CARTESIAN_POINT ( 'NONE',  ( 0.000000000000000000, 0.000000000000000000, -6.500000000000000000 ) ) ;
#2244=VERTEX_POINT ( 'NONE', #15462 ) ;
#2245=CARTESIAN_POINT ( 'NONE',  ( -3.401318489841309578, -30.91344420362545264, -2.750000000000000000 ) ) ;
#2247=ORIENTED_EDGE ( 'NONE', *, *, #7336, .F. ) ;
#2250=ORIENTED_EDGE ( 'NONE', *, *, #3988, .T. ) ;
#2257=CIRCLE ( 'NONE', #16886, 31.10000000000000142 ) ;
#2261=DIRECTION ( 'NONE',  ( 0.3681245526846875782, 0.9297764858882475725, 0.000000000000000000 ) ) ;
#2263=FACE_OUTER_BOUND ( 'NONE', #14410, .T. ) ;
#2265=CARTESIAN_POINT ( 'NONE',  ( -0.4999838450259763700, 31.09598070739550124, -2.750000000000000000 ) ) ;
#2268=EDGE_CURVE ( 'NONE', #7474, #12702, #12622, .T. ) ;
#2272=ORIENTED_EDGE ( 'NONE', *, *, #6192, .F. ) ;
#2274=VERTEX_POINT ( 'NONE', #7473 ) ;
#2275=CARTESIAN_POINT ( 'NONE',  ( -30.54913349766228592, -5.827558883615738594, 1.000000000000000000 ) ) ;
#2279=ORIENTED_EDGE ( 'NONE', *, *, #13815, .F. ) ;
#2286=CARTESIAN_POINT ( 'NONE',  ( 29.09636799667075024, -10.98232076577232519, -6.500000000000000000 ) ) ;
#2287=CYLINDRICAL_SURFACE ( 'NONE', #22537, 31.10000000000000142 ) ;
#2289=DIRECTION ( 'NONE',  ( 0.000000000000000000, 0.000000000000000000, 1.000000000000000000 ) ) ;
#2293=DIRECTION ( 'NONE',  ( 0.000000000000000000, 0.000000000000000000, 1.000000000000000000 ) ) ;
#2294=EDGE_CURVE ( 'NONE', #2754, #246, #2086, .T. ) ;
#2302=EDGE_CURVE ( 'NONE', #2607, #25564, #21701, .T. ) ;
#2306=LINE ( 'NONE', #10528, #24599 ) ;
#2310=ORIENTED_EDGE ( 'NONE', *, *, #17345, .T. ) ;
#2314=CARTESIAN_POINT ( 'NONE',  ( -31.09598070739550835, -0.4999838450256507416, -2.750000000000000000 ) ) ;
#2316=CARTESIAN_POINT ( 'NONE',  ( 0.000000000000000000, 0.000000000000000000, 1.000000000000000000 ) ) ;
#2319=CARTESIAN_POINT ( 'NONE',  ( 25.98730014090442353, 17.08421000182768523, -2.750000000000000000 ) ) ;
#2321=DIRECTION ( 'NONE',  ( 0.000000000000000000, -0.000000000000000000, 1.000000000000000000 ) ) ;
#2325=DIRECTION ( 'NONE',  ( 0.000000000000000000, -0.000000000000000000, 1.000000000000000000 ) ) ;
#2326=DIRECTION ( 'NONE',  ( 1.000000000000000000, 0.000000000000000000, 0.000000000000000000 ) ) ;
#2333=CYLINDRICAL_SURFACE ( 'NONE', #9264, 0.5000000000000004441 ) ;
#2337=CARTESIAN_POINT ( 'NONE',  ( -28.72825533807120024, 11.91206721063071505, 1.000000000000000000 ) ) ;
#2339=EDGE_CURVE ( 'NONE', #3260, #21795, #3942, .T. ) ;
#2340=EDGE_LOOP ( 'NONE', ( #22044, #21766, #23462, #9916 ) ) ;
#2341=ORIENTED_EDGE ( 'NONE', *, *, #17195, .T. ) ;
#2343=ORIENTED_EDGE ( 'NONE', *, *, #9994, .F. ) ;
#2357=CARTESIAN_POINT ( 'NONE',  ( -22.32573188046936252, -21.65113613650319380, -6.500000000000000000 ) ) ;
#2359=LINE ( 'NONE', #20530, #3564 ) ;
#2364=CARTESIAN_POINT ( 'NONE',  ( -20.92219106202066925, -23.01025686871623321, -2.750000000000000000 ) ) ;
#2365=LINE ( 'NONE', #18198, #23752 ) ;
#2367=EDGE_CURVE ( 'NONE', #6766, #2636, #12028, .T. ) ;
#2368=ADVANCED_FACE ( 'NONE', ( #5645 ), #13625, .F. ) ;
#2371=ORIENTED_EDGE ( 'NONE', *, *, #8349, .T. ) ;
#2373=ORIENTED_EDGE ( 'NONE', *, *, #8900, .F. ) ;
#2374=DIRECTION ( 'NONE',  ( 1.000000000000000000, 0.000000000000000000, 0.000000000000000000 ) ) ;
#2385=DIRECTION ( 'NONE',  ( 0.000000000000000000, -0.000000000000000000, 1.000000000000000000 ) ) ;
#2386=CARTESIAN_POINT ( 'NONE',  ( -20.92219106202066925, -23.01025686871623321, -6.500000000000000000 ) ) ;
#2388=CARTESIAN_POINT ( 'NONE',  ( -27.49048467073837898, 14.54246377227389075, 1.000000000000000000 ) ) ;
#2397=ORIENTED_EDGE ( 'NONE', *, *, #1567, .T. ) ;
#2398=ORIENTED_EDGE ( 'NONE', *, *, #13996, .F. ) ;
#2406=EDGE_CURVE ( 'NONE', #13215, #25296, #17525, .T. ) ;
#2409=DIRECTION ( 'NONE',  ( -0.6374239897486843054, 0.7705132427757935831, 0.000000000000000000 ) ) ;
#2412=AXIS2_PLACEMENT_3D ( 'NONE', #12844, #7087, #15076 ) ;
#2413=DIRECTION ( 'NONE',  ( 1.000000000000000000, 0.000000000000000000, 0.000000000000000000 ) ) ;
#2420=DIRECTION ( 'NONE',  ( 0.000000000000000000, -0.000000000000000000, 1.000000000000000000 ) ) ;
#2424=AXIS2_PLACEMENT_3D ( 'NONE', #18763, #854, #12630 ) ;
#2429=CARTESIAN_POINT ( 'NONE',  ( 0.000000000000000000, 0.000000000000000000, -6.500000000000000000 ) ) ;
#2433=CIRCLE ( 'NONE', #22489, 31.10000000000000142 ) ;
#2434=DIRECTION ( 'NONE',  ( 0.000000000000000000, 0.000000000000000000, 1.000000000000000000 ) ) ;
#2436=EDGE_CURVE ( 'NONE', #10602, #22990, #928, .T. ) ;
#2438=CIRCLE ( 'NONE', #15040, 31.10000000000000142 ) ;
#2439=CYLINDRICAL_SURFACE ( 'NONE', #24268, 31.10000000000000142 ) ;
#2441=AXIS2_PLACEMENT_3D ( 'NONE', #4566, #24569, #2741 ) ;
#2442=DIRECTION ( 'NONE',  ( 1.000000000000000000, 0.000000000000000000, 0.000000000000000000 ) ) ;
#2451=CARTESIAN_POINT ( 'NONE',  ( -7.248980000274416469, -30.24338421796776544, -6.500000000000000000 ) ) ;
#2457=AXIS2_PLACEMENT_3D ( 'NONE', #17604, #13291, #19546 ) ;
#2460=ORIENTED_EDGE ( 'NONE', *, *, #7737, .F. ) ;
#2461=ORIENTED_EDGE ( 'NONE', *, *, #25604, .T. ) ;
#2462=CARTESIAN_POINT ( 'NONE',  ( -30.04913349766228592, -5.827558883615738594, 1.000000000000000000 ) ) ;
#2465=AXIS2_PLACEMENT_3D ( 'NONE', #20665, #18695, #2869 ) ;
#2471=ADVANCED_FACE ( 'NONE', ( #8377 ), #10321, .F. ) ;
#2472=DIRECTION ( 'NONE',  ( 0.000000000000000000, -0.000000000000000000, 1.000000000000000000 ) ) ;
#2474=CARTESIAN_POINT ( 'NONE',  ( -9.133673601486680838, -29.72853858738275434, 1.000000000000000000 ) ) ;
#2476=DIRECTION ( 'NONE',  ( 0.000000000000000000, 0.000000000000000000, 1.000000000000000000 ) ) ;
#2477=CARTESIAN_POINT ( 'NONE',  ( -9.610428525060479288, 29.57785765677940404, -6.500000000000000000 ) ) ;
#2483=VECTOR ( 'NONE', #15095, 1000.000000000000000 ) ;
#2485=CARTESIAN_POINT ( 'NONE',  ( -30.45149776762733751, -6.317933499823126908, 1.000000000000000000 ) ) ;
#2489=CARTESIAN_POINT ( 'NONE',  ( 27.10000000000000142, 3.318792825689327485E-15, 1.000000000000000000 ) ) ;
#2491=EDGE_LOOP ( 'NONE', ( #11578, #21763, #25653, #7166 ) ) ;
#2492=AXIS2_PLACEMENT_3D ( 'NONE', #24578, #787, #8762 ) ;
#2495=EDGE_LOOP ( 'NONE', ( #10958, #9083, #13510, #24271 ) ) ;
#2497=DIRECTION ( 'NONE',  ( 1.000000000000000000, 0.000000000000000000, 0.000000000000000000 ) ) ;
#2498=CIRCLE ( 'NONE', #17120, 0.4999999999999996669 ) ;
#2499=AXIS2_PLACEMENT_3D ( 'NONE', #2842, #1023, #7022 ) ;
#2501=CYLINDRICAL_SURFACE ( 'NONE', #14849, 0.5000000000000004441 ) ;
#2504=AXIS2_PLACEMENT_3D ( 'NONE', #11262, #1081, #15331 ) ;
#2505=EDGE_CURVE ( 'NONE', #184, #12340, #22364, .T. ) ;
#2507=DIRECTION ( 'NONE',  ( 0.000000000000000000, -0.000000000000000000, -1.000000000000000000 ) ) ;
#2509=CARTESIAN_POINT ( 'NONE',  ( -26.25859848311247902, 16.66421332384710752, -6.500000000000000000 ) ) ;
#2510=EDGE_CURVE ( 'NONE', #6672, #9003, #19601, .T. ) ;
#2511=CARTESIAN_POINT ( 'NONE',  ( -19.82388608118395013, 23.96296185032730364, 1.000000000000000000 ) ) ;
#2514=CARTESIAN_POINT ( 'NONE',  ( -4.393401135981330086, -30.78811501957140351, -2.750000000000000000 ) ) ;
#2515=AXIS2_PLACEMENT_3D ( 'NONE', #13737, #15318, #1852 ) ;
#2522=AXIS2_PLACEMENT_3D ( 'NONE', #16518, #4990, #16632 ) ;
#2523=ADVANCED_FACE ( 'NONE', ( #6808 ), #24722, .T. ) ;
#2524=ORIENTED_EDGE ( 'NONE', *, *, #13156, .F. ) ;
#2526=ORIENTED_EDGE ( 'NONE', *, *, #4172, .F. ) ;
#2529=DIRECTION ( 'NONE',  ( 0.000000000000000000, 0.000000000000000000, 1.000000000000000000 ) ) ;
#2530=DIRECTION ( 'NONE',  ( 1.000000000000000000, 0.000000000000000000, 0.000000000000000000 ) ) ;
#2531=AXIS2_PLACEMENT_3D ( 'NONE', #17826, #12196, #9725 ) ;
#2537=DIRECTION ( 'NONE',  ( 0.000000000000000000, 0.000000000000000000, 1.000000000000000000 ) ) ;
#2538=CARTESIAN_POINT ( 'NONE',  ( 21.28941499438225904, 22.67092431280586240, -6.500000000000000000 ) ) ;
#2540=CIRCLE ( 'NONE', #5879, 31.10000000000000142 ) ;
#2549=AXIS2_PLACEMENT_3D ( 'NONE', #19963, #2067, #16069 ) ;
#2553=VERTEX_POINT ( 'NONE', #12420 ) ;
#2558=ORIENTED_EDGE ( 'NONE', *, *, #8063, .T. ) ;
#2559=CARTESIAN_POINT ( 'NONE',  ( 23.64116323484238080, 20.20656826142275264, -6.500000000000000000 ) ) ;
#2563=ORIENTED_EDGE ( 'NONE', *, *, #16767, .F. ) ;
#2564=VERTEX_POINT ( 'NONE', #22638 ) ;
#2568=AXIS2_PLACEMENT_3D ( 'NONE', #15890, #11564, #5947 ) ;
#2570=VECTOR ( 'NONE', #209, 1000.000000000000000 ) ;
#2577=DIRECTION ( 'NONE',  ( 0.000000000000000000, 0.000000000000000000, 1.000000000000000000 ) ) ;
#2578=EDGE_CURVE ( 'NONE', #18387, #14523, #17115, .T. ) ;
#2579=CARTESIAN_POINT ( 'NONE',  ( 25.45105997952912702, -17.87326343783951899, -6.500000000000000000 ) ) ;
#2580=DIRECTION ( 'NONE',  ( -0.7705132427757840352, 0.6374239897486960738, 0.000000000000000000 ) ) ;
#2584=DIRECTION ( 'NONE',  ( 0.000000000000000000, 0.000000000000000000, 1.000000000000000000 ) ) ;
#2588=ORIENTED_EDGE ( 'NONE', *, *, #13785, .F. ) ;
#2593=ORIENTED_EDGE ( 'NONE', *, *, #1215, .T. ) ;
#2595=CARTESIAN_POINT ( 'NONE',  ( -1.452785157361201396, 31.03863125411927371, -6.500000000000000000 ) ) ;
#2598=ORIENTED_EDGE ( 'NONE', *, *, #22688, .T. ) ;
#2600=CIRCLE ( 'NONE', #8027, 31.10000000000000142 ) ;
#2607=VERTEX_POINT ( 'NONE', #16615 ) ;
#2608=DIRECTION ( 'NONE',  ( -0.000000000000000000, -0.000000000000000000, 1.000000000000000000 ) ) ;
#2609=CYLINDRICAL_SURFACE ( 'NONE', #23897, 0.5000000000000004441 ) ;
#2613=LINE ( 'NONE', #12931, #18471 ) ;
#2617=DIRECTION ( 'NONE',  ( 1.000000000000000000, 0.000000000000000000, 0.000000000000000000 ) ) ;
#2624=CARTESIAN_POINT ( 'NONE',  ( -3.397863563849436108, 30.85476721088031482, -6.500000000000000000 ) ) ;
#2626=ORIENTED_EDGE ( 'NONE', *, *, #846, .F. ) ;
#2632=ORIENTED_EDGE ( 'NONE', *, *, #20451, .F. ) ;
#2633=ORIENTED_EDGE ( 'NONE', *, *, #25293, .T. ) ;
#2636=VERTEX_POINT ( 'NONE', #17392 ) ;
#2637=CYLINDRICAL_SURFACE ( 'NONE', #21391, 31.10000000000000142 ) ;
#2638=EDGE_CURVE ( 'NONE', #10597, #19004, #4581, .T. ) ;
#2646=FACE_OUTER_BOUND ( 'NONE', #4165, .T. ) ;
#2650=DIRECTION ( 'NONE',  ( 0.9048270524660262382, 0.4257792915650585042, 0.000000000000000000 ) ) ;
#2656=ORIENTED_EDGE ( 'NONE', *, *, #13667, .T. ) ;
#2657=EDGE_LOOP ( 'NONE', ( #4903, #21039, #15568, #5873 ) ) ;
#2660=CARTESIAN_POINT ( 'NONE',  ( 1.952785157361650370, 31.03863125411924528, 1.000000000000000000 ) ) ;
#2663=FACE_OUTER_BOUND ( 'NONE', #9440, .T. ) ;
#2665=CYLINDRICAL_SURFACE ( 'NONE', #7591, 0.5000000000000004441 ) ;
#2667=VECTOR ( 'NONE', #3651, 1000.000000000000000 ) ;
#2668=DIRECTION ( 'NONE',  ( 1.000000000000000000, 0.000000000000000000, 0.000000000000000000 ) ) ;
#2669=ORIENTED_EDGE ( 'NONE', *, *, #9832, .T. ) ;
#2670=DIRECTION ( 'NONE',  ( 0.000000000000000000, 0.000000000000000000, 1.000000000000000000 ) ) ;
#2672=CYLINDRICAL_SURFACE ( 'NONE', #6392, 0.5000000000000004441 ) ;
#2673=CARTESIAN_POINT ( 'NONE',  ( -31.10000000000000142, 3.257552089140643357E-13, 1.000000000000000000 ) ) ;
#2674=DIRECTION ( 'NONE',  ( 0.000000000000000000, 0.000000000000000000, -1.000000000000000000 ) ) ;
#2678=CARTESIAN_POINT ( 'NONE',  ( 10.98232076577212624, -29.09636799667083196, 1.000000000000000000 ) ) ;
#2681=DIRECTION ( 'NONE',  ( 0.000000000000000000, -0.000000000000000000, -1.000000000000000000 ) ) ;
#2687=FACE_OUTER_BOUND ( 'NONE', #1056, .T. ) ;
#2688=ORIENTED_EDGE ( 'NONE', *, *, #22471, .T. ) ;
#2689=EDGE_CURVE ( 'NONE', #5115, #24168, #16292, .T. ) ;
#2690=VERTEX_POINT ( 'NONE', #12951 ) ;
#2694=ORIENTED_EDGE ( 'NONE', *, *, #6490, .F. ) ;
#2697=ADVANCED_FACE ( 'NONE', ( #1307 ), #1560, .T. ) ;
#2698=DIRECTION ( 'NONE',  ( 0.000000000000000000, 0.000000000000000000, 1.000000000000000000 ) ) ;
#2700=EDGE_CURVE ( 'NONE', #19352, #12340, #24642, .T. ) ;
#2702=FACE_OUTER_BOUND ( 'NONE', #19595, .T. ) ;
#2703=CYLINDRICAL_SURFACE ( 'NONE', #20515, 0.5000000000000004441 ) ;
#2705=CARTESIAN_POINT ( 'NONE',  ( 30.85476721088027929, 3.897863563849760737, -6.500000000000000000 ) ) ;
#2709=DIRECTION ( 'NONE',  ( 1.000000000000000000, 0.000000000000000000, 0.000000000000000000 ) ) ;
#2711=FACE_OUTER_BOUND ( 'NONE', #8416, .T. ) ;
#2712=ORIENTED_EDGE ( 'NONE', *, *, #7114, .T. ) ;
#2715=ORIENTED_EDGE ( 'NONE', *, *, #900, .F. ) ;
#2719=DIRECTION ( 'NONE',  ( 0.000000000000000000, 0.000000000000000000, 1.000000000000000000 ) ) ;
#2721=DIRECTION ( 'NONE',  ( 1.000000000000000000, 0.000000000000000000, 0.000000000000000000 ) ) ;
#2724=ORIENTED_EDGE ( 'NONE', *, *, #7392, .T. ) ;
#2725=ORIENTED_EDGE ( 'NONE', *, *, #7581, .F. ) ;
#2728=EDGE_CURVE ( 'NONE', #16373, #19798, #11228, .T. ) ;
#2729=AXIS2_PLACEMENT_3D ( 'NONE', #24331, #662, #24455 ) ;
#2737=CARTESIAN_POINT ( 'NONE',  ( 5.335677986744693513, -30.63887302793247258, 1.000000000000000000 ) ) ;
#2738=AXIS2_PLACEMENT_3D ( 'NONE', #8286, #16268, #12339 ) ;
#2740=LINE ( 'NONE', #18826, #12558 ) ;
#2741=DIRECTION ( 'NONE',  ( 1.000000000000000000, 0.000000000000000000, 0.000000000000000000 ) ) ;
#2744=CARTESIAN_POINT ( 'NONE',  ( -30.78811501957148167, -4.393401135980793626, -2.750000000000000000 ) ) ;
#2746=FACE_OUTER_BOUND ( 'NONE', #19654, .T. ) ;
#2749=AXIS2_PLACEMENT_3D ( 'NONE', #4983, #24590, #22506 ) ;
#2752=ORIENTED_EDGE ( 'NONE', *, *, #6733, .T. ) ;
#2754=VERTEX_POINT ( 'NONE', #3391 ) ;
#2757=ORIENTED_EDGE ( 'NONE', *, *, #13499, .F. ) ;
#2759=VERTEX_POINT ( 'NONE', #19468 ) ;
#2760=DIRECTION ( 'NONE',  ( 1.000000000000000000, 0.000000000000000000, 0.000000000000000000 ) ) ;
#2762=EDGE_CURVE ( 'NONE', #18175, #2002, #17007, .T. ) ;
#2764=CARTESIAN_POINT ( 'NONE',  ( -1.952785157361201618, 31.03863125411927371, 1.000000000000000000 ) ) ;
#2766=EDGE_CURVE ( 'NONE', #25364, #18910, #3342, .T. ) ;
#2768=CARTESIAN_POINT ( 'NONE',  ( -31.03863125411922752, 1.952785157361987878, -6.500000000000000000 ) ) ;
#2770=DIRECTION ( 'NONE',  ( -0.000000000000000000, -0.000000000000000000, 1.000000000000000000 ) ) ;
#2775=LINE ( 'NONE', #12588, #4943 ) ;
#2777=ORIENTED_EDGE ( 'NONE', *, *, #136, .T. ) ;
#2778=ORIENTED_EDGE ( 'NONE', *, *, #24551, .F. ) ;
#2780=EDGE_CURVE ( 'NONE', #20797, #6542, #17, .T. ) ;
#2781=ORIENTED_EDGE ( 'NONE', *, *, #1250, .T. ) ;
#2782=CARTESIAN_POINT ( 'NONE',  ( 27.49048467073848911, -14.54246377227368647, 1.000000000000000000 ) ) ;
#2787=VERTEX_POINT ( 'NONE', #13479 ) ;
#2788=CYLINDRICAL_SURFACE ( 'NONE', #25222, 30.10000000000000142 ) ;
#2791=LINE ( 'NONE', #6852, #16768 ) ;
#2792=CARTESIAN_POINT ( 'NONE',  ( 28.34936733434200207, 12.78762572734058978, 1.000000000000000000 ) ) ;
#2796=EDGE_CURVE ( 'NONE', #21955, #15596, #7439, .T. ) ;
#2798=EDGE_LOOP ( 'NONE', ( #8102, #892, #24766, #13917 ) ) ;
#2804=EDGE_CURVE ( 'NONE', #7472, #12264, #5614, .T. ) ;
#2812=EDGE_CURVE ( 'NONE', #16116, #24341, #1256, .T. ) ;
#2814=ORIENTED_EDGE ( 'NONE', *, *, #14043, .T. ) ;
#2818=CYLINDRICAL_SURFACE ( 'NONE', #154, 0.5000000000000004441 ) ;
#2820=CARTESIAN_POINT ( 'NONE',  ( -31.10000000000000142, 3.257552089140643357E-13, -6.500000000000000000 ) ) ;
#2825=FACE_OUTER_BOUND ( 'NONE', #23704, .T. ) ;
#2826=AXIS2_PLACEMENT_3D ( 'NONE', #20097, #8083, #10278 ) ;
#2828=CARTESIAN_POINT ( 'NONE',  ( -31.10000000000000142, 3.257552089140643357E-13, 1.000000000000000000 ) ) ;
#2832=DIRECTION ( 'NONE',  ( 0.9048270524660262382, 0.4257792915650585042, 0.000000000000000000 ) ) ;
#2834=CARTESIAN_POINT ( 'NONE',  ( -6.317933499823659815, -30.45149776762723093, -6.500000000000000000 ) ) ;
#2837=CARTESIAN_POINT ( 'NONE',  ( -18.68225429291695860, 24.86329371854795056, -6.500000000000000000 ) ) ;
#2838=VERTEX_POINT ( 'NONE', #21562 ) ;
#2842=CARTESIAN_POINT ( 'NONE',  ( -14.98253926456356666, -27.25313774936403988, 1.000000000000000000 ) ) ;
#2843=ORIENTED_EDGE ( 'NONE', *, *, #22743, .F. ) ;
#2844=CARTESIAN_POINT ( 'NONE',  ( 16.66421332384682685, 26.25859848311265310, 1.000000000000000000 ) ) ;
#2848=VERTEX_POINT ( 'NONE', #11997 ) ;
#2850=DIRECTION ( 'NONE',  ( -0.1253332335642912687, 0.9921147013144795412, 0.000000000000000000 ) ) ;
#2852=CIRCLE ( 'NONE', #20811, 31.10000000000000142 ) ;
#2854=AXIS2_PLACEMENT_3D ( 'NONE', #22092, #6022, #24187 ) ;
#2858=LINE ( 'NONE', #4711, #11722 ) ;
#2859=FACE_OUTER_BOUND ( 'NONE', #16413, .T. ) ;
#2863=DIRECTION ( 'NONE',  ( 0.000000000000000000, 0.000000000000000000, 1.000000000000000000 ) ) ;
#2865=CARTESIAN_POINT ( 'NONE',  ( -11.44867358849371541, -28.91604871112453168, -6.500000000000000000 ) ) ;
#2868=CIRCLE ( 'NONE', #2026, 0.4999999999999989453 ) ;
#2869=DIRECTION ( 'NONE',  ( 1.000000000000000000, 0.000000000000000000, 0.000000000000000000 ) ) ;
#2871=ADVANCED_FACE ( 'NONE', ( #3642 ), #22070, .T. ) ;
#2872=CIRCLE ( 'NONE', #17488, 0.5000000000000000000 ) ;
#2873=ORIENTED_EDGE ( 'NONE', *, *, #20339, .F. ) ;
#2875=DIRECTION ( 'NONE',  ( 1.000000000000000000, 0.000000000000000000, 0.000000000000000000 ) ) ;
#2877=AXIS2_PLACEMENT_3D ( 'NONE', #20857, #19281, #23091 ) ;
#2880=VERTEX_POINT ( 'NONE', #6122 ) ;
#2881=ORIENTED_EDGE ( 'NONE', *, *, #11890, .T. ) ;
#2883=CARTESIAN_POINT ( 'NONE',  ( 30.45149776762725224, -6.317933499823547017, -6.500000000000000000 ) ) ;
#2888=AXIS2_PLACEMENT_3D ( 'NONE', #5067, #6893, #15144 ) ;
#2894=VECTOR ( 'NONE', #18580, 1000.000000000000000 ) ;
#2899=DIRECTION ( 'NONE',  ( 0.000000000000000000, 0.000000000000000000, 1.000000000000000000 ) ) ;
#2900=LINE ( 'NONE', #9048, #3802 ) ;
#2903=EDGE_CURVE ( 'NONE', #17608, #5905, #25059, .T. ) ;
#2906=VERTEX_POINT ( 'NONE', #25874 ) ;
#2908=VECTOR ( 'NONE', #7277, 1000.000000000000000 ) ;
#2909=EDGE_CURVE ( 'NONE', #14282, #4475, #7706, .T. ) ;
#2910=AXIS2_PLACEMENT_3D ( 'NONE', #13480, #17897, #25875 ) ;
#2911=ORIENTED_EDGE ( 'NONE', *, *, #24526, .F. ) ;
#2912=CARTESIAN_POINT ( 'NONE',  ( 0.000000000000000000, 0.000000000000000000, 1.000000000000000000 ) ) ;
#2915=EDGE_CURVE ( 'NONE', #19787, #21069, #1830, .T. ) ;
#2918=AXIS2_PLACEMENT_3D ( 'NONE', #2764, #11001, #17022 ) ;
#2919=AXIS2_PLACEMENT_3D ( 'NONE', #19547, #8182, #9876 ) ;
#2922=EDGE_CURVE ( 'NONE', #2906, #414, #9197, .T. ) ;
#2923=DIRECTION ( 'NONE',  ( 0.000000000000000000, 0.000000000000000000, 1.000000000000000000 ) ) ;
#2926=VECTOR ( 'NONE', #17138, 1000.000000000000000 ) ;
#2927=FACE_OUTER_BOUND ( 'NONE', #23153, .T. ) ;
#2930=CIRCLE ( 'NONE', #9201, 31.10000000000000142 ) ;
#2935=CARTESIAN_POINT ( 'NONE',  ( 0.000000000000000000, 31.10000000000000142, 1.000000000000000000 ) ) ;
#2941=DIRECTION ( 'NONE',  ( 0.8763066800438685799, 0.4817536741017063306, 0.000000000000000000 ) ) ;
#2943=DIRECTION ( 'NONE',  ( 0.000000000000000000, 0.000000000000000000, -1.000000000000000000 ) ) ;
#2947=CYLINDRICAL_SURFACE ( 'NONE', #25419, 0.5000000000000004441 ) ;
#2948=CIRCLE ( 'NONE', #13807, 0.5000000000000003331 ) ;
#2949=CIRCLE ( 'NONE', #6693, 0.5000000000000004441 ) ;
#2951=ORIENTED_EDGE ( 'NONE', *, *, #17946, .T. ) ;
#2952=EDGE_CURVE ( 'NONE', #21505, #13603, #3912, .T. ) ;
#2953=AXIS2_PLACEMENT_3D ( 'NONE', #18009, #8314, #18527 ) ;
#2963=DIRECTION ( 'NONE',  ( 1.000000000000000000, 0.000000000000000000, 0.000000000000000000 ) ) ;
#2965=CARTESIAN_POINT ( 'NONE',  ( 14.98253926456337837, 27.25313774936414291, -6.500000000000000000 ) ) ;
#2966=CYLINDRICAL_SURFACE ( 'NONE', #13424, 31.10000000000000142 ) ;
#2971=DIRECTION ( 'NONE',  ( 0.000000000000000000, 0.000000000000000000, 1.000000000000000000 ) ) ;
#2973=DIRECTION ( 'NONE',  ( 0.000000000000000000, 0.000000000000000000, 1.000000000000000000 ) ) ;
#2975=CARTESIAN_POINT ( 'NONE',  ( 29.72853858738278987, -9.133673601486577809, 1.000000000000000000 ) ) ;
#2976=ORIENTED_EDGE ( 'NONE', *, *, #24436, .T. ) ;
#2977=CARTESIAN_POINT ( 'NONE',  ( 0.000000000000000000, 0.000000000000000000, 1.000000000000000000 ) ) ;
#2983=AXIS2_PLACEMENT_3D ( 'NONE', #9865, #5809, #2020 ) ;
#2984=EDGE_LOOP ( 'NONE', ( #16925, #4086, #24094, #23586 ) ) ;
#2988=ORIENTED_EDGE ( 'NONE', *, *, #21118, .F. ) ;
#2993=DIRECTION ( 'NONE',  ( 1.000000000000000000, 0.000000000000000000, 0.000000000000000000 ) ) ;
#3000=CYLINDRICAL_SURFACE ( 'NONE', #19238, 31.10000000000000142 ) ;
#3002=CYLINDRICAL_SURFACE ( 'NONE', #20478, 0.5000000000000000000 ) ;
#3004=CARTESIAN_POINT ( 'NONE',  ( -4.393401135981330086, -30.78811501957140351, -6.500000000000000000 ) ) ;
#3005=CARTESIAN_POINT ( 'NONE',  ( 30.63887302793244061, -5.335677986744896906, 1.000000000000000000 ) ) ;
#3007=AXIS2_PLACEMENT_3D ( 'NONE', #5748, #13734, #21711 ) ;
#3009=CIRCLE ( 'NONE', #7174, 0.4999999999999991673 ) ;
#3014=DIRECTION ( 'NONE',  ( -0.000000000000000000, 0.000000000000000000, -1.000000000000000000 ) ) ;
#3015=CYLINDRICAL_SURFACE ( 'NONE', #4153, 31.10000000000000142 ) ;
#3017=AXIS2_PLACEMENT_3D ( 'NONE', #21054, #1045, #303 ) ;
#3018=VERTEX_POINT ( 'NONE', #12234 ) ;
#3019=ORIENTED_EDGE ( 'NONE', *, *, #5268, .T. ) ;
#3024=AXIS2_PLACEMENT_3D ( 'NONE', #18051, #19979, #4166 ) ;
#3030=CIRCLE ( 'NONE', #5124, 31.10000000000000142 ) ;
#3032=DIRECTION ( 'NONE',  ( 1.000000000000000000, 0.000000000000000000, 0.000000000000000000 ) ) ;
#3040=DIRECTION ( 'NONE',  ( -0.8763066800438602533, 0.4817536741017213187, 0.000000000000000000 ) ) ;
#3042=CARTESIAN_POINT ( 'NONE',  ( 0.000000000000000000, 0.000000000000000000, 1.000000000000000000 ) ) ;
#3043=VECTOR ( 'NONE', #4699, 1000.000000000000000 ) ;
#3048=ORIENTED_EDGE ( 'NONE', *, *, #8670, .F. ) ;
#3049=CARTESIAN_POINT ( 'NONE',  ( -18.68225429291695860, 24.86329371854795056, 1.000000000000000000 ) ) ;
#3052=EDGE_LOOP ( 'NONE', ( #13152, #12062 ) ) ;
#3054=CIRCLE ( 'NONE', #12225, 0.4999999999999999445 ) ;
#3055=ORIENTED_EDGE ( 'NONE', *, *, #22866, .T. ) ;
#3058=EDGE_CURVE ( 'NONE', #23094, #22605, #25178, .T. ) ;
#3062=DIRECTION ( 'NONE',  ( 1.000000000000000000, 0.000000000000000000, 0.000000000000000000 ) ) ;
#3063=EDGE_CURVE ( 'NONE', #2607, #4728, #20997, .T. ) ;
#3064=EDGE_CURVE ( 'NONE', #23924, #18764, #11689, .T. ) ;
#3068=ORIENTED_EDGE ( 'NONE', *, *, #25224, .T. ) ;
#3069=EDGE_CURVE ( 'NONE', #5761, #9189, #3193, .T. ) ;
#3075=DIRECTION ( 'NONE',  ( -0.000000000000000000, 0.000000000000000000, 1.000000000000000000 ) ) ;
#3078=ORIENTED_EDGE ( 'NONE', *, *, #4498, .F. ) ;
#3079=DIRECTION ( 'NONE',  ( 0.000000000000000000, 0.000000000000000000, 1.000000000000000000 ) ) ;
#3081=ORIENTED_EDGE ( 'NONE', *, *, #13459, .F. ) ;
#3084=CARTESIAN_POINT ( 'NONE',  ( -26.52310962334755473, -16.23990935651699985, 1.000000000000000000 ) ) ;
#3085=CARTESIAN_POINT ( 'NONE',  ( 7.248980000274197977, 30.24338421796781518, -6.500000000000000000 ) ) ;
#3096=DIRECTION ( 'NONE',  ( -0.000000000000000000, 0.000000000000000000, -1.000000000000000000 ) ) ;
#3103=CARTESIAN_POINT ( 'NONE',  ( -29.57785765677917311, 9.610428525061202265, -6.500000000000000000 ) ) ;
#3105=DIRECTION ( 'NONE',  ( 0.000000000000000000, 0.000000000000000000, 1.000000000000000000 ) ) ;
#3110=DIRECTION ( 'NONE',  ( 0.000000000000000000, -0.000000000000000000, 1.000000000000000000 ) ) ;
#3113=ORIENTED_EDGE ( 'NONE', *, *, #1697, .T. ) ;
#3119=DIRECTION ( 'NONE',  ( 0.000000000000000000, -0.000000000000000000, 1.000000000000000000 ) ) ;
#3120=CYLINDRICAL_SURFACE ( 'NONE', #20869, 31.10000000000000142 ) ;
#3122=DIRECTION ( 'NONE',  ( 1.000000000000000000, 0.000000000000000000, 0.000000000000000000 ) ) ;
#3125=DIRECTION ( 'NONE',  ( 1.000000000000000000, 0.000000000000000000, 0.000000000000000000 ) ) ;
#3131=DIRECTION ( 'NONE',  ( 1.000000000000000000, 0.000000000000000000, 0.000000000000000000 ) ) ;
#3132=EDGE_CURVE ( 'NONE', #14371, #18149, #17208, .T. ) ;
#3133=CARTESIAN_POINT ( 'NONE',  ( -16.66421332384646448, 26.25859848311288403, 1.000000000000000000 ) ) ;
#3137=FACE_OUTER_BOUND ( 'NONE', #23201, .T. ) ;
#3142=DIRECTION ( 'NONE',  ( 0.000000000000000000, 0.000000000000000000, 1.000000000000000000 ) ) ;
#3146=ORIENTED_EDGE ( 'NONE', *, *, #18494, .T. ) ;
#3160=DIRECTION ( 'NONE',  ( 0.000000000000000000, 0.000000000000000000, 1.000000000000000000 ) ) ;
#3161=CYLINDRICAL_SURFACE ( 'NONE', #19229, 31.10000000000000142 ) ;
#3163=DIRECTION ( 'NONE',  ( 0.000000000000000000, -0.000000000000000000, 1.000000000000000000 ) ) ;
#3164=CARTESIAN_POINT ( 'NONE',  ( 30.63887302793244061, -5.335677986744896906, -6.500000000000000000 ) ) ;
#3166=ORIENTED_EDGE ( 'NONE', *, *, #20668, .T. ) ;
#3169=VERTEX_POINT ( 'NONE', #23204 ) ;
#3170=AXIS2_PLACEMENT_3D ( 'NONE', #1060, #6577, #18619 ) ;
#3173=CARTESIAN_POINT ( 'NONE',  ( 29.41953157733093960, 10.08469938919488484, -6.500000000000000000 ) ) ;
#3176=DIRECTION ( 'NONE',  ( -0.3090169943749382919, 0.9510565162951566398, 0.000000000000000000 ) ) ;
#3179=DIRECTION ( 'NONE',  ( 1.000000000000000000, 0.000000000000000000, 0.000000000000000000 ) ) ;
#3185=DIRECTION ( 'NONE',  ( -0.000000000000000000, -0.000000000000000000, 1.000000000000000000 ) ) ;
#3186=VERTEX_POINT ( 'NONE', #21239 ) ;
#3187=EDGE_LOOP ( 'NONE', ( #11686, #635 ) ) ;
#3193=LINE ( 'NONE', #23087, #19214 ) ;
#3196=CYLINDRICAL_SURFACE ( 'NONE', #12476, 31.10000000000000142 ) ;
#3198=ORIENTED_EDGE ( 'NONE', *, *, #6598, .T. ) ;
#3200=ADVANCED_FACE ( 'NONE', ( #1892 ), #19521, .T. ) ;
#3201=DIRECTION ( 'NONE',  ( 0.000000000000000000, -0.000000000000000000, 1.000000000000000000 ) ) ;
#3203=CARTESIAN_POINT ( 'NONE',  ( -29.09636799667086748, -10.98232076577202676, 1.000000000000000000 ) ) ;
#3207=CARTESIAN_POINT ( 'NONE',  ( -11.44867358849371541, -28.91604871112453168, -6.500000000000000000 ) ) ;
#3208=CARTESIAN_POINT ( 'NONE',  ( -25.16042852506104666, -18.28012134629567598, -6.500000000000000000 ) ) ;
#3215=CARTESIAN_POINT ( 'NONE',  ( 0.000000000000000000, 0.000000000000000000, 0.000000000000000000 ) ) ;
#3217=DIRECTION ( 'NONE',  ( 1.000000000000000000, 0.000000000000000000, 0.000000000000000000 ) ) ;
#3222=CYLINDRICAL_SURFACE ( 'NONE', #1662, 31.10000000000000142 ) ;
#3223=ORIENTED_EDGE ( 'NONE', *, *, #12704, .F. ) ;
#3225=EDGE_CURVE ( 'NONE', #14766, #18150, #17142, .T. ) ;
#3228=VERTEX_POINT ( 'NONE', #17838 ) ;
#3229=VERTEX_POINT ( 'NONE', #15748 ) ;
#3230=EDGE_CURVE ( 'NONE', #2553, #22371, #12534, .T. ) ;
#3233=LINE ( 'NONE', #17374, #9349 ) ;
#3234=EDGE_CURVE ( 'NONE', #19968, #4306, #4187, .T. ) ;
#3236=FACE_OUTER_BOUND ( 'NONE', #8525, .T. ) ;
#3242=CARTESIAN_POINT ( 'NONE',  ( -25.45105997952938637, -17.87326343783915306, -2.750000000000000000 ) ) ;
#3243=DIRECTION ( 'NONE',  ( 1.000000000000000000, 0.000000000000000000, 0.000000000000000000 ) ) ;
#3250=APPLICATION_CONTEXT ( 'automotive_design' ) ;
#3251=ORIENTED_EDGE ( 'NONE', *, *, #15969, .T. ) ;
#3254=DIRECTION ( 'NONE',  ( 0.000000000000000000, 0.000000000000000000, 1.000000000000000000 ) ) ;
#3258=VERTEX_POINT ( 'NONE', #13653 ) ;
#3259=VERTEX_POINT ( 'NONE', #7889 ) ;
#3260=VERTEX_POINT ( 'NONE', #25807 ) ;
#3264=CIRCLE ( 'NONE', #23719, 0.5000000000000013323 ) ;
#3265=EDGE_CURVE ( 'NONE', #13534, #6671, #7964, .T. ) ;
#3266=CARTESIAN_POINT ( 'NONE',  ( 0.000000000000000000, 0.000000000000000000, -6.500000000000000000 ) ) ;
#3272=CARTESIAN_POINT ( 'NONE',  ( 27.49048467073858859, 14.54246377227349463, -6.500000000000000000 ) ) ;
#3273=CIRCLE ( 'NONE', #9957, 0.4999999999999991118 ) ;
#3274=DIRECTION ( 'NONE',  ( -0.000000000000000000, 0.000000000000000000, 1.000000000000000000 ) ) ;
#3276=CIRCLE ( 'NONE', #24576, 0.5000000000000001110 ) ;
#3277=DIRECTION ( 'NONE',  ( 0.000000000000000000, 0.000000000000000000, 1.000000000000000000 ) ) ;
#3278=DIRECTION ( 'NONE',  ( 0.000000000000000000, 0.000000000000000000, 1.000000000000000000 ) ) ;
#3279=CARTESIAN_POINT ( 'NONE',  ( 30.78811501957144969, 4.393401135981008565, -6.500000000000000000 ) ) ;
#3284=VECTOR ( 'NONE', #7814, 1000.000000000000000 ) ;
#3288=VERTEX_POINT ( 'NONE', #11940 ) ;
#3290=CYLINDRICAL_SURFACE ( 'NONE', #18369, 0.5000000000000004441 ) ;
#3293=ORIENTED_EDGE ( 'NONE', *, *, #14907, .T. ) ;
#3295=AXIS2_PLACEMENT_3D ( 'NONE', #7997, #21983, #12029 ) ;
#3299=CARTESIAN_POINT ( 'NONE',  ( 0.000000000000000000, 0.000000000000000000, -6.500000000000000000 ) ) ;
#3300=CIRCLE ( 'NONE', #7907, 31.10000000000000142 ) ;
#3302=CIRCLE ( 'NONE', #17925, 0.4999999999999996114 ) ;
#3303=CYLINDRICAL_SURFACE ( 'NONE', #18438, 0.5000000000000004441 ) ;
#3306=DIRECTION ( 'NONE',  ( -0.000000000000000000, -0.000000000000000000, 1.000000000000000000 ) ) ;
#3308=CIRCLE ( 'NONE', #17942, 0.5000000000000007772 ) ;
#3311=DIRECTION ( 'NONE',  ( 0.000000000000000000, 0.000000000000000000, 1.000000000000000000 ) ) ;
#3312=ORIENTED_EDGE ( 'NONE', *, *, #11200, .F. ) ;
#3316=CARTESIAN_POINT ( 'NONE',  ( -10.98232076577180649, 29.09636799667095630, -6.500000000000000000 ) ) ;
#3318=CARTESIAN_POINT ( 'NONE',  ( -3.397863563849436108, 30.85476721088031482, -6.500000000000000000 ) ) ;
#3319=VECTOR ( 'NONE', #23736, 1000.000000000000000 ) ;
#3321=DIRECTION ( 'NONE',  ( 0.000000000000000000, 0.000000000000000000, -1.000000000000000000 ) ) ;
#3322=EDGE_LOOP ( 'NONE', ( #21033, #9702, #24347, #10136 ) ) ;
#3323=VERTEX_POINT ( 'NONE', #1498 ) ;
#3324=CARTESIAN_POINT ( 'NONE',  ( 0.000000000000000000, 0.000000000000000000, -6.500000000000000000 ) ) ;
#3326=ORIENTED_EDGE ( 'NONE', *, *, #21610, .F. ) ;
#3332=CIRCLE ( 'NONE', #17122, 0.4999999999999999445 ) ;
#3336=FACE_OUTER_BOUND ( 'NONE', #16051, .T. ) ;
#3338=DIRECTION ( 'NONE',  ( 0.000000000000000000, 0.000000000000000000, 1.000000000000000000 ) ) ;
#3340=DIRECTION ( 'NONE',  ( 0.000000000000000000, 0.000000000000000000, -1.000000000000000000 ) ) ;
#3342=CIRCLE ( 'NONE', #3753, 0.5000000000000005551 ) ;
#3343=CARTESIAN_POINT ( 'NONE',  ( 24.27856662945507438, 19.43607991388980238, -6.500000000000000000 ) ) ;
#3348=VECTOR ( 'NONE', #18603, 1000.000000000000000 ) ;
#3353=ORIENTED_EDGE ( 'NONE', *, *, #24202, .T. ) ;
#3358=ORIENTED_EDGE ( 'NONE', *, *, #16174, .T. ) ;
#3360=EDGE_LOOP ( 'NONE', ( #7856, #5830, #23652, #3251 ) ) ;
#3362=ORIENTED_EDGE ( 'NONE', *, *, #11269, .T. ) ;
#3364=CYLINDRICAL_SURFACE ( 'NONE', #12647, 31.10000000000000142 ) ;
#3366=AXIS2_PLACEMENT_3D ( 'NONE', #19560, #6094, #20081 ) ;
#3373=AXIS2_PLACEMENT_3D ( 'NONE', #11351, #17494, #19332 ) ;
#3377=CARTESIAN_POINT ( 'NONE',  ( -22.17092431280563503, 21.28941499438250062, -6.500000000000000000 ) ) ;
#3379=DIRECTION ( 'NONE',  ( 0.000000000000000000, 0.000000000000000000, 1.000000000000000000 ) ) ;
#3380=DIRECTION ( 'NONE',  ( 0.000000000000000000, 0.000000000000000000, 1.000000000000000000 ) ) ;
#3385=AXIS2_PLACEMENT_3D ( 'NONE', #11697, #1777, #16026 ) ;
#3387=LINE ( 'NONE', #25239, #4733 ) ;
#3388=ORIENTED_EDGE ( 'NONE', *, *, #14330, .F. ) ;
#3390=EDGE_CURVE ( 'NONE', #17006, #10323, #14246, .T. ) ;
#3391=CARTESIAN_POINT ( 'NONE',  ( -27.49048467073837898, 14.54246377227389075, -6.500000000000000000 ) ) ;
#3392=CARTESIAN_POINT ( 'NONE',  ( 0.000000000000000000, 0.000000000000000000, 1.000000000000000000 ) ) ;
#3393=EDGE_LOOP ( 'NONE', ( #4729, #20675, #20171, #8284 ) ) ;
#3394=AXIS2_PLACEMENT_3D ( 'NONE', #8989, #24422, #6499 ) ;
#3396=ORIENTED_EDGE ( 'NONE', *, *, #7684, .T. ) ;
#3397=VERTEX_POINT ( 'NONE', #4480 ) ;
#3398=VERTEX_POINT ( 'NONE', #20302 ) ;
#3399=EDGE_LOOP ( 'NONE', ( #23435, #8641, #417, #23627 ) ) ;
#3400=DIRECTION ( 'NONE',  ( 1.000000000000000000, 0.000000000000000000, 0.000000000000000000 ) ) ;
#3409=DIRECTION ( 'NONE',  ( 1.000000000000000000, 0.000000000000000000, 0.000000000000000000 ) ) ;
#3415=FACE_OUTER_BOUND ( 'NONE', #24009, .T. ) ;
#3416=EDGE_CURVE ( 'NONE', #9389, #1951, #35, .T. ) ;
#3421=CARTESIAN_POINT ( 'NONE',  ( -10.94867358849309547, 28.91604871112477326, -6.500000000000000000 ) ) ;
#3422=CARTESIAN_POINT ( 'NONE',  ( -15.41874213889433776, -27.00874656207289704, -2.750000000000000000 ) ) ;
#3425=EDGE_CURVE ( 'NONE', #9259, #14853, #11294, .T. ) ;
#3426=CARTESIAN_POINT ( 'NONE',  ( 5.335677986744788548, 30.63887302793246548, -2.750000000000000000 ) ) ;
#3431=ORIENTED_EDGE ( 'NONE', *, *, #4672, .F. ) ;
#3435=ORIENTED_EDGE ( 'NONE', *, *, #14268, .F. ) ;
#3440=CIRCLE ( 'NONE', #1355, 0.5000000000000006661 ) ;
#3442=DIRECTION ( 'NONE',  ( 0.000000000000000000, -0.000000000000000000, 1.000000000000000000 ) ) ;
#3443=CARTESIAN_POINT ( 'NONE',  ( -31.10000000000000142, 3.257552089140643357E-13, -6.500000000000000000 ) ) ;
#3448=AXIS2_PLACEMENT_3D ( 'NONE', #24195, #6806, #16368 ) ;
#3450=DIRECTION ( 'NONE',  ( 0.000000000000000000, 0.000000000000000000, 1.000000000000000000 ) ) ;
#3451=ORIENTED_EDGE ( 'NONE', *, *, #23269, .T. ) ;
#3452=EDGE_CURVE ( 'NONE', #10325, #4475, #14652, .T. ) ;
#3460=DIRECTION ( 'NONE',  ( -0.9510565162951561957, -0.3090169943749392911, 0.000000000000000000 ) ) ;
#3461=EDGE_LOOP ( 'NONE', ( #4451, #3737, #12560, #12370 ) ) ;
#3462=VERTEX_POINT ( 'NONE', #22922 ) ;
#3464=EDGE_CURVE ( 'NONE', #16823, #12173, #7549, .T. ) ;
#3465=AXIS2_PLACEMENT_3D ( 'NONE', #21629, #2154, #17589 ) ;
#3466=CYLINDRICAL_SURFACE ( 'NONE', #20703, 31.10000000000000142 ) ;
#3471=VECTOR ( 'NONE', #23774, 1000.000000000000000 ) ;
#3475=DIRECTION ( 'NONE',  ( 0.000000000000000000, 0.000000000000000000, 1.000000000000000000 ) ) ;
#3476=CARTESIAN_POINT ( 'NONE',  ( -1.453535542772161238, 31.06601413805604750, -2.750000000000000000 ) ) ;
#3477=CIRCLE ( 'NONE', #21463, 0.4999999999999995004 ) ;
#3483=FACE_OUTER_BOUND ( 'NONE', #4356, .T. ) ;
#3486=ADVANCED_FACE ( 'NONE', ( #23059 ), #11019, .F. ) ;
#3489=ORIENTED_EDGE ( 'NONE', *, *, #4704, .T. ) ;
#3494=ORIENTED_EDGE ( 'NONE', *, *, #20508, .F. ) ;
#3503=ADVANCED_FACE ( 'NONE', ( #2663 ), #10625, .F. ) ;
#3504=CIRCLE ( 'NONE', #14787, 0.5000000000000013323 ) ;
#3507=CYLINDRICAL_SURFACE ( 'NONE', #942, 0.5000000000000004441 ) ;
#3509=DIRECTION ( 'NONE',  ( 1.000000000000000000, 0.000000000000000000, 0.000000000000000000 ) ) ;
#3510=STYLED_ITEM ( 'NONE', ( #5333 ), #16592 ) ;
#3513=LINE ( 'NONE', #17498, #11208 ) ;
#3517=LINE ( 'NONE', #9661, #8400 ) ;
#3526=ORIENTED_EDGE ( 'NONE', *, *, #14414, .T. ) ;
#3527=ORIENTED_EDGE ( 'NONE', *, *, #21031, .T. ) ;
#3528=ORIENTED_EDGE ( 'NONE', *, *, #3225, .T. ) ;
#3532=DIRECTION ( 'NONE',  ( 0.000000000000000000, -0.000000000000000000, 1.000000000000000000 ) ) ;
#3534=DIRECTION ( 'NONE',  ( 0.4817536741017131585, -0.8763066800438648052, 0.000000000000000000 ) ) ;
#3539=DIRECTION ( 'NONE',  ( -0.000000000000000000, -0.000000000000000000, 1.000000000000000000 ) ) ;
#3546=DIRECTION ( 'NONE',  ( 0.000000000000000000, 0.000000000000000000, 1.000000000000000000 ) ) ;
#3547=FACE_OUTER_BOUND ( 'NONE', #7383, .T. ) ;
#3550=ADVANCED_FACE ( 'NONE', ( #13955 ), #97, .F. ) ;
#3552=EDGE_LOOP ( 'NONE', ( #3048, #99, #5644, #20396 ) ) ;
#3557=ORIENTED_EDGE ( 'NONE', *, *, #12840, .T. ) ;
#3560=VERTEX_POINT ( 'NONE', #16050 ) ;
#3563=CARTESIAN_POINT ( 'NONE',  ( 0.000000000000000000, 0.000000000000000000, -6.500000000000000000 ) ) ;
#3564=VECTOR ( 'NONE', #12295, 1000.000000000000000 ) ;
#3569=EDGE_CURVE ( 'NONE', #4968, #24375, #11725, .T. ) ;
#3576=AXIS2_PLACEMENT_3D ( 'NONE', #452, #24380, #8425 ) ;
#3577=ORIENTED_EDGE ( 'NONE', *, *, #21161, .T. ) ;
#3578=VERTEX_POINT ( 'NONE', #1664 ) ;
#3580=EDGE_LOOP ( 'NONE', ( #5554, #4297, #3745, #11494 ) ) ;
#3583=DIRECTION ( 'NONE',  ( 0.000000000000000000, 0.000000000000000000, 1.000000000000000000 ) ) ;
#3587=ORIENTED_EDGE ( 'NONE', *, *, #17336, .T. ) ;
#3596=DIRECTION ( 'NONE',  ( 1.000000000000000000, 0.000000000000000000, 0.000000000000000000 ) ) ;
#3597=EDGE_CURVE ( 'NONE', #5826, #3462, #21331, .T. ) ;
#3598=DIRECTION ( 'NONE',  ( 1.000000000000000000, 0.000000000000000000, 0.000000000000000000 ) ) ;
#3603=LINE ( 'NONE', #21403, #20510 ) ;
#3608=CARTESIAN_POINT ( 'NONE',  ( 30.91344420362547041, 3.401318489841111514, 1.000000000000000000 ) ) ;
#3619=ORIENTED_EDGE ( 'NONE', *, *, #25271, .F. ) ;
#3620=DIRECTION ( 'NONE',  ( -0.000000000000000000, -0.000000000000000000, 1.000000000000000000 ) ) ;
#3622=ADVANCED_FACE ( 'NONE', ( #7678 ), #15662, .T. ) ;
#3624=EDGE_CURVE ( 'NONE', #10717, #21352, #1281, .T. ) ;
#3627=CARTESIAN_POINT ( 'NONE',  ( 31.10000000000000142, -1.085850696380214537E-13, -6.500000000000000000 ) ) ;
#3632=DIRECTION ( 'NONE',  ( -0.000000000000000000, -0.000000000000000000, 1.000000000000000000 ) ) ;
#3633=DIRECTION ( 'NONE',  ( 1.000000000000000000, 0.000000000000000000, 0.000000000000000000 ) ) ;
#3634=ORIENTED_EDGE ( 'NONE', *, *, #18266, .T. ) ;
#3638=EDGE_CURVE ( 'NONE', #22500, #1446, #1699, .T. ) ;
#3640=ORIENTED_EDGE ( 'NONE', *, *, #7545, .T. ) ;
#3642=FACE_OUTER_BOUND ( 'NONE', #24853, .T. ) ;
#3645=ORIENTED_EDGE ( 'NONE', *, *, #19553, .F. ) ;
#3649=CARTESIAN_POINT ( 'NONE',  ( -28.41604871112473418, -11.44867358849319849, -6.500000000000000000 ) ) ;
#3650=CYLINDRICAL_SURFACE ( 'NONE', #12787, 31.10000000000000142 ) ;
#3651=DIRECTION ( 'NONE',  ( -0.000000000000000000, -0.000000000000000000, 1.000000000000000000 ) ) ;
#3659=DIRECTION ( 'NONE',  ( -0.000000000000000000, 0.000000000000000000, 1.000000000000000000 ) ) ;
#3663=FACE_OUTER_BOUND ( 'NONE', #758, .T. ) ;
#3666=DIRECTION ( 'NONE',  ( 0.000000000000000000, 0.000000000000000000, 1.000000000000000000 ) ) ;
#3669=CYLINDRICAL_SURFACE ( 'NONE', #13071, 31.10000000000000142 ) ;
#3670=ORIENTED_EDGE ( 'NONE', *, *, #17830, .T. ) ;
#3671=DIRECTION ( 'NONE',  ( 0.000000000000000000, -0.000000000000000000, 1.000000000000000000 ) ) ;
#3672=ORIENTED_EDGE ( 'NONE', *, *, #9994, .T. ) ;
#3673=ORIENTED_EDGE ( 'NONE', *, *, #9968, .T. ) ;
#3676=AXIS2_PLACEMENT_3D ( 'NONE', #24845, #12547, #399 ) ;
#3677=ORIENTED_EDGE ( 'NONE', *, *, #3960, .T. ) ;
#3679=VERTEX_POINT ( 'NONE', #18386 ) ;
#3680=DIRECTION ( 'NONE',  ( 1.000000000000000000, 0.000000000000000000, 0.000000000000000000 ) ) ;
#3681=ORIENTED_EDGE ( 'NONE', *, *, #22094, .T. ) ;
#3684=CIRCLE ( 'NONE', #18312, 0.5000000000000005551 ) ;
#3690=CIRCLE ( 'NONE', #4117, 31.10000000000000142 ) ;
#3695=CARTESIAN_POINT ( 'NONE',  ( -24.86329371854788661, -18.68225429291705098, 1.000000000000000000 ) ) ;
#3700=ORIENTED_EDGE ( 'NONE', *, *, #1391, .T. ) ;
#3701=CARTESIAN_POINT ( 'NONE',  ( -22.32573188046889356, 21.65113613650366986, -2.750000000000000000 ) ) ;
#3702=AXIS2_PLACEMENT_3D ( 'NONE', #22447, #10666, #24808 ) ;
#3704=DIRECTION ( 'NONE',  ( 1.000000000000000000, 0.000000000000000000, 0.000000000000000000 ) ) ;
#3709=ORIENTED_EDGE ( 'NONE', *, *, #13815, .T. ) ;
#3718=CIRCLE ( 'NONE', #7076, 31.10000000000000142 ) ;
#3719=CYLINDRICAL_SURFACE ( 'NONE', #13861, 31.10000000000000142 ) ;
#3721=VECTOR ( 'NONE', #985, 1000.000000000000000 ) ;
#3735=EDGE_CURVE ( 'NONE', #2553, #19625, #4268, .T. ) ;
#3737=ORIENTED_EDGE ( 'NONE', *, *, #25399, .T. ) ;
#3739=AXIS2_PLACEMENT_3D ( 'NONE', #11567, #19535, #19038 ) ;
#3740=EDGE_CURVE ( 'NONE', #1683, #14407, #10452, .T. ) ;
#3741=CARTESIAN_POINT ( 'NONE',  ( -7.234255490826573265, 30.12293631110053838, 1.000000000000000000 ) ) ;
#3742=AXIS2_PLACEMENT_3D ( 'NONE', #24689, #7293, #18939 ) ;
#3745=ORIENTED_EDGE ( 'NONE', *, *, #16115, .T. ) ;
#3750=AXIS2_PLACEMENT_3D ( 'NONE', #25658, #11913, #23434 ) ;
#3753=AXIS2_PLACEMENT_3D ( 'NONE', #25107, #5483, #24973 ) ;
#3756=AXIS2_PLACEMENT_3D ( 'NONE', #12719, #13228, #12971 ) ;
#3760=DIRECTION ( 'NONE',  ( 1.000000000000000000, 0.000000000000000000, 0.000000000000000000 ) ) ;
#3762=CARTESIAN_POINT ( 'NONE',  ( -23.01025686871616216, 20.92219106202074741, -6.500000000000000000 ) ) ;
#3765=DIRECTION ( 'NONE',  ( 0.000000000000000000, 0.000000000000000000, 1.000000000000000000 ) ) ;
#3768=VECTOR ( 'NONE', #19158, 1000.000000000000000 ) ;
#3769=DIRECTION ( 'NONE',  ( 0.4817536741017267032, 0.8763066800438573667, 0.000000000000000000 ) ) ;
#3770=CARTESIAN_POINT ( 'NONE',  ( 5.335677986744788548, 30.63887302793246548, -6.500000000000000000 ) ) ;
#3772=DIRECTION ( 'NONE',  ( 1.000000000000000000, 0.000000000000000000, 0.000000000000000000 ) ) ;
#3781=VERTEX_POINT ( 'NONE', #4220 ) ;
#3783=VERTEX_POINT ( 'NONE', #1997 ) ;
#3784=DIRECTION ( 'NONE',  ( 0.9822872507286911636, 0.1873813145857119722, 0.000000000000000000 ) ) ;
#3785=CIRCLE ( 'NONE', #17165, 0.5000000000000004441 ) ;
#3794=CYLINDRICAL_SURFACE ( 'NONE', #9205, 31.10000000000000142 ) ;
#3795=CARTESIAN_POINT ( 'NONE',  ( -17.08421000182742233, 25.98730014090460472, 1.000000000000000000 ) ) ;
#3798=CARTESIAN_POINT ( 'NONE',  ( -24.66042852506064165, 18.28012134629622309, -6.500000000000000000 ) ) ;
#3800=DIRECTION ( 'NONE',  ( 0.000000000000000000, 0.000000000000000000, 1.000000000000000000 ) ) ;
#3802=VECTOR ( 'NONE', #23048, 1000.000000000000000 ) ;
#3804=AXIS2_PLACEMENT_3D ( 'NONE', #21167, #5095, #3125 ) ;
#3805=PLANE ( 'NONE',  #19525 ) ;
#3806=CARTESIAN_POINT ( 'NONE',  ( -13.24173596767398742, -28.14012133169310559, -6.500000000000000000 ) ) ;
#3808=EDGE_LOOP ( 'NONE', ( #6930, #25612, #13410, #11872 ) ) ;
#3812=ORIENTED_EDGE ( 'NONE', *, *, #17316, .F. ) ;
#3813=CARTESIAN_POINT ( 'NONE',  ( -27.00874656207282953, 15.41874213889444079, -2.750000000000000000 ) ) ;
#3814=ORIENTED_EDGE ( 'NONE', *, *, #4652, .T. ) ;
#3816=ORIENTED_EDGE ( 'NONE', *, *, #6574, .T. ) ;
#3817=CARTESIAN_POINT ( 'NONE',  ( 26.25859848311259981, -16.66421332384692278, -6.500000000000000000 ) ) ;
#3818=EDGE_CURVE ( 'NONE', #12311, #364, #25087, .T. ) ;
#3821=CYLINDRICAL_SURFACE ( 'NONE', #14763, 31.10000000000000142 ) ;
#3822=AXIS2_PLACEMENT_3D ( 'NONE', #22267, #20290, #22386 ) ;
#3824=CARTESIAN_POINT ( 'NONE',  ( 0.000000000000000000, 0.000000000000000000, -6.500000000000000000 ) ) ;
#3827=CIRCLE ( 'NONE', #7604, 0.5000000000000006661 ) ;
#3835=AXIS2_PLACEMENT_3D ( 'NONE', #10057, #4173, #6880 ) ;
#3837=ORIENTED_EDGE ( 'NONE', *, *, #7363, .F. ) ;
#3839=AXIS2_PLACEMENT_3D ( 'NONE', #11898, #24057, #1850 ) ;
#3841=EDGE_LOOP ( 'NONE', ( #22776, #15990, #22244, #20178 ) ) ;
#3844=CARTESIAN_POINT ( 'NONE',  ( -5.827558883615604479, 30.54913349766230724, -6.500000000000000000 ) ) ;
#3845=ORIENTED_EDGE ( 'NONE', *, *, #16029, .F. ) ;
#3850=ORIENTED_EDGE ( 'NONE', *, *, #19484, .F. ) ;
#3852=CARTESIAN_POINT ( 'NONE',  ( -28.72825533807115050, 11.91206721063083229, -2.750000000000000000 ) ) ;
#3858=CIRCLE ( 'NONE', #15131, 0.5000000000000000000 ) ;
#3870=( GEOMETRIC_REPRESENTATION_CONTEXT ( 3 ) GLOBAL_UNCERTAINTY_ASSIGNED_CONTEXT ( ( #14901 ) ) GLOBAL_UNIT_ASSIGNED_CONTEXT ( ( #12798, #14386, #4551 ) ) REPRESENTATION_CONTEXT ( 'NONE', 'WORKASPACE' ) );
#3871=FACE_OUTER_BOUND ( 'NONE', #10260, .T. ) ;
#3873=ORIENTED_EDGE ( 'NONE', *, *, #7691, .F. ) ;
#3878=ORIENTED_EDGE ( 'NONE', *, *, #9853, .F. ) ;
#3882=DIRECTION ( 'NONE',  ( 1.000000000000000000, 0.000000000000000000, 0.000000000000000000 ) ) ;
#3883=ORIENTED_EDGE ( 'NONE', *, *, #1634, .F. ) ;
#3884=ORIENTED_EDGE ( 'NONE', *, *, #19484, .T. ) ;
#3887=ADVANCED_FACE ( 'NONE', ( #13232 ), #3161, .T. ) ;
#3888=AXIS2_PLACEMENT_3D ( 'NONE', #9542, #15191, #15698 ) ;
#3890=EDGE_CURVE ( 'NONE', #4940, #20266, #4620, .T. ) ;
#3894=CARTESIAN_POINT ( 'NONE',  ( -30.24338421796790044, -7.248980000273874680, -6.500000000000000000 ) ) ;
#3895=CARTESIAN_POINT ( 'NONE',  ( -29.57785765677917311, 9.610428525061202265, 1.000000000000000000 ) ) ;
#3898=DIRECTION ( 'NONE',  ( 1.000000000000000000, 0.000000000000000000, 0.000000000000000000 ) ) ;
#3908=CARTESIAN_POINT ( 'NONE',  ( 31.10000000000000142, -1.085850696380214537E-13, -6.500000000000000000 ) ) ;
#3910=ORIENTED_EDGE ( 'NONE', *, *, #10251, .T. ) ;
#3912=LINE ( 'NONE', #6001, #12955 ) ;
#3913=DIRECTION ( 'NONE',  ( 1.000000000000000000, 0.000000000000000000, 0.000000000000000000 ) ) ;
#3914=ORIENTED_EDGE ( 'NONE', *, *, #1319, .T. ) ;
#3916=ORIENTED_EDGE ( 'NONE', *, *, #11089, .T. ) ;
#3917=VERTEX_POINT ( 'NONE', #17940 ) ;
#3919=CARTESIAN_POINT ( 'NONE',  ( 0.000000000000000000, 0.000000000000000000, -6.500000000000000000 ) ) ;
#3920=CARTESIAN_POINT ( 'NONE',  ( -26.52310962334761868, -16.23990935651689327, -2.750000000000000000 ) ) ;
#3929=CYLINDRICAL_SURFACE ( 'NONE', #3839, 0.5000000000000004441 ) ;
#3931=DIRECTION ( 'NONE',  ( 0.000000000000000000, 0.000000000000000000, 1.000000000000000000 ) ) ;
#3933=DIRECTION ( 'NONE',  ( 0.000000000000000000, 0.000000000000000000, 1.000000000000000000 ) ) ;
#3937=DIRECTION ( 'NONE',  ( 0.000000000000000000, -0.000000000000000000, 1.000000000000000000 ) ) ;
#3939=DIRECTION ( 'NONE',  ( 0.000000000000000000, 0.000000000000000000, -1.000000000000000000 ) ) ;
#3940=FACE_OUTER_BOUND ( 'NONE', #17928, .T. ) ;
#3942=LINE ( 'NONE', #4191, #1651 ) ;
#3945=ORIENTED_EDGE ( 'NONE', *, *, #14074, .T. ) ;
#3947=AXIS2_PLACEMENT_3D ( 'NONE', #19346, #19085, #23150 ) ;
#3957=CARTESIAN_POINT ( 'NONE',  ( 23.01025686871646059, 20.92219106202042056, -2.750000000000000000 ) ) ;
#3960=EDGE_CURVE ( 'NONE', #18350, #23781, #16113, .T. ) ;
#3961=CARTESIAN_POINT ( 'NONE',  ( 0.000000000000000000, 0.000000000000000000, 1.000000000000000000 ) ) ;
#3970=EDGE_CURVE ( 'NONE', #14942, #16234, #16337, .T. ) ;
#3976=ORIENTED_EDGE ( 'NONE', *, *, #15921, .T. ) ;
#3977=VECTOR ( 'NONE', #8098, 1000.000000000000000 ) ;
#3980=FACE_OUTER_BOUND ( 'NONE', #10297, .T. ) ;
#3986=CARTESIAN_POINT ( 'NONE',  ( -17.78012134629558716, 25.16042852506110705, -6.500000000000000000 ) ) ;
#3988=EDGE_CURVE ( 'NONE', #6294, #5290, #8005, .T. ) ;
#3989=CARTESIAN_POINT ( 'NONE',  ( -27.25313774936397948, 14.98253926456367502, 1.000000000000000000 ) ) ;
#3995=CARTESIAN_POINT ( 'NONE',  ( 0.000000000000000000, 0.000000000000000000, -6.500000000000000000 ) ) ;
#4001=ADVANCED_FACE ( 'NONE', ( #10329 ), #6039, .F. ) ;
#4003=CARTESIAN_POINT ( 'NONE',  ( 19.82388608118429119, 23.96296185032701587, 1.000000000000000000 ) ) ;
#4011=CARTESIAN_POINT ( 'NONE',  ( -15.41874213889376044, 27.00874656207322388, -6.500000000000000000 ) ) ;
#4015=ADVANCED_FACE ( 'NONE', ( #23822 ), #24205, .T. ) ;
#4016=CYLINDRICAL_SURFACE ( 'NONE', #11732, 0.5000000000000004441 ) ;
#4017=DIRECTION ( 'NONE',  ( 1.000000000000000000, 0.000000000000000000, 0.000000000000000000 ) ) ;
#4022=CYLINDRICAL_SURFACE ( 'NONE', #2549, 0.5000000000000004441 ) ;
#4027=CARTESIAN_POINT ( 'NONE',  ( 29.09636799667079288, 10.98232076577223637, 1.000000000000000000 ) ) ;
#4031=DIRECTION ( 'NONE',  ( 0.000000000000000000, 0.000000000000000000, 1.000000000000000000 ) ) ;
#4038=VERTEX_POINT ( 'NONE', #2883 ) ;
#4039=DIRECTION ( 'NONE',  ( 0.000000000000000000, 0.000000000000000000, 1.000000000000000000 ) ) ;
#4046=DIRECTION ( 'NONE',  ( 0.5877852522924853496, 0.8090169943749385695, 0.000000000000000000 ) ) ;
#4048=DIRECTION ( 'NONE',  ( 0.000000000000000000, 0.000000000000000000, -1.000000000000000000 ) ) ;
#4053=DIRECTION ( 'NONE',  ( 1.000000000000000000, 0.000000000000000000, 0.000000000000000000 ) ) ;
#4055=CARTESIAN_POINT ( 'NONE',  ( -30.78811501957148167, -4.393401135980793626, -6.500000000000000000 ) ) ;
#4056=ORIENTED_EDGE ( 'NONE', *, *, #20696, .F. ) ;
#4059=ORIENTED_EDGE ( 'NONE', *, *, #8340, .F. ) ;
#4061=FACE_OUTER_BOUND ( 'NONE', #14921, .T. ) ;
#4063=ADVANCED_FACE ( 'NONE', ( #18465 ), #2637, .T. ) ;
#4065=VERTEX_POINT ( 'NONE', #8918 ) ;
#4067=EDGE_CURVE ( 'NONE', #9149, #21754, #4679, .T. ) ;
#4069=DIRECTION ( 'NONE',  ( 1.000000000000000000, 0.000000000000000000, 0.000000000000000000 ) ) ;
#4071=FACE_OUTER_BOUND ( 'NONE', #10750, .T. ) ;
#4072=DIRECTION ( 'NONE',  ( 0.000000000000000000, 0.000000000000000000, 1.000000000000000000 ) ) ;
#4074=DIRECTION ( 'NONE',  ( 0.000000000000000000, 0.000000000000000000, 1.000000000000000000 ) ) ;
#4076=AXIS2_PLACEMENT_3D ( 'NONE', #25290, #980, #13395 ) ;
#4082=CARTESIAN_POINT ( 'NONE',  ( 22.67092431280594056, 21.28941499438218088, -6.500000000000000000 ) ) ;
#4084=ORIENTED_EDGE ( 'NONE', *, *, #2780, .T. ) ;
#4086=ORIENTED_EDGE ( 'NONE', *, *, #10046, .F. ) ;
#4087=LINE ( 'NONE', #7639, #7909 ) ;
#4093=EDGE_CURVE ( 'NONE', #17423, #10079, #18848, .T. ) ;
#4094=AXIS2_PLACEMENT_3D ( 'NONE', #22666, #20566, #10616 ) ;
#4096=ORIENTED_EDGE ( 'NONE', *, *, #14893, .T. ) ;
#4101=CARTESIAN_POINT ( 'NONE',  ( -26.52310962334761868, -16.23990935651689327, -6.500000000000000000 ) ) ;
#4104=EDGE_CURVE ( 'NONE', #3462, #10049, #10599, .T. ) ;
#4107=DIRECTION ( 'NONE',  ( 1.000000000000000000, 0.000000000000000000, 0.000000000000000000 ) ) ;
#4108=AXIS2_PLACEMENT_3D ( 'NONE', #4443, #14131, #4720 ) ;
#4110=DIRECTION ( 'NONE',  ( 0.000000000000000000, 0.000000000000000000, 1.000000000000000000 ) ) ;
#4112=FACE_OUTER_BOUND ( 'NONE', #1765, .T. ) ;
#4114=AXIS2_PLACEMENT_3D ( 'NONE', #18804, #20639, #14885 ) ;
#4117=AXIS2_PLACEMENT_3D ( 'NONE', #6724, #14193, #12089 ) ;
#4125=CARTESIAN_POINT ( 'NONE',  ( -21.65113613650310143, 22.32573188046944068, -2.750000000000000000 ) ) ;
#4127=ORIENTED_EDGE ( 'NONE', *, *, #18605, .F. ) ;
#4128=ORIENTED_EDGE ( 'NONE', *, *, #21854, .T. ) ;
#4132=EDGE_CURVE ( 'NONE', #13061, #6542, #22893, .T. ) ;
#4133=CIRCLE ( 'NONE', #18752, 0.5000000000000000000 ) ;
#4135=CIRCLE ( 'NONE', #18757, 0.5000000000000005551 ) ;
#4137=AXIS2_PLACEMENT_3D ( 'NONE', #3806, #8247, #18313 ) ;
#4140=DIRECTION ( 'NONE',  ( 1.000000000000000000, 0.000000000000000000, 0.000000000000000000 ) ) ;
#4151=AXIS2_PLACEMENT_3D ( 'NONE', #4401, #14740, #24927 ) ;
#4152=CARTESIAN_POINT ( 'NONE',  ( -14.54246377227378062, -27.49048467073843227, -6.500000000000000000 ) ) ;
#4153=AXIS2_PLACEMENT_3D ( 'NONE', #19347, #6809, #10986 ) ;
#4155=DIRECTION ( 'NONE',  ( 0.000000000000000000, 0.000000000000000000, 1.000000000000000000 ) ) ;
#4156=ORIENTED_EDGE ( 'NONE', *, *, #7037, .F. ) ;
#4161=ORIENTED_EDGE ( 'NONE', *, *, #15136, .F. ) ;
#4162=CIRCLE ( 'NONE', #20021, 31.10000000000000142 ) ;
#4163=ORIENTED_EDGE ( 'NONE', *, *, #6994, .T. ) ;
#4164=EDGE_LOOP ( 'NONE', ( #4127, #21755, #12241, #24038 ) ) ;
#4165=EDGE_LOOP ( 'NONE', ( #20942, #15306, #17453, #9056 ) ) ;
#4166=DIRECTION ( 'NONE',  ( 1.000000000000000000, 0.000000000000000000, 0.000000000000000000 ) ) ;
#4167=CARTESIAN_POINT ( 'NONE',  ( 13.24173596767378847, 28.14012133169319796, -6.500000000000000000 ) ) ;
#4168=EDGE_CURVE ( 'NONE', #22990, #21593, #24316, .T. ) ;
#4169=AXIS2_PLACEMENT_3D ( 'NONE', #18197, #9823, #158 ) ;
#4171=AXIS2_PLACEMENT_3D ( 'NONE', #12838, #15070, #20956 ) ;
#4172=EDGE_CURVE ( 'NONE', #20797, #12699, #527, .T. ) ;
#4173=DIRECTION ( 'NONE',  ( 0.000000000000000000, 0.000000000000000000, 1.000000000000000000 ) ) ;
#4176=VECTOR ( 'NONE', #2507, 1000.000000000000000 ) ;
#4180=DIRECTION ( 'NONE',  ( 1.000000000000000000, 0.000000000000000000, 0.000000000000000000 ) ) ;
#4187=CIRCLE ( 'NONE', #18814, 31.10000000000000142 ) ;
#4190=ORIENTED_EDGE ( 'NONE', *, *, #21931, .T. ) ;
#4191=CARTESIAN_POINT ( 'NONE',  ( 28.34936733434196299, -12.78762572734067149, -2.750000000000000000 ) ) ;
#4192=DIRECTION ( 'NONE',  ( 0.000000000000000000, 0.000000000000000000, 1.000000000000000000 ) ) ;
#4193=ORIENTED_EDGE ( 'NONE', *, *, #17399, .F. ) ;
#4196=ORIENTED_EDGE ( 'NONE', *, *, #10386, .T. ) ;
#4199=EDGE_LOOP ( 'NONE', ( #20046, #18620, #9848, #6177 ) ) ;
#4200=DIRECTION ( 'NONE',  ( 0.7289686274214236539, 0.6845471059286760696, 0.000000000000000000 ) ) ;
#4202=VERTEX_POINT ( 'NONE', #20676 ) ;
#4207=DIRECTION ( 'NONE',  ( 0.6374239897486995154, 0.7705132427757811486, 0.000000000000000000 ) ) ;
#4212=CIRCLE ( 'NONE', #11302, 0.4999999999999989453 ) ;
#4215=EDGE_CURVE ( 'NONE', #15212, #4065, #5121, .T. ) ;
#4218=VECTOR ( 'NONE', #145, 1000.000000000000000 ) ;
#4220=CARTESIAN_POINT ( 'NONE',  ( -30.78811501957138930, 4.393401135981437555, -6.500000000000000000 ) ) ;
#4226=ORIENTED_EDGE ( 'NONE', *, *, #22255, .F. ) ;
#4230=ORIENTED_EDGE ( 'NONE', *, *, #21894, .T. ) ;
#4232=AXIS2_PLACEMENT_3D ( 'NONE', #4603, #22664, #20691 ) ;
#4233=DIRECTION ( 'NONE',  ( 1.000000000000000000, 0.000000000000000000, 0.000000000000000000 ) ) ;
#4234=EDGE_LOOP ( 'NONE', ( #5141, #21984, #15593, #9325 ) ) ;
#4240=CARTESIAN_POINT ( 'NONE',  ( 0.000000000000000000, 0.000000000000000000, -6.500000000000000000 ) ) ;
#4242=AXIS2_PLACEMENT_3D ( 'NONE', #22924, #5009, #12993 ) ;
#4243=ADVANCED_FACE ( 'NONE', ( #11114 ), #17522, .T. ) ;
#4245=AXIS2_PLACEMENT_3D ( 'NONE', #22012, #12066, #20044 ) ;
#4246=EDGE_CURVE ( 'NONE', #3783, #1051, #23475, .T. ) ;
#4249=DIRECTION ( 'NONE',  ( 0.000000000000000000, 0.000000000000000000, -1.000000000000000000 ) ) ;
#4250=CYLINDRICAL_SURFACE ( 'NONE', #16832, 30.10000000000000142 ) ;
#4251=CARTESIAN_POINT ( 'NONE',  ( -22.67092431280563503, 21.28941499438250062, -6.500000000000000000 ) ) ;
#4253=EDGE_CURVE ( 'NONE', #18011, #18810, #24732, .T. ) ;
#4258=ORIENTED_EDGE ( 'NONE', *, *, #11420, .T. ) ;
#4262=ORIENTED_EDGE ( 'NONE', *, *, #17280, .F. ) ;
#4263=ORIENTED_EDGE ( 'NONE', *, *, #7114, .F. ) ;
#4266=VECTOR ( 'NONE', #24731, 1000.000000000000000 ) ;
#4268=LINE ( 'NONE', #10385, #11704 ) ;
#4269=VERTEX_POINT ( 'NONE', #17400 ) ;
#4278=EDGE_CURVE ( 'NONE', #18972, #5285, #938, .T. ) ;
#4280=ADVANCED_FACE ( 'NONE', ( #11504 ), #11623, .T. ) ;
#4282=AXIS2_PLACEMENT_3D ( 'NONE', #14890, #14632, #10817 ) ;
#4283=CYLINDRICAL_SURFACE ( 'NONE', #5085, 31.10000000000000142 ) ;
#4284=DIRECTION ( 'NONE',  ( 0.000000000000000000, 0.000000000000000000, 1.000000000000000000 ) ) ;
#4285=CARTESIAN_POINT ( 'NONE',  ( 28.91604871112465602, 11.44867358849340633, 1.000000000000000000 ) ) ;
#4290=DIRECTION ( 'NONE',  ( -0.000000000000000000, -0.000000000000000000, 1.000000000000000000 ) ) ;
#4293=DIRECTION ( 'NONE',  ( 0.000000000000000000, 0.000000000000000000, 1.000000000000000000 ) ) ;
#4295=DIRECTION ( 'NONE',  ( -0.6374239897486843054, 0.7705132427757935831, 0.000000000000000000 ) ) ;
#4296=LINE ( 'NONE', #20356, #441 ) ;
#4297=ORIENTED_EDGE ( 'NONE', *, *, #11393, .F. ) ;
#4303=EDGE_CURVE ( 'NONE', #23296, #14980, #21570, .T. ) ;
#4305=ORIENTED_EDGE ( 'NONE', *, *, #5876, .F. ) ;
#4306=VERTEX_POINT ( 'NONE', #13218 ) ;
#4307=CARTESIAN_POINT ( 'NONE',  ( 0.4999838450259764255, -31.09598070739550124, -6.500000000000000000 ) ) ;
#4312=EDGE_CURVE ( 'NONE', #24168, #23712, #19288, .T. ) ;
#4316=DIRECTION ( 'NONE',  ( 0.000000000000000000, 0.000000000000000000, -1.000000000000000000 ) ) ;
#4317=FACE_OUTER_BOUND ( 'NONE', #19471, .T. ) ;
#4318=DIRECTION ( 'NONE',  ( 0.000000000000000000, 0.000000000000000000, 1.000000000000000000 ) ) ;
#4320=DIRECTION ( 'NONE',  ( 0.000000000000000000, -0.000000000000000000, -1.000000000000000000 ) ) ;
#4321=CARTESIAN_POINT ( 'NONE',  ( -29.09636799667067564, 10.98232076577254368, -6.500000000000000000 ) ) ;
#4324=EDGE_CURVE ( 'NONE', #14942, #12173, #18487, .T. ) ;
#4327=CARTESIAN_POINT ( 'NONE',  ( -16.16421332384646448, 26.25859848311288403, -6.500000000000000000 ) ) ;
#4328=EDGE_LOOP ( 'NONE', ( #20005, #25336, #16919, #11886 ) ) ;
#4329=ORIENTED_EDGE ( 'NONE', *, *, #170, .T. ) ;
#4331=EDGE_LOOP ( 'NONE', ( #13956, #2988, #5146, #1954 ) ) ;
#4332=ORIENTED_EDGE ( 'NONE', *, *, #16167, .T. ) ;
#4333=ORIENTED_EDGE ( 'NONE', *, *, #1646, .F. ) ;
#4336=ORIENTED_EDGE ( 'NONE', *, *, #10121, .T. ) ;
#4337=DIRECTION ( 'NONE',  ( -0.000000000000000000, -0.000000000000000000, 1.000000000000000000 ) ) ;
#4339=VECTOR ( 'NONE', #1388, 1000.000000000000000 ) ;
#4346=DIRECTION ( 'NONE',  ( -0.000000000000000000, 0.000000000000000000, -1.000000000000000000 ) ) ;
#4349=DIRECTION ( 'NONE',  ( 0.000000000000000000, -0.000000000000000000, 1.000000000000000000 ) ) ;
#4352=ORIENTED_EDGE ( 'NONE', *, *, #8233, .T. ) ;
#4356=EDGE_LOOP ( 'NONE', ( #8522, #10203, #9764, #4336 ) ) ;
#4363=ORIENTED_EDGE ( 'NONE', *, *, #16025, .F. ) ;
#4364=EDGE_CURVE ( 'NONE', #24045, #9259, #1176, .T. ) ;
#4365=CARTESIAN_POINT ( 'NONE',  ( -21.65113613650310143, 22.32573188046944068, -6.500000000000000000 ) ) ;
#4367=DIRECTION ( 'NONE',  ( 1.000000000000000000, 0.000000000000000000, 0.000000000000000000 ) ) ;
#4368=DIRECTION ( 'NONE',  ( -0.4257792915650782661, -0.9048270524660170233, 0.000000000000000000 ) ) ;
#4377=FACE_OUTER_BOUND ( 'NONE', #4199, .T. ) ;
#4384=ORIENTED_EDGE ( 'NONE', *, *, #11921, .T. ) ;
#4385=DIRECTION ( 'NONE',  ( -0.9822872507286872779, 0.1873813145857327056, 0.000000000000000000 ) ) ;
#4388=ORIENTED_EDGE ( 'NONE', *, *, #6750, .T. ) ;
#4389=ORIENTED_EDGE ( 'NONE', *, *, #10921, .T. ) ;
#4394=EDGE_CURVE ( 'NONE', #5166, #22953, #5519, .T. ) ;
#4396=ADVANCED_FACE ( 'NONE', ( #15308 ), #13345, .T. ) ;
#4398=CARTESIAN_POINT ( 'NONE',  ( -13.24173596767339767, 28.14012133169338270, -6.500000000000000000 ) ) ;
#4401=CARTESIAN_POINT ( 'NONE',  ( -18.28012134629558716, 25.16042852506110705, -6.500000000000000000 ) ) ;
#4402=CARTESIAN_POINT ( 'NONE',  ( 14.54246377227340048, -27.49048467073863833, -2.750000000000000000 ) ) ;
#4407=ORIENTED_EDGE ( 'NONE', *, *, #11890, .F. ) ;
#4408=CARTESIAN_POINT ( 'NONE',  ( 0.000000000000000000, 0.000000000000000000, -6.500000000000000000 ) ) ;
#4409=FACE_OUTER_BOUND ( 'NONE', #21758, .T. ) ;
#4418=DIRECTION ( 'NONE',  ( 0.000000000000000000, 0.000000000000000000, 1.000000000000000000 ) ) ;
#4420=CARTESIAN_POINT ( 'NONE',  ( 31.06601413805602263, -1.453535542772716793, -6.500000000000000000 ) ) ;
#4421=EDGE_LOOP ( 'NONE', ( #18563, #3431, #15528, #4190 ) ) ;
#4423=EDGE_CURVE ( 'NONE', #15106, #7204, #1955, .T. ) ;
#4427=ORIENTED_EDGE ( 'NONE', *, *, #9829, .F. ) ;
#4434=EDGE_CURVE ( 'NONE', #19279, #184, #6767, .T. ) ;
#4436=DIRECTION ( 'NONE',  ( 0.000000000000000000, 0.000000000000000000, 1.000000000000000000 ) ) ;
#4438=DIRECTION ( 'NONE',  ( 0.6374239897486995154, 0.7705132427757811486, 0.000000000000000000 ) ) ;
#4443=CARTESIAN_POINT ( 'NONE',  ( 0.000000000000000000, 0.000000000000000000, 1.000000000000000000 ) ) ;
#4448=CARTESIAN_POINT ( 'NONE',  ( 0.000000000000000000, 0.000000000000000000, -6.500000000000000000 ) ) ;
#4450=ORIENTED_EDGE ( 'NONE', *, *, #24313, .T. ) ;
#4451=ORIENTED_EDGE ( 'NONE', *, *, #5993, .F. ) ;
#4454=ORIENTED_EDGE ( 'NONE', *, *, #24551, .T. ) ;
#4455=VERTEX_POINT ( 'NONE', #22220 ) ;
#4458=CYLINDRICAL_SURFACE ( 'NONE', #23872, 0.5000000000000004441 ) ;
#4460=ADVANCED_FACE ( 'NONE', ( #16084 ), #12279, .T. ) ;
#4464=CARTESIAN_POINT ( 'NONE',  ( 0.000000000000000000, 0.000000000000000000, -6.500000000000000000 ) ) ;
#4469=DIRECTION ( 'NONE',  ( 0.000000000000000000, -0.000000000000000000, 1.000000000000000000 ) ) ;
#4470=DIRECTION ( 'NONE',  ( -0.000000000000000000, -0.000000000000000000, 1.000000000000000000 ) ) ;
#4474=EDGE_LOOP ( 'NONE', ( #12143, #4163, #21216, #18232 ) ) ;
#4475=VERTEX_POINT ( 'NONE', #261 ) ;
#4477=VERTEX_POINT ( 'NONE', #4307 ) ;
#4478=DIRECTION ( 'NONE',  ( 1.000000000000000000, 0.000000000000000000, 0.000000000000000000 ) ) ;
#4479=VERTEX_POINT ( 'NONE', #19857 ) ;
#4480=CARTESIAN_POINT ( 'NONE',  ( -12.78762572734029312, 28.34936733434213352, 1.000000000000000000 ) ) ;
#4481=EDGE_LOOP ( 'NONE', ( #6289, #22861, #1024, #11460 ) ) ;
#4482=CARTESIAN_POINT ( 'NONE',  ( 0.000000000000000000, 0.000000000000000000, 1.000000000000000000 ) ) ;
#4485=ORIENTED_EDGE ( 'NONE', *, *, #20590, .F. ) ;
#4488=DIRECTION ( 'NONE',  ( 1.000000000000000000, 0.000000000000000000, 0.000000000000000000 ) ) ;
#4489=EDGE_CURVE ( 'NONE', #10075, #2553, #14309, .T. ) ;
#4493=EDGE_CURVE ( 'NONE', #14796, #17688, #20148, .T. ) ;
#4495=EDGE_CURVE ( 'NONE', #22067, #5321, #19742, .T. ) ;
#4496=DIRECTION ( 'NONE',  ( 0.7705132427757999114, 0.6374239897486768669, 0.000000000000000000 ) ) ;
#4498=EDGE_CURVE ( 'NONE', #25487, #7861, #8043, .T. ) ;
#4501=DIRECTION ( 'NONE',  ( 1.000000000000000000, 0.000000000000000000, 0.000000000000000000 ) ) ;
#4503=ORIENTED_EDGE ( 'NONE', *, *, #20547, .T. ) ;
#4507=VERTEX_POINT ( 'NONE', #17661 ) ;
#4508=VERTEX_POINT ( 'NONE', #20120 ) ;
#4513=ORIENTED_EDGE ( 'NONE', *, *, #21124, .F. ) ;
#4516=CARTESIAN_POINT ( 'NONE',  ( 25.16042852506077665, -18.28012134629603835, 1.000000000000000000 ) ) ;
#4520=AXIS2_PLACEMENT_3D ( 'NONE', #21780, #4110, #1784 ) ;
#4522=EDGE_CURVE ( 'NONE', #10325, #674, #7832, .T. ) ;
#4524=CIRCLE ( 'NONE', #22913, 0.5000000000000005551 ) ;
#4525=DIRECTION ( 'NONE',  ( 1.000000000000000000, 0.000000000000000000, 0.000000000000000000 ) ) ;
#4526=CARTESIAN_POINT ( 'NONE',  ( -10.08469938919458286, 29.41953157733104263, -6.500000000000000000 ) ) ;
#4530=EDGE_CURVE ( 'NONE', #4728, #15879, #22667, .T. ) ;
#4531=DIRECTION ( 'NONE',  ( 0.000000000000000000, 0.000000000000000000, 1.000000000000000000 ) ) ;
#4534=ADVANCED_FACE ( 'NONE', ( #12305 ), #16201, .T. ) ;
#4535=DIRECTION ( 'NONE',  ( 0.000000000000000000, -0.000000000000000000, 1.000000000000000000 ) ) ;
#4536=ORIENTED_EDGE ( 'NONE', *, *, #5627, .T. ) ;
#4538=DIRECTION ( 'NONE',  ( -0.000000000000000000, 0.000000000000000000, 1.000000000000000000 ) ) ;
#4541=DIRECTION ( 'NONE',  ( 0.000000000000000000, 0.000000000000000000, 1.000000000000000000 ) ) ;
#4546=ORIENTED_EDGE ( 'NONE', *, *, #1319, .F. ) ;
#4548=ORIENTED_EDGE ( 'NONE', *, *, #17695, .T. ) ;
#4549=CIRCLE ( 'NONE', #10755, 0.4999999999999999445 ) ;
#4551=( NAMED_UNIT ( * ) SI_UNIT ( $, .STERADIAN. ) SOLID_ANGLE_UNIT ( ) );
#4553=AXIS2_PLACEMENT_3D ( 'NONE', #22455, #18552, #12517 ) ;
#4560=CARTESIAN_POINT ( 'NONE',  ( -28.41604871112473418, -11.44867358849319849, -6.500000000000000000 ) ) ;
#4561=AXIS2_PLACEMENT_3D ( 'NONE', #17278, #7825, #3913 ) ;
#4563=EDGE_CURVE ( 'NONE', #5989, #20109, #6261, .T. ) ;
#4566=CARTESIAN_POINT ( 'NONE',  ( 0.000000000000000000, 0.000000000000000000, -6.500000000000000000 ) ) ;
#4570=VECTOR ( 'NONE', #1220, 1000.000000000000000 ) ;
#4574=DIRECTION ( 'NONE',  ( 0.000000000000000000, -0.000000000000000000, -1.000000000000000000 ) ) ;
#4578=LINE ( 'NONE', #4327, #13329 ) ;
#4580=EDGE_LOOP ( 'NONE', ( #3878, #13681, #18935, #1565 ) ) ;
#4581=CIRCLE ( 'NONE', #3947, 31.10000000000000142 ) ;
#4583=VERTEX_POINT ( 'NONE', #23786 ) ;
#4584=ORIENTED_EDGE ( 'NONE', *, *, #19209, .F. ) ;
#4588=CIRCLE ( 'NONE', #1, 0.5000000000000002220 ) ;
#4590=DIRECTION ( 'NONE',  ( -0.000000000000000000, 0.000000000000000000, 1.000000000000000000 ) ) ;
#4599=CARTESIAN_POINT ( 'NONE',  ( -19.43607991389006528, -24.27856662945486832, 1.000000000000000000 ) ) ;
#4602=ADVANCED_FACE ( 'NONE', ( #5874 ), #13989, .T. ) ;
#4603=CARTESIAN_POINT ( 'NONE',  ( 0.000000000000000000, 0.000000000000000000, -6.500000000000000000 ) ) ;
#4604=CIRCLE ( 'NONE', #7941, 31.10000000000000142 ) ;
#4611=CIRCLE ( 'NONE', #2522, 0.5000000000000001110 ) ;
#4613=VERTEX_POINT ( 'NONE', #8616 ) ;
#4619=ADVANCED_FACE ( 'NONE', ( #16866 ), #16343, .F. ) ;
#4620=CIRCLE ( 'NONE', #20927, 31.10000000000000142 ) ;
#4625=AXIS2_PLACEMENT_3D ( 'NONE', #8627, #14645, #17125 ) ;
#4626=AXIS2_PLACEMENT_3D ( 'NONE', #564, #24598, #2261 ) ;
#4627=MANIFOLD_SOLID_BREP ( 'CirPattern1', #5043 ) ;
#4631=CIRCLE ( 'NONE', #13411, 0.4999999999999998890 ) ;
#4634=DIRECTION ( 'NONE',  ( 1.000000000000000000, 0.000000000000000000, 0.000000000000000000 ) ) ;
#4638=CYLINDRICAL_SURFACE ( 'NONE', #491, 0.5000000000000004441 ) ;
#4642=CIRCLE ( 'NONE', #21764, 0.5000000000000003331 ) ;
#4643=ADVANCED_FACE ( 'NONE', ( #24697 ), #8882, .F. ) ;
#4652=EDGE_CURVE ( 'NONE', #22312, #6939, #25182, .T. ) ;
#4653=DIRECTION ( 'NONE',  ( 0.000000000000000000, 0.000000000000000000, 1.000000000000000000 ) ) ;
#4658=CIRCLE ( 'NONE', #21797, 0.5000000000000003331 ) ;
#4659=DIRECTION ( 'NONE',  ( 0.000000000000000000, 0.000000000000000000, 1.000000000000000000 ) ) ;
#4661=CIRCLE ( 'NONE', #19271, 0.5000000000000003331 ) ;
#4662=VECTOR ( 'NONE', #4469, 1000.000000000000000 ) ;
#4665=CIRCLE ( 'NONE', #25298, 0.4999999999999999445 ) ;
#4670=DIRECTION ( 'NONE',  ( -0.000000000000000000, -0.000000000000000000, 1.000000000000000000 ) ) ;
#4672=EDGE_CURVE ( 'NONE', #4507, #18169, #7222, .T. ) ;
#4675=DIRECTION ( 'NONE',  ( 0.000000000000000000, 0.000000000000000000, 1.000000000000000000 ) ) ;
#4677=CYLINDRICAL_SURFACE ( 'NONE', #12471, 0.5000000000000004441 ) ;
#4678=VERTEX_POINT ( 'NONE', #2462 ) ;
#4679=CIRCLE ( 'NONE', #21812, 31.10000000000000142 ) ;
#4682=LINE ( 'NONE', #634, #16730 ) ;
#4684=DIRECTION ( 'NONE',  ( 0.000000000000000000, 0.000000000000000000, 1.000000000000000000 ) ) ;
#4688=VERTEX_POINT ( 'NONE', #20772 ) ;
#4691=AXIS2_PLACEMENT_3D ( 'NONE', #18690, #4318, #14269 ) ;
#4692=EDGE_CURVE ( 'NONE', #23209, #16529, #5138, .T. ) ;
#4693=ORIENTED_EDGE ( 'NONE', *, *, #13161, .T. ) ;
#4695=ORIENTED_EDGE ( 'NONE', *, *, #15699, .F. ) ;
#4696=AXIS2_PLACEMENT_3D ( 'NONE', #1775, #25566, #17722 ) ;
#4698=EDGE_CURVE ( 'NONE', #7162, #14796, #24441, .T. ) ;
#4699=DIRECTION ( 'NONE',  ( -0.000000000000000000, -0.000000000000000000, 1.000000000000000000 ) ) ;
#4700=AXIS2_PLACEMENT_3D ( 'NONE', #18533, #226, #14353 ) ;
#4704=EDGE_CURVE ( 'NONE', #22201, #5837, #13488, .T. ) ;
#4705=VECTOR ( 'NONE', #3620, 1000.000000000000000 ) ;
#4711=CARTESIAN_POINT ( 'NONE',  ( 19.43607991388988765, 24.27856662945500688, -2.750000000000000000 ) ) ;
#4712=CARTESIAN_POINT ( 'NONE',  ( -17.08421000182795879, -25.98730014090424234, -6.500000000000000000 ) ) ;
#4720=DIRECTION ( 'NONE',  ( 1.000000000000000000, 0.000000000000000000, 0.000000000000000000 ) ) ;
#4721=CARTESIAN_POINT ( 'NONE',  ( -29.62293631110035363, 7.734255490827311341, -6.500000000000000000 ) ) ;
#4725=DIRECTION ( 'NONE',  ( 1.000000000000000000, 0.000000000000000000, 0.000000000000000000 ) ) ;
#4726=ORIENTED_EDGE ( 'NONE', *, *, #4522, .T. ) ;
#4727=CIRCLE ( 'NONE', #12217, 31.10000000000000142 ) ;
#4728=VERTEX_POINT ( 'NONE', #18428 ) ;
#4729=ORIENTED_EDGE ( 'NONE', *, *, #10657, .F. ) ;
#4731=VERTEX_POINT ( 'NONE', #20645 ) ;
#4733=VECTOR ( 'NONE', #21060, 1000.000000000000000 ) ;
#4734=ORIENTED_EDGE ( 'NONE', *, *, #362, .F. ) ;
#4735=EDGE_CURVE ( 'NONE', #19594, #15159, #18564, .T. ) ;
#4736=DIRECTION ( 'NONE',  ( 1.000000000000000000, 0.000000000000000000, 0.000000000000000000 ) ) ;
#4739=EDGE_CURVE ( 'NONE', #17107, #4508, #16825, .T. ) ;
#4741=DIRECTION ( 'NONE',  ( -0.000000000000000000, -0.000000000000000000, 1.000000000000000000 ) ) ;
#4743=ADVANCED_FACE ( 'NONE', ( #25338 ), #3364, .T. ) ;
#4744=DIRECTION ( 'NONE',  ( -0.000000000000000000, 0.000000000000000000, 1.000000000000000000 ) ) ;
#4749=DIRECTION ( 'NONE',  ( 1.000000000000000000, 0.000000000000000000, 0.000000000000000000 ) ) ;
#4752=DIRECTION ( 'NONE',  ( 0.000000000000000000, 0.000000000000000000, 1.000000000000000000 ) ) ;
#4754=CYLINDRICAL_SURFACE ( 'NONE', #13284, 0.5000000000000004441 ) ;
#4755=EDGE_CURVE ( 'NONE', #9389, #4038, #4727, .T. ) ;
#4760=ORIENTED_EDGE ( 'NONE', *, *, #19981, .F. ) ;
#4761=CYLINDRICAL_SURFACE ( 'NONE', #9192, 0.5000000000000004441 ) ;
#4762=ORIENTED_EDGE ( 'NONE', *, *, #13106, .T. ) ;
#4766=ORIENTED_EDGE ( 'NONE', *, *, #16566, .T. ) ;
#4770=DIRECTION ( 'NONE',  ( 0.000000000000000000, 0.000000000000000000, 1.000000000000000000 ) ) ;
#4771=DIRECTION ( 'NONE',  ( 0.000000000000000000, 0.000000000000000000, 1.000000000000000000 ) ) ;
#4777=DIRECTION ( 'NONE',  ( 0.9822872507286884991, -0.1873813145857256834, 0.000000000000000000 ) ) ;
#4779=DIRECTION ( 'NONE',  ( 1.000000000000000000, 0.000000000000000000, 0.000000000000000000 ) ) ;
#4785=ORIENTED_EDGE ( 'NONE', *, *, #4423, .F. ) ;
#4800=CARTESIAN_POINT ( 'NONE',  ( -29.99470236596038220, -8.217531866530892515, 1.000000000000000000 ) ) ;
#4801=FACE_OUTER_BOUND ( 'NONE', #9566, .T. ) ;
#4806=DIRECTION ( 'NONE',  ( -0.000000000000000000, 0.000000000000000000, 1.000000000000000000 ) ) ;
#4807=EDGE_CURVE ( 'NONE', #22201, #23568, #15665, .T. ) ;
#4809=DIRECTION ( 'NONE',  ( -0.000000000000000000, -0.000000000000000000, 1.000000000000000000 ) ) ;
#4811=CARTESIAN_POINT ( 'NONE',  ( 24.27856662945494293, -19.43607991388997291, 1.000000000000000000 ) ) ;
#4812=VERTEX_POINT ( 'NONE', #23506 ) ;
#4813=DIRECTION ( 'NONE',  ( 0.000000000000000000, 0.000000000000000000, 1.000000000000000000 ) ) ;
#4816=VERTEX_POINT ( 'NONE', #19946 ) ;
#4820=EDGE_LOOP ( 'NONE', ( #25713, #19268, #14049, #4450 ) ) ;
#4821=ORIENTED_EDGE ( 'NONE', *, *, #6192, .T. ) ;
#4828=EDGE_CURVE ( 'NONE', #17442, #24369, #22045, .T. ) ;
#4829=DIRECTION ( 'NONE',  ( 0.000000000000000000, 0.000000000000000000, 1.000000000000000000 ) ) ;
#4831=AXIS2_PLACEMENT_3D ( 'NONE', #11942, #24239, #14442 ) ;
#4840=DIRECTION ( 'NONE',  ( -0.000000000000000000, -0.000000000000000000, 1.000000000000000000 ) ) ;
#4841=CARTESIAN_POINT ( 'NONE',  ( -31.00322564728516639, -2.451530025008796798, 1.000000000000000000 ) ) ;
#4843=EDGE_CURVE ( 'NONE', #19911, #19004, #5155, .T. ) ;
#4845=CARTESIAN_POINT ( 'NONE',  ( 14.98253926456319007, -27.25313774936425304, -6.500000000000000000 ) ) ;
#4846=ORIENTED_EDGE ( 'NONE', *, *, #3638, .T. ) ;
#4847=ORIENTED_EDGE ( 'NONE', *, *, #3569, .F. ) ;
#4851=ORIENTED_EDGE ( 'NONE', *, *, #239, .F. ) ;
#4852=DIRECTION ( 'NONE',  ( 0.000000000000000000, 0.000000000000000000, 1.000000000000000000 ) ) ;
#4853=VERTEX_POINT ( 'NONE', #9889 ) ;
#4863=DIRECTION ( 'NONE',  ( -0.8090169943749417891, 0.5877852522924807976, 0.000000000000000000 ) ) ;
#4864=CARTESIAN_POINT ( 'NONE',  ( 9.610428525060889626, 29.57785765677927614, 1.000000000000000000 ) ) ;
#4870=EDGE_CURVE ( 'NONE', #383, #5108, #25721, .T. ) ;
#4871=ORIENTED_EDGE ( 'NONE', *, *, #14360, .F. ) ;
#4876=ORIENTED_EDGE ( 'NONE', *, *, #17614, .F. ) ;
#4878=ORIENTED_EDGE ( 'NONE', *, *, #10953, .F. ) ;
#4879=CARTESIAN_POINT ( 'NONE',  ( -16.23990935651680090, 26.52310962334767908, -6.500000000000000000 ) ) ;
#4881=ORIENTED_EDGE ( 'NONE', *, *, #16934, .F. ) ;
#4882=DIRECTION ( 'NONE',  ( 0.5358267949789962126, -0.8443279255020154084, 0.000000000000000000 ) ) ;
#4884=DIRECTION ( 'NONE',  ( 0.8090169943749532244, 0.5877852522924652545, 0.000000000000000000 ) ) ;
#4885=DIRECTION ( 'NONE',  ( 0.000000000000000000, 0.000000000000000000, 1.000000000000000000 ) ) ;
#4888=LINE ( 'NONE', #11419, #5849 ) ;
#4890=LINE ( 'NONE', #22297, #2172 ) ;
#4891=DIRECTION ( 'NONE',  ( 0.000000000000000000, 0.000000000000000000, 1.000000000000000000 ) ) ;
#4897=EDGE_CURVE ( 'NONE', #5989, #9673, #8077, .T. ) ;
#4898=DIRECTION ( 'NONE',  ( -0.000000000000000000, -0.000000000000000000, 1.000000000000000000 ) ) ;
#4902=ORIENTED_EDGE ( 'NONE', *, *, #11344, .T. ) ;
#4903=ORIENTED_EDGE ( 'NONE', *, *, #9378, .F. ) ;
#4906=ORIENTED_EDGE ( 'NONE', *, *, #16902, .F. ) ;
#4908=LINE ( 'NONE', #8978, #21807 ) ;
#4910=DIRECTION ( 'NONE',  ( 0.000000000000000000, 0.000000000000000000, 1.000000000000000000 ) ) ;
#4916=CARTESIAN_POINT ( 'NONE',  ( -23.64116323484252291, -20.20656826142258211, 1.000000000000000000 ) ) ;
#4918=CARTESIAN_POINT ( 'NONE',  ( 24.27856662945494293, -19.43607991388997291, -6.500000000000000000 ) ) ;
#4923=DIRECTION ( 'NONE',  ( 1.000000000000000000, 0.000000000000000000, 0.000000000000000000 ) ) ;
#4925=DIRECTION ( 'NONE',  ( 0.000000000000000000, 0.000000000000000000, 1.000000000000000000 ) ) ;
#4928=CIRCLE ( 'NONE', #10776, 0.4999999999999983902 ) ;
#4933=DIRECTION ( 'NONE',  ( -0.5877852522924652545, 0.8090169943749532244, 0.000000000000000000 ) ) ;
#4935=LINE ( 'NONE', #8729, #18745 ) ;
#4937=VERTEX_POINT ( 'NONE', #9603 ) ;
#4939=EDGE_LOOP ( 'NONE', ( #11298, #8517, #13447, #17687 ) ) ;
#4940=VERTEX_POINT ( 'NONE', #23716 ) ;
#4943=VECTOR ( 'NONE', #20295, 1000.000000000000000 ) ;
#4944=CARTESIAN_POINT ( 'NONE',  ( 0.000000000000000000, 0.000000000000000000, -6.500000000000000000 ) ) ;
#4946=CIRCLE ( 'NONE', #8291, 31.10000000000000142 ) ;
#4947=CIRCLE ( 'NONE', #25000, 0.4999999999999991673 ) ;
#4950=CARTESIAN_POINT ( 'NONE',  ( 19.43607991388981304, -24.27856662945506727, 1.000000000000000000 ) ) ;
#4952=LINE ( 'NONE', #12934, #21750 ) ;
#4953=CARTESIAN_POINT ( 'NONE',  ( -26.52310962334728828, 16.23990935651745460, 1.000000000000000000 ) ) ;
#4960=CARTESIAN_POINT ( 'NONE',  ( 27.92360179968377309, 13.69242354489143842, -2.750000000000000000 ) ) ;
#4963=LINE ( 'NONE', #5225, #24573 ) ;
#4964=VECTOR ( 'NONE', #11221, 1000.000000000000000 ) ;
#4965=DIRECTION ( 'NONE',  ( 0.000000000000000000, 0.000000000000000000, 1.000000000000000000 ) ) ;
#4968=VERTEX_POINT ( 'NONE', #11829 ) ;
#4969=DIRECTION ( 'NONE',  ( -0.000000000000000000, -0.000000000000000000, 1.000000000000000000 ) ) ;
#4970=CYLINDRICAL_SURFACE ( 'NONE', #5408, 0.5000000000000004441 ) ;
#4971=ORIENTED_EDGE ( 'NONE', *, *, #25125, .F. ) ;
#4973=ADVANCED_FACE ( 'NONE', ( #1897 ), #11560, .T. ) ;
#4976=ORIENTED_EDGE ( 'NONE', *, *, #11344, .F. ) ;
#4980=ADVANCED_FACE ( 'NONE', ( #3980 ), #15753, .F. ) ;
#4983=CARTESIAN_POINT ( 'NONE',  ( 0.000000000000000000, 0.000000000000000000, -6.500000000000000000 ) ) ;
#4988=EDGE_CURVE ( 'NONE', #19150, #12673, #25199, .T. ) ;
#4990=DIRECTION ( 'NONE',  ( 0.000000000000000000, 0.000000000000000000, 1.000000000000000000 ) ) ;
#4991=CIRCLE ( 'NONE', #2079, 0.5000000000000001110 ) ;
#4993=CYLINDRICAL_SURFACE ( 'NONE', #8358, 0.5000000000000004441 ) ;
#4995=CARTESIAN_POINT ( 'NONE',  ( -23.46296185032722548, -19.82388608118403539, -6.500000000000000000 ) ) ;
#5003=AXIS2_PLACEMENT_3D ( 'NONE', #232, #13965, #23760 ) ;
#5004=ORIENTED_EDGE ( 'NONE', *, *, #6792, .T. ) ;
#5008=ORIENTED_EDGE ( 'NONE', *, *, #16401, .F. ) ;
#5009=DIRECTION ( 'NONE',  ( -0.000000000000000000, -0.000000000000000000, 1.000000000000000000 ) ) ;
#5010=AXIS2_PLACEMENT_3D ( 'NONE', #8397, #16387, #3032 ) ;
#5011=CIRCLE ( 'NONE', #20432, 0.4999999999999998890 ) ;
#5016=FACE_OUTER_BOUND ( 'NONE', #14044, .T. ) ;
#5017=CARTESIAN_POINT ( 'NONE',  ( 7.734255490826784651, -30.12293631110048153, -6.500000000000000000 ) ) ;
#5022=ADVANCED_FACE ( 'NONE', ( #21509 ), #1774, .T. ) ;
#5023=CYLINDRICAL_SURFACE ( 'NONE', #19220, 31.10000000000000142 ) ;
#5031=CARTESIAN_POINT ( 'NONE',  ( 0.000000000000000000, 0.000000000000000000, 1.000000000000000000 ) ) ;
#5035=CYLINDRICAL_SURFACE ( 'NONE', #8275, 27.10000000000000142 ) ;
#5040=VECTOR ( 'NONE', #16517, 1000.000000000000000 ) ;
#5041=FACE_OUTER_BOUND ( 'NONE', #1236, .T. ) ;
#5042=ORIENTED_EDGE ( 'NONE', *, *, #23060, .T. ) ;
#5043=CLOSED_SHELL ( 'NONE', ( #18116, #11158, #25191, #1660, #25034, #8100, #19119, #5623, #10720, #24784, #12328, #16836, #6459, #2368, #1413, #20223, #10909, #15518, #12945, #13509, #13820, #19302, #16404, #4643, #6391, #22772, #24053, #23722, #8067, #4619, #15228, #10982, #21222, #3550, #5298, #25626, #1763, #5174, #5715, #14941, #22965, #11527, #22401, #16246, #18348, #13532, #18635, #15445, #8262, #17929, #8202, #23217, #17621, #24081, #18462, #17306, #20726, #11301, #20067, #17665, #15089, #4973, #7716, #25590, #456, #12540, #21190, #19855, #14841, #24192, #100, #679, #9935, #21455, #23886, #21314, #4243, #1282, #1539, #9431, #4460, #9797, #3887, #18134, #15371, #19192, #23963, #16731, #25151, #8046, #25237, #3200, #4534, #25086, #2697, #8499, #10471, #10960, #6092, #7467, #11741, #2112, #21458, #4280, #5056, #14112, #19326, #244, #16631, #4602, #25192, #17373, #15846, #22146, #19384, #21557, #3622, #22826, #4063, #7551, #16669, #7082, #25664, #944, #10570, #20719, #9652, #17118, #25427, #8463, #23511, #992, #22838, #890, #10404, #4396, #5022, #4015, #2523, #19782, #9532, #24831, #20215, #16066, #13765, #18589, #23838, #4743, #12402, #17577, #2871, #15810, #5366, #1032, #6746, #25787, #2190, #685, #5490, #21661, #736, #17113, #6646, #8236, #18054, #2471, #6967, #6128, #15737, #3486, #11386, #16038, #18598, #22292, #1102, #15559, #10159, #6466, #16601, #20413, #18019, #13025, #5756, #6429, #13489, #10244, #6488, #8055, #5414, #20473, #8132, #6365, #24023, #17667, #9927, #20376, #4980, #22670, #14176, #17193, #6944, #23951, #16508, #24394, #13731, #12012, #7391, #14602, #6991, #351, #10188, #9496, #3503, #17752, #24277, #22651, #1444, #8540, #23691, #7619, #894, #17699, #11046, #4001, #12283, #493, #13292, #12707, #12353, #12899, #22541, #15097, #12681, #18268, #14302, #9065, #1336, #20057, #7687, #8524, #20868, #16840, #17154, #25368, #14898, #21395, #13350, #10347, #8571, #22281, #1038, #22497, #25758, #15406, #11757, #13926 ) ) ;
#5047=AXIS2_PLACEMENT_3D ( 'NONE', #10443, #18437, #533 ) ;
#5052=AXIS2_PLACEMENT_3D ( 'NONE', #24077, #9831, #4200 ) ;
#5053=DIRECTION ( 'NONE',  ( 0.000000000000000000, -0.000000000000000000, 1.000000000000000000 ) ) ;
#5056=ADVANCED_FACE ( 'NONE', ( #22542 ), #16414, .T. ) ;
#5058=CIRCLE ( 'NONE', #19646, 0.5000000000000001110 ) ;
#5059=LINE ( 'NONE', #9368, #906 ) ;
#5061=CARTESIAN_POINT ( 'NONE',  ( 16.23990935651709222, -26.52310962334749433, 1.000000000000000000 ) ) ;
#5064=CARTESIAN_POINT ( 'NONE',  ( -16.66421332384646448, 26.25859848311288403, -6.500000000000000000 ) ) ;
#5066=AXIS2_PLACEMENT_3D ( 'NONE', #9483, #8984, #11568 ) ;
#5067=CARTESIAN_POINT ( 'NONE',  ( -26.25859848311247902, 16.66421332384710752, 1.000000000000000000 ) ) ;
#5070=ORIENTED_EDGE ( 'NONE', *, *, #11892, .T. ) ;
#5071=CARTESIAN_POINT ( 'NONE',  ( -11.44867358849371541, -28.91604871112453168, 1.000000000000000000 ) ) ;
#5080=ORIENTED_EDGE ( 'NONE', *, *, #23723, .T. ) ;
#5081=ORIENTED_EDGE ( 'NONE', *, *, #25543, .F. ) ;
#5083=VECTOR ( 'NONE', #19050, 1000.000000000000000 ) ;
#5085=AXIS2_PLACEMENT_3D ( 'NONE', #10028, #12121, #11866 ) ;
#5095=DIRECTION ( 'NONE',  ( -0.000000000000000000, -0.000000000000000000, 1.000000000000000000 ) ) ;
#5097=FACE_OUTER_BOUND ( 'NONE', #762, .T. ) ;
#5101=AXIS2_PLACEMENT_3D ( 'NONE', #21971, #9812, #4046 ) ;
#5106=DIRECTION ( 'NONE',  ( 0.000000000000000000, -0.000000000000000000, -1.000000000000000000 ) ) ;
#5108=VERTEX_POINT ( 'NONE', #12738 ) ;
#5110=DIRECTION ( 'NONE',  ( 1.000000000000000000, 0.000000000000000000, 0.000000000000000000 ) ) ;
#5111=ORIENTED_EDGE ( 'NONE', *, *, #13529, .F. ) ;
#5113=AXIS2_PLACEMENT_3D ( 'NONE', #6363, #14082, #22047 ) ;
#5115=VERTEX_POINT ( 'NONE', #4365 ) ;
#5116=ORIENTED_EDGE ( 'NONE', *, *, #390, .F. ) ;
#5117=ORIENTED_EDGE ( 'NONE', *, *, #21515, .T. ) ;
#5120=LINE ( 'NONE', #3920, #5264 ) ;
#5121=CIRCLE ( 'NONE', #20567, 31.10000000000000142 ) ;
#5123=CIRCLE ( 'NONE', #19725, 31.10000000000000142 ) ;
#5124=AXIS2_PLACEMENT_3D ( 'NONE', #6023, #25514, #15976 ) ;
#5138=CIRCLE ( 'NONE', #24753, 0.4999999999999998335 ) ;
#5139=CARTESIAN_POINT ( 'NONE',  ( 17.08421000182778116, 25.98730014090436313, -6.500000000000000000 ) ) ;
#5141=ORIENTED_EDGE ( 'NONE', *, *, #11265, .F. ) ;
#5143=CIRCLE ( 'NONE', #22252, 31.10000000000000142 ) ;
#5144=ORIENTED_EDGE ( 'NONE', *, *, #13139, .T. ) ;
#5145=DIRECTION ( 'NONE',  ( 0.000000000000000000, 0.000000000000000000, 1.000000000000000000 ) ) ;
#5146=ORIENTED_EDGE ( 'NONE', *, *, #24265, .T. ) ;
#5148=VERTEX_POINT ( 'NONE', #10237 ) ;
#5150=CIRCLE ( 'NONE', #23508, 31.10000000000000142 ) ;
#5155=CIRCLE ( 'NONE', #14742, 0.5000000000000000000 ) ;
#5156=DIRECTION ( 'NONE',  ( 1.000000000000000000, 0.000000000000000000, 0.000000000000000000 ) ) ;
#5165=CIRCLE ( 'NONE', #7254, 31.10000000000000142 ) ;
#5166=VERTEX_POINT ( 'NONE', #20434 ) ;
#5170=CIRCLE ( 'NONE', #12250, 0.5000000000000002220 ) ;
#5171=CARTESIAN_POINT ( 'NONE',  ( -14.98253926456298579, 27.25313774936435962, -6.500000000000000000 ) ) ;
#5174=ADVANCED_FACE ( 'NONE', ( #22682 ), #8167, .F. ) ;
#5175=ORIENTED_EDGE ( 'NONE', *, *, #2268, .F. ) ;
#5176=ORIENTED_EDGE ( 'NONE', *, *, #1162, .F. ) ;
#5177=CARTESIAN_POINT ( 'NONE',  ( -27.25313774936430633, -14.98253926456308172, -6.500000000000000000 ) ) ;
#5186=CARTESIAN_POINT ( 'NONE',  ( 30.85476721088025442, -3.897863563849982782, -6.500000000000000000 ) ) ;
#5197=CARTESIAN_POINT ( 'NONE',  ( -11.44867358849309547, 28.91604871112477326, -6.500000000000000000 ) ) ;
#5206=EDGE_CURVE ( 'NONE', #25291, #24730, #1810, .T. ) ;
#5210=ORIENTED_EDGE ( 'NONE', *, *, #22674, .T. ) ;
#5221=CYLINDRICAL_SURFACE ( 'NONE', #6364, 0.5000000000000004441 ) ;
#5222=DIRECTION ( 'NONE',  ( 0.4257792915650712717, -0.9048270524660203540, 0.000000000000000000 ) ) ;
#5224=CARTESIAN_POINT ( 'NONE',  ( -27.25313774936430633, -14.98253926456308172, -6.500000000000000000 ) ) ;
#5225=CARTESIAN_POINT ( 'NONE',  ( -10.98232076577180649, 29.09636799667095630, -2.750000000000000000 ) ) ;
#5227=EDGE_CURVE ( 'NONE', #21732, #7703, #11826, .T. ) ;
#5229=EDGE_LOOP ( 'NONE', ( #23264, #6089, #12306, #16444 ) ) ;
#5231=DIRECTION ( 'NONE',  ( 0.6374239897486886353, -0.7705132427757902525, 0.000000000000000000 ) ) ;
#5232=ORIENTED_EDGE ( 'NONE', *, *, #18103, .F. ) ;
#5235=ORIENTED_EDGE ( 'NONE', *, *, #24881, .F. ) ;
#5236=ORIENTED_EDGE ( 'NONE', *, *, #11312, .F. ) ;
#5239=DIRECTION ( 'NONE',  ( 0.000000000000000000, 0.000000000000000000, 1.000000000000000000 ) ) ;
#5241=EDGE_CURVE ( 'NONE', #20109, #6572, #8913, .T. ) ;
#5249=DIRECTION ( 'NONE',  ( 0.000000000000000000, -0.000000000000000000, 1.000000000000000000 ) ) ;
#5255=CYLINDRICAL_SURFACE ( 'NONE', #17879, 0.5000000000000004441 ) ;
#5257=ORIENTED_EDGE ( 'NONE', *, *, #9458, .T. ) ;
#5263=VERTEX_POINT ( 'NONE', #11142 ) ;
#5264=VECTOR ( 'NONE', #9679, 1000.000000000000000 ) ;
#5265=CARTESIAN_POINT ( 'NONE',  ( 9.610428525060671134, -29.57785765677934009, -6.500000000000000000 ) ) ;
#5268=EDGE_CURVE ( 'NONE', #18492, #15884, #23510, .T. ) ;
#5271=DIRECTION ( 'NONE',  ( -0.000000000000000000, -0.000000000000000000, 1.000000000000000000 ) ) ;
#5274=DIRECTION ( 'NONE',  ( 0.1873813145857330109, 0.9822872507286871668, 0.000000000000000000 ) ) ;
#5276=LINE ( 'NONE', #11281, #7942 ) ;
#5282=ORIENTED_EDGE ( 'NONE', *, *, #11200, .T. ) ;
#5285=VERTEX_POINT ( 'NONE', #15574 ) ;
#5286=CARTESIAN_POINT ( 'NONE',  ( -30.60000000000000142, 3.257552089140643357E-13, -6.500000000000000000 ) ) ;
#5289=ORIENTED_EDGE ( 'NONE', *, *, #15336, .T. ) ;
#5290=VERTEX_POINT ( 'NONE', #21098 ) ;
#5291=CARTESIAN_POINT ( 'NONE',  ( 0.000000000000000000, 0.000000000000000000, -6.500000000000000000 ) ) ;
#5298=ADVANCED_FACE ( 'NONE', ( #1213 ), #18883, .F. ) ;
#5301=EDGE_CURVE ( 'NONE', #9082, #16618, #18517, .T. ) ;
#5311=DIRECTION ( 'NONE',  ( 0.8443279255020205154, 0.5358267949789882190, 0.000000000000000000 ) ) ;
#5321=VERTEX_POINT ( 'NONE', #23542 ) ;
#5325=ORIENTED_EDGE ( 'NONE', *, *, #4522, .F. ) ;
#5326=ORIENTED_EDGE ( 'NONE', *, *, #2230, .F. ) ;
#5330=EDGE_CURVE ( 'NONE', #27, #7696, #7241, .T. ) ;
#5331=AXIS2_PLACEMENT_3D ( 'NONE', #15487, #4891, #8961 ) ;
#5333=PRESENTATION_STYLE_ASSIGNMENT (( #17631 ) ) ;
#5335=CARTESIAN_POINT ( 'NONE',  ( 0.000000000000000000, 0.000000000000000000, -6.500000000000000000 ) ) ;
#5336=EDGE_CURVE ( 'NONE', #4455, #12921, #13606, .T. ) ;
#5337=CARTESIAN_POINT ( 'NONE',  ( 26.52310962334750855, 16.23990935651707801, -2.750000000000000000 ) ) ;
#5339=CARTESIAN_POINT ( 'NONE',  ( 0.000000000000000000, 0.000000000000000000, -6.500000000000000000 ) ) ;
#5341=DIRECTION ( 'NONE',  ( -0.000000000000000000, 0.000000000000000000, 1.000000000000000000 ) ) ;
#5352=ORIENTED_EDGE ( 'NONE', *, *, #4988, .T. ) ;
#5354=AXIS2_PLACEMENT_3D ( 'NONE', #15715, #7992, #5641 ) ;
#5356=ORIENTED_EDGE ( 'NONE', *, *, #7759, .T. ) ;
#5357=ORIENTED_EDGE ( 'NONE', *, *, #10784, .T. ) ;
#5358=CARTESIAN_POINT ( 'NONE',  ( 0.000000000000000000, 0.000000000000000000, 1.000000000000000000 ) ) ;
#5366=ADVANCED_FACE ( 'NONE', ( #831 ), #2788, .F. ) ;
#5387=VERTEX_POINT ( 'NONE', #19005 ) ;
#5390=EDGE_LOOP ( 'NONE', ( #22334, #6903, #8523, #24492 ) ) ;
#5392=CARTESIAN_POINT ( 'NONE',  ( 5.827558883616049457, 30.54913349766221842, -6.500000000000000000 ) ) ;
#5395=AXIS2_PLACEMENT_3D ( 'NONE', #8906, #14788, #8633 ) ;
#5397=DIRECTION ( 'NONE',  ( 0.000000000000000000, 0.000000000000000000, 1.000000000000000000 ) ) ;
#5399=EDGE_CURVE ( 'NONE', #17170, #4613, #14356, .T. ) ;
#5401=DIRECTION ( 'NONE',  ( -0.000000000000000000, -0.000000000000000000, 1.000000000000000000 ) ) ;
#5408=AXIS2_PLACEMENT_3D ( 'NONE', #18969, #19086, #5110 ) ;
#5409=VERTEX_POINT ( 'NONE', #12282 ) ;
#5412=VECTOR ( 'NONE', #9336, 1000.000000000000000 ) ;
#5414=ADVANCED_FACE ( 'NONE', ( #18296 ), #7835, .F. ) ;
#5415=ORIENTED_EDGE ( 'NONE', *, *, #9720, .T. ) ;
#5420=ORIENTED_EDGE ( 'NONE', *, *, #18266, .F. ) ;
#5421=ORIENTED_EDGE ( 'NONE', *, *, #25545, .T. ) ;
#5423=CARTESIAN_POINT ( 'NONE',  ( -12.78762572734017589, 28.34936733434218681, -2.750000000000000000 ) ) ;
#5424=AXIS2_PLACEMENT_3D ( 'NONE', #16226, #3671, #11649 ) ;
#5425=ORIENTED_EDGE ( 'NONE', *, *, #8327, .F. ) ;
#5428=AXIS2_PLACEMENT_3D ( 'NONE', #14934, #16777, #25132 ) ;
#5429=DIRECTION ( 'NONE',  ( 1.000000000000000000, 0.000000000000000000, 0.000000000000000000 ) ) ;
#5433=DIRECTION ( 'NONE',  ( -0.000000000000000000, -0.000000000000000000, 1.000000000000000000 ) ) ;
#5443=CYLINDRICAL_SURFACE ( 'NONE', #379, 31.10000000000000142 ) ;
#5445=LINE ( 'NONE', #13676, #1705 ) ;
#5451=ORIENTED_EDGE ( 'NONE', *, *, #8498, .F. ) ;
#5457=ORIENTED_EDGE ( 'NONE', *, *, #3624, .T. ) ;
#5462=AXIS2_PLACEMENT_3D ( 'NONE', #18661, #4675, #8596 ) ;
#5464=EDGE_CURVE ( 'NONE', #2244, #1666, #23131, .T. ) ;
#5466=AXIS2_PLACEMENT_3D ( 'NONE', #25473, #21295, #7307 ) ;
#5470=DIRECTION ( 'NONE',  ( -0.000000000000000000, 0.000000000000000000, 1.000000000000000000 ) ) ;
#5471=CARTESIAN_POINT ( 'NONE',  ( -30.04913349766215802, 5.827558883616378083, 1.000000000000000000 ) ) ;
#5473=ORIENTED_EDGE ( 'NONE', *, *, #19553, .T. ) ;
#5475=DIRECTION ( 'NONE',  ( 0.000000000000000000, 0.000000000000000000, -1.000000000000000000 ) ) ;
#5478=EDGE_CURVE ( 'NONE', #23155, #20629, #13939, .T. ) ;
#5479=AXIS2_PLACEMENT_3D ( 'NONE', #1632, #5682, #13933 ) ;
#5482=EDGE_LOOP ( 'NONE', ( #8971, #21408, #11403, #25710 ) ) ;
#5483=DIRECTION ( 'NONE',  ( 0.000000000000000000, 0.000000000000000000, 1.000000000000000000 ) ) ;
#5490=ADVANCED_FACE ( 'NONE', ( #16987 ), #20647, .F. ) ;
#5491=ORIENTED_EDGE ( 'NONE', *, *, #14403, .T. ) ;
#5492=DIRECTION ( 'NONE',  ( 0.000000000000000000, 0.000000000000000000, 1.000000000000000000 ) ) ;
#5493=AXIS2_PLACEMENT_3D ( 'NONE', #21398, #25057, #16960 ) ;
#5494=DIRECTION ( 'NONE',  ( 1.000000000000000000, 0.000000000000000000, -0.000000000000000000 ) ) ;
#5495=DIRECTION ( 'NONE',  ( 0.000000000000000000, 0.000000000000000000, 1.000000000000000000 ) ) ;
#5500=CARTESIAN_POINT ( 'NONE',  ( 30.45149776762725224, -6.317933499823547017, -2.750000000000000000 ) ) ;
#5501=CIRCLE ( 'NONE', #14293, 0.5000000000000002220 ) ;
#5503=AXIS2_PLACEMENT_3D ( 'NONE', #4864, #11128, #19106 ) ;
#5505=CARTESIAN_POINT ( 'NONE',  ( -22.32573188046898238, 21.65113613650357749, 1.000000000000000000 ) ) ;
#5508=CARTESIAN_POINT ( 'NONE',  ( -5.335677986744467027, 30.63887302793251877, 1.000000000000000000 ) ) ;
#5515=CARTESIAN_POINT ( 'NONE',  ( 25.45105997952925136, 17.87326343783933780, -2.750000000000000000 ) ) ;
#5516=ORIENTED_EDGE ( 'NONE', *, *, #14033, .T. ) ;
#5517=CARTESIAN_POINT ( 'NONE',  ( 1.952785157361650370, 31.03863125411924528, -6.500000000000000000 ) ) ;
#5519=CIRCLE ( 'NONE', #15987, 0.5000000000000002220 ) ;
#5520=ORIENTED_EDGE ( 'NONE', *, *, #23366, .T. ) ;
#5521=DIRECTION ( 'NONE',  ( 1.000000000000000000, 0.000000000000000000, 0.000000000000000000 ) ) ;
#5525=EDGE_CURVE ( 'NONE', #24045, #1951, #12693, .T. ) ;
#5530=VERTEX_POINT ( 'NONE', #20370 ) ;
#5531=VECTOR ( 'NONE', #11693, 1000.000000000000000 ) ;
#5535=CIRCLE ( 'NONE', #23070, 31.10000000000000142 ) ;
#5540=AXIS2_PLACEMENT_3D ( 'NONE', #6642, #15396, #21282 ) ;
#5544=DIRECTION ( 'NONE',  ( 1.000000000000000000, 0.000000000000000000, 0.000000000000000000 ) ) ;
#5545=ORIENTED_EDGE ( 'NONE', *, *, #11555, .T. ) ;
#5549=DIRECTION ( 'NONE',  ( 0.000000000000000000, -0.000000000000000000, 1.000000000000000000 ) ) ;
#5550=AXIS2_PLACEMENT_3D ( 'NONE', #3299, #1873, #25783 ) ;
#5551=EDGE_CURVE ( 'NONE', #24860, #13686, #19362, .T. ) ;
#5554=ORIENTED_EDGE ( 'NONE', *, *, #7444, .F. ) ;
#5555=ORIENTED_EDGE ( 'NONE', *, *, #18400, .T. ) ;
#5557=AXIS2_PLACEMENT_3D ( 'NONE', #12605, #2670, #24767 ) ;
#5569=DIRECTION ( 'NONE',  ( -0.9297764858882481276, 0.3681245526846864125, 0.000000000000000000 ) ) ;
#5570=DIRECTION ( 'NONE',  ( 0.000000000000000000, -0.000000000000000000, 1.000000000000000000 ) ) ;
#5576=LINE ( 'NONE', #9622, #24714 ) ;
#5578=DIRECTION ( 'NONE',  ( 1.000000000000000000, 0.000000000000000000, 0.000000000000000000 ) ) ;
#5595=AXIS2_PLACEMENT_3D ( 'NONE', #23338, #25310, #23101 ) ;
#5599=FILL_AREA_STYLE ('',( #19571 ) ) ;
#5602=CYLINDRICAL_SURFACE ( 'NONE', #16774, 0.5000000000000004441 ) ;
#5608=DIRECTION ( 'NONE',  ( -0.1873813145857119722, 0.9822872507286911636, 0.000000000000000000 ) ) ;
#5614=LINE ( 'NONE', #1694, #7938 ) ;
#5616=VERTEX_POINT ( 'NONE', #16869 ) ;
#5617=EDGE_LOOP ( 'NONE', ( #10086, #20543, #3451, #1447 ) ) ;
#5620=EDGE_LOOP ( 'NONE', ( #18203, #5939, #5326, #19028 ) ) ;
#5623=ADVANCED_FACE ( 'NONE', ( #24834 ), #18948, .F. ) ;
#5626=FACE_OUTER_BOUND ( 'NONE', #3399, .T. ) ;
#5627=EDGE_CURVE ( 'NONE', #19467, #23600, #1033, .T. ) ;
#5630=EDGE_CURVE ( 'NONE', #1683, #13534, #1540, .T. ) ;
#5633=CARTESIAN_POINT ( 'NONE',  ( -23.46296185032722548, -19.82388608118403539, 1.000000000000000000 ) ) ;
#5637=EDGE_CURVE ( 'NONE', #3578, #13216, #3233, .T. ) ;
#5641=DIRECTION ( 'NONE',  ( 1.000000000000000000, 0.000000000000000000, 0.000000000000000000 ) ) ;
#5643=DIRECTION ( 'NONE',  ( 1.000000000000000000, 0.000000000000000000, 0.000000000000000000 ) ) ;
#5644=ORIENTED_EDGE ( 'NONE', *, *, #17773, .T. ) ;
#5645=FACE_OUTER_BOUND ( 'NONE', #22995, .T. ) ;
#5646=EDGE_LOOP ( 'NONE', ( #5869, #131, #23428, #24013 ) ) ;
#5648=DIRECTION ( 'NONE',  ( 0.000000000000000000, 0.000000000000000000, 1.000000000000000000 ) ) ;
#5651=VERTEX_POINT ( 'NONE', #21423 ) ;
#5655=DIRECTION ( 'NONE',  ( 0.9822872507286884991, -0.1873813145857256834, 0.000000000000000000 ) ) ;
#5657=VECTOR ( 'NONE', #24572, 1000.000000000000000 ) ;
#5664=EDGE_CURVE ( 'NONE', #14041, #13717, #169, .T. ) ;
#5667=CARTESIAN_POINT ( 'NONE',  ( -22.67092431280563503, 21.28941499438250062, -6.500000000000000000 ) ) ;
#5676=ORIENTED_EDGE ( 'NONE', *, *, #8645, .T. ) ;
#5680=CARTESIAN_POINT ( 'NONE',  ( 26.52310962334739486, -16.23990935651726275, -6.500000000000000000 ) ) ;
#5682=DIRECTION ( 'NONE',  ( 0.000000000000000000, 0.000000000000000000, 1.000000000000000000 ) ) ;
#5684=EDGE_CURVE ( 'NONE', #23080, #13703, #5170, .T. ) ;
#5685=DIRECTION ( 'NONE',  ( 0.000000000000000000, 0.000000000000000000, 1.000000000000000000 ) ) ;
#5686=DIRECTION ( 'NONE',  ( 0.000000000000000000, 0.000000000000000000, 1.000000000000000000 ) ) ;
#5693=CARTESIAN_POINT ( 'NONE',  ( -28.14012133169306296, 13.24173596767408867, -6.500000000000000000 ) ) ;
#5697=DIRECTION ( 'NONE',  ( 0.000000000000000000, 0.000000000000000000, 1.000000000000000000 ) ) ;
#5707=ORIENTED_EDGE ( 'NONE', *, *, #6994, .F. ) ;
#5708=ORIENTED_EDGE ( 'NONE', *, *, #14297, .T. ) ;
#5715=ADVANCED_FACE ( 'NONE', ( #10781 ), #2818, .F. ) ;
#5718=DIRECTION ( 'NONE',  ( -0.7705132427757840352, 0.6374239897486960738, 0.000000000000000000 ) ) ;
#5719=CARTESIAN_POINT ( 'NONE',  ( -11.44867358849309547, 28.91604871112477326, 1.000000000000000000 ) ) ;
#5723=DIRECTION ( 'NONE',  ( -0.9510565162951518658, 0.3090169943749528914, 0.000000000000000000 ) ) ;
#5736=ORIENTED_EDGE ( 'NONE', *, *, #10271, .F. ) ;
#5737=VERTEX_POINT ( 'NONE', #10393 ) ;
#5738=ORIENTED_EDGE ( 'NONE', *, *, #1001, .F. ) ;
#5740=CARTESIAN_POINT ( 'NONE',  ( 13.24173596767359662, -28.14012133169329388, 1.000000000000000000 ) ) ;
#5743=DIRECTION ( 'NONE',  ( 0.000000000000000000, 0.000000000000000000, 1.000000000000000000 ) ) ;
#5747=LINE ( 'NONE', #21464, #20471 ) ;
#5748=CARTESIAN_POINT ( 'NONE',  ( -25.16042852506064165, 18.28012134629622309, -6.500000000000000000 ) ) ;
#5750=CYLINDRICAL_SURFACE ( 'NONE', #20461, 0.5000000000000004441 ) ;
#5752=DIRECTION ( 'NONE',  ( -0.000000000000000000, -0.000000000000000000, 1.000000000000000000 ) ) ;
#5755=FACE_OUTER_BOUND ( 'NONE', #24409, .T. ) ;
#5756=ADVANCED_FACE ( 'NONE', ( #18392 ), #490, .F. ) ;
#5761=VERTEX_POINT ( 'NONE', #14862 ) ;
#5762=EDGE_CURVE ( 'NONE', #20598, #16676, #3477, .T. ) ;
#5763=ORIENTED_EDGE ( 'NONE', *, *, #20254, .F. ) ;
#5765=CIRCLE ( 'NONE', #2424, 31.10000000000000142 ) ;
#5766=ORIENTED_EDGE ( 'NONE', *, *, #13029, .F. ) ;
#5769=EDGE_LOOP ( 'NONE', ( #19394, #18871, #8880, #4766 ) ) ;
#5771=ORIENTED_EDGE ( 'NONE', *, *, #17070, .T. ) ;
#5772=EDGE_CURVE ( 'NONE', #4968, #5905, #2257, .T. ) ;
#5775=CARTESIAN_POINT ( 'NONE',  ( -29.57785765677917311, 9.610428525061202265, -6.500000000000000000 ) ) ;
#5776=CYLINDRICAL_SURFACE ( 'NONE', #9165, 0.5000000000000004441 ) ;
#5779=CIRCLE ( 'NONE', #7034, 31.10000000000000142 ) ;
#5780=DIRECTION ( 'NONE',  ( 1.000000000000000000, 0.000000000000000000, 0.000000000000000000 ) ) ;
#5786=CARTESIAN_POINT ( 'NONE',  ( -3.397863563850083146, -30.85476721088024021, -6.500000000000000000 ) ) ;
#5790=EDGE_CURVE ( 'NONE', #13306, #6385, #3504, .T. ) ;
#5791=CIRCLE ( 'NONE', #2457, 0.5000000000000006661 ) ;
#5792=ORIENTED_EDGE ( 'NONE', *, *, #21913, .T. ) ;
#5793=DIRECTION ( 'NONE',  ( 1.000000000000000000, 0.000000000000000000, 0.000000000000000000 ) ) ;
#5794=CIRCLE ( 'NONE', #19566, 31.10000000000000142 ) ;
#5796=DIRECTION ( 'NONE',  ( 0.000000000000000000, 0.000000000000000000, 1.000000000000000000 ) ) ;
#5799=VERTEX_POINT ( 'NONE', #21010 ) ;
#5800=CIRCLE ( 'NONE', #20835, 0.5000000000000001110 ) ;
#5802=VECTOR ( 'NONE', #13084, 1000.000000000000000 ) ;
#5804=EDGE_CURVE ( 'NONE', #4455, #1627, #6847, .T. ) ;
#5809=DIRECTION ( 'NONE',  ( 0.000000000000000000, 0.000000000000000000, 1.000000000000000000 ) ) ;
#5811=AXIS2_PLACEMENT_3D ( 'NONE', #2077, #25358, #7440 ) ;
#5814=AXIS2_PLACEMENT_3D ( 'NONE', #25283, #5397, #9579 ) ;
#5825=DIRECTION ( 'NONE',  ( 0.000000000000000000, -0.000000000000000000, -1.000000000000000000 ) ) ;
#5826=VERTEX_POINT ( 'NONE', #7139 ) ;
#5830=ORIENTED_EDGE ( 'NONE', *, *, #3597, .F. ) ;
#5834=AXIS2_PLACEMENT_3D ( 'NONE', #25451, #9385, #1795 ) ;
#5837=VERTEX_POINT ( 'NONE', #24922 ) ;
#5838=ORIENTED_EDGE ( 'NONE', *, *, #19516, .T. ) ;
#5842=EDGE_CURVE ( 'NONE', #10320, #7996, #19289, .T. ) ;
#5849=VECTOR ( 'NONE', #17437, 1000.000000000000000 ) ;
#5850=CARTESIAN_POINT ( 'NONE',  ( -1.452785157361865531, -31.03863125411923463, 1.000000000000000000 ) ) ;
#5856=ORIENTED_EDGE ( 'NONE', *, *, #12211, .F. ) ;
#5857=CYLINDRICAL_SURFACE ( 'NONE', #9697, 0.5000000000000004441 ) ;
#5860=VECTOR ( 'NONE', #3539, 1000.000000000000000 ) ;
#5862=DIRECTION ( 'NONE',  ( 1.000000000000000000, 0.000000000000000000, 0.000000000000000000 ) ) ;
#5863=DIRECTION ( 'NONE',  ( 0.000000000000000000, 0.000000000000000000, 1.000000000000000000 ) ) ;
#5864=ORIENTED_EDGE ( 'NONE', *, *, #14835, .F. ) ;
#5869=ORIENTED_EDGE ( 'NONE', *, *, #22549, .T. ) ;
#5873=ORIENTED_EDGE ( 'NONE', *, *, #7331, .T. ) ;
#5874=FACE_OUTER_BOUND ( 'NONE', #3360, .T. ) ;
#5876=EDGE_CURVE ( 'NONE', #4812, #9189, #24799, .T. ) ;
#5877=CIRCLE ( 'NONE', #21745, 31.10000000000000142 ) ;
#5879=AXIS2_PLACEMENT_3D ( 'NONE', #15777, #4653, #12635 ) ;
#5881=VECTOR ( 'NONE', #13871, 1000.000000000000000 ) ;
#5886=EDGE_CURVE ( 'NONE', #7162, #12485, #1002, .T. ) ;
#5887=DIRECTION ( 'NONE',  ( 0.3090169943749591086, 0.9510565162951497564, 0.000000000000000000 ) ) ;
#5895=DIRECTION ( 'NONE',  ( -0.000000000000000000, -0.000000000000000000, 1.000000000000000000 ) ) ;
#5901=ORIENTED_EDGE ( 'NONE', *, *, #7980, .T. ) ;
#5902=VECTOR ( 'NONE', #22321, 1000.000000000000000 ) ;
#5903=ORIENTED_EDGE ( 'NONE', *, *, #2796, .T. ) ;
#5904=DIRECTION ( 'NONE',  ( 0.000000000000000000, 0.000000000000000000, 1.000000000000000000 ) ) ;
#5905=VERTEX_POINT ( 'NONE', #1510 ) ;
#5915=EDGE_CURVE ( 'NONE', #7097, #23080, #14984, .T. ) ;
#5919=AXIS2_PLACEMENT_3D ( 'NONE', #15642, #11703, #19682 ) ;
#5924=EDGE_CURVE ( 'NONE', #15245, #15811, #23550, .T. ) ;
#5925=DIRECTION ( 'NONE',  ( 1.000000000000000000, 0.000000000000000000, 0.000000000000000000 ) ) ;
#5927=DIRECTION ( 'NONE',  ( 0.000000000000000000, 0.000000000000000000, 1.000000000000000000 ) ) ;
#5928=ORIENTED_EDGE ( 'NONE', *, *, #19790, .T. ) ;
#5929=VERTEX_POINT ( 'NONE', #3203 ) ;
#5931=AXIS2_PLACEMENT_3D ( 'NONE', #23799, #24184, #25761 ) ;
#5932=AXIS2_PLACEMENT_3D ( 'NONE', #7846, #13498, #25646 ) ;
#5939=ORIENTED_EDGE ( 'NONE', *, *, #24006, .F. ) ;
#5940=CIRCLE ( 'NONE', #6784, 31.10000000000000142 ) ;
#5947=DIRECTION ( 'NONE',  ( 1.000000000000000000, 0.000000000000000000, 0.000000000000000000 ) ) ;
#5948=FACE_OUTER_BOUND ( 'NONE', #1696, .T. ) ;
#5955=FACE_OUTER_BOUND ( 'NONE', #16589, .T. ) ;
#5960=CARTESIAN_POINT ( 'NONE',  ( 29.99470236596026496, -8.217531866531315288, -6.500000000000000000 ) ) ;
#5962=MECHANICAL_DESIGN_GEOMETRIC_PRESENTATION_REPRESENTATION('',(#18080),#3870);
#5963=CARTESIAN_POINT ( 'NONE',  ( -24.27856662945521649, -19.43607991388963185, -2.750000000000000000 ) ) ;
#5968=ORIENTED_EDGE ( 'NONE', *, *, #21128, .T. ) ;
#5970=DIRECTION ( 'NONE',  ( -0.9822872507286897203, -0.1873813145857189666, 0.000000000000000000 ) ) ;
#5973=ORIENTED_EDGE ( 'NONE', *, *, #23660, .T. ) ;
#5974=VERTEX_POINT ( 'NONE', #15509 ) ;
#5977=CIRCLE ( 'NONE', #5550, 31.10000000000000142 ) ;
#5980=AXIS2_PLACEMENT_3D ( 'NONE', #14052, #66, #16022 ) ;
#5989=VERTEX_POINT ( 'NONE', #19802 ) ;
#5990=CARTESIAN_POINT ( 'NONE',  ( 4.393401135980900207, -30.78811501957146390, -6.500000000000000000 ) ) ;
#5993=EDGE_CURVE ( 'NONE', #789, #15159, #16355, .T. ) ;
#5998=ORIENTED_EDGE ( 'NONE', *, *, #431, .F. ) ;
#6001=CARTESIAN_POINT ( 'NONE',  ( -14.48253926456298579, 27.25313774936435962, -6.500000000000000000 ) ) ;
#6002=DIRECTION ( 'NONE',  ( 0.000000000000000000, 0.000000000000000000, 1.000000000000000000 ) ) ;
#6004=AXIS2_PLACEMENT_3D ( 'NONE', #24558, #10962, #18815 ) ;
#6007=ORIENTED_EDGE ( 'NONE', *, *, #6490, .T. ) ;
#6018=DIRECTION ( 'NONE',  ( 1.000000000000000000, 0.000000000000000000, 0.000000000000000000 ) ) ;
#6019=EDGE_CURVE ( 'NONE', #10563, #12702, #12156, .T. ) ;
#6021=FACE_OUTER_BOUND ( 'NONE', #23857, .T. ) ;
#6022=DIRECTION ( 'NONE',  ( 0.000000000000000000, 0.000000000000000000, 1.000000000000000000 ) ) ;
#6023=CARTESIAN_POINT ( 'NONE',  ( 0.000000000000000000, 0.000000000000000000, -6.500000000000000000 ) ) ;
#6027=DIRECTION ( 'NONE',  ( 0.000000000000000000, 0.000000000000000000, 1.000000000000000000 ) ) ;
#6029=VERTEX_POINT ( 'NONE', #23990 ) ;
#6039=CYLINDRICAL_SURFACE ( 'NONE', #6354, 0.5000000000000004441 ) ;
#6040=AXIS2_PLACEMENT_3D ( 'NONE', #23259, #17386, #17130 ) ;
#6042=ORIENTED_EDGE ( 'NONE', *, *, #12864, .T. ) ;
#6052=EDGE_CURVE ( 'NONE', #18040, #7266, #24692, .T. ) ;
#6055=LINE ( 'NONE', #5786, #11165 ) ;
#6056=ORIENTED_EDGE ( 'NONE', *, *, #579, .T. ) ;
#6061=FACE_OUTER_BOUND ( 'NONE', #3393, .T. ) ;
#6065=ORIENTED_EDGE ( 'NONE', *, *, #12246, .T. ) ;
#6073=DIRECTION ( 'NONE',  ( 1.000000000000000000, 0.000000000000000000, 0.000000000000000000 ) ) ;
#6076=DIRECTION ( 'NONE',  ( 1.000000000000000000, 0.000000000000000000, 0.000000000000000000 ) ) ;
#6078=CARTESIAN_POINT ( 'NONE',  ( -31.06601413805600842, 1.453535542772947942, -2.750000000000000000 ) ) ;
#6082=CARTESIAN_POINT ( 'NONE',  ( -21.28941499438242246, -22.67092431280570963, -6.500000000000000000 ) ) ;
#6089=ORIENTED_EDGE ( 'NONE', *, *, #17341, .F. ) ;
#6092=ADVANCED_FACE ( 'NONE', ( #25817 ), #17981, .T. ) ;
#6094=DIRECTION ( 'NONE',  ( -0.000000000000000000, -0.000000000000000000, 1.000000000000000000 ) ) ;
#6095=EDGE_LOOP ( 'NONE', ( #11373, #18842, #4902, #21374 ) ) ;
#6105=CYLINDRICAL_SURFACE ( 'NONE', #24679, 31.10000000000000142 ) ;
#6110=EDGE_CURVE ( 'NONE', #4583, #3323, #6318, .T. ) ;
#6114=DIRECTION ( 'NONE',  ( 0.000000000000000000, 0.000000000000000000, 1.000000000000000000 ) ) ;
#6116=CARTESIAN_POINT ( 'NONE',  ( 0.000000000000000000, 0.000000000000000000, 1.000000000000000000 ) ) ;
#6122=CARTESIAN_POINT ( 'NONE',  ( 8.217531866531087914, 29.99470236596032535, 1.000000000000000000 ) ) ;
#6125=ORIENTED_EDGE ( 'NONE', *, *, #2638, .F. ) ;
#6126=VERTEX_POINT ( 'NONE', #4101 ) ;
#6127=EDGE_LOOP ( 'NONE', ( #16407, #643, #10816, #7298 ) ) ;
#6128=ADVANCED_FACE ( 'NONE', ( #21771 ), #11832, .F. ) ;
#6129=CARTESIAN_POINT ( 'NONE',  ( 21.28941499438209206, -22.67092431280601872, 1.000000000000000000 ) ) ;
#6132=EDGE_CURVE ( 'NONE', #9673, #7360, #2144, .T. ) ;
#6140=DIRECTION ( 'NONE',  ( 0.000000000000000000, -0.000000000000000000, 1.000000000000000000 ) ) ;
#6142=CARTESIAN_POINT ( 'NONE',  ( 29.72853858738281829, 9.133673601486481886, 1.000000000000000000 ) ) ;
#6150=VERTEX_POINT ( 'NONE', #24246 ) ;
#6152=CARTESIAN_POINT ( 'NONE',  ( 0.000000000000000000, 0.000000000000000000, -6.500000000000000000 ) ) ;
#6153=ORIENTED_EDGE ( 'NONE', *, *, #17946, .F. ) ;
#6156=VERTEX_POINT ( 'NONE', #22409 ) ;
#6157=ORIENTED_EDGE ( 'NONE', *, *, #17323, .T. ) ;
#6177=ORIENTED_EDGE ( 'NONE', *, *, #3638, .F. ) ;
#6178=ORIENTED_EDGE ( 'NONE', *, *, #22992, .T. ) ;
#6180=ORIENTED_EDGE ( 'NONE', *, *, #21709, .T. ) ;
#6181=CARTESIAN_POINT ( 'NONE',  ( -22.32573188046936252, -21.65113613650319380, -2.750000000000000000 ) ) ;
#6185=VERTEX_POINT ( 'NONE', #10241 ) ;
#6186=CIRCLE ( 'NONE', #9534, 0.5000000000000004441 ) ;
#6187=DIRECTION ( 'NONE',  ( 1.000000000000000000, 0.000000000000000000, 0.000000000000000000 ) ) ;
#6190=EDGE_CURVE ( 'NONE', #4202, #2078, #2791, .T. ) ;
#6192=EDGE_CURVE ( 'NONE', #485, #672, #23845, .T. ) ;
#6193=AXIS2_PLACEMENT_3D ( 'NONE', #13229, #3278, #19232 ) ;
#6200=AXIS2_PLACEMENT_3D ( 'NONE', #15039, #20925, #18963 ) ;
#6201=AXIS2_PLACEMENT_3D ( 'NONE', #15550, #11739, #7693 ) ;
#6203=DIRECTION ( 'NONE',  ( 0.000000000000000000, 0.000000000000000000, 1.000000000000000000 ) ) ;
#6206=AXIS2_PLACEMENT_3D ( 'NONE', #3324, #21002, #9084 ) ;
#6209=AXIS2_PLACEMENT_3D ( 'NONE', #18, #21857, #16223 ) ;
#6210=VERTEX_POINT ( 'NONE', #12345 ) ;
#6214=EDGE_LOOP ( 'NONE', ( #8723, #15432, #22137, #10428 ) ) ;
#6219=ORIENTED_EDGE ( 'NONE', *, *, #390, .T. ) ;
#6223=VECTOR ( 'NONE', #16290, 1000.000000000000000 ) ;
#6226=VECTOR ( 'NONE', #4840, 1000.000000000000000 ) ;
#6227=EDGE_CURVE ( 'NONE', #3169, #19826, #23036, .T. ) ;
#6232=DIRECTION ( 'NONE',  ( -0.000000000000000000, 0.000000000000000000, 1.000000000000000000 ) ) ;
#6237=CARTESIAN_POINT ( 'NONE',  ( -16.66421332384701515, -26.25859848311253941, -6.500000000000000000 ) ) ;
#6241=DIRECTION ( 'NONE',  ( 0.000000000000000000, 0.000000000000000000, 1.000000000000000000 ) ) ;
#6242=CYLINDRICAL_SURFACE ( 'NONE', #9237, 0.5000000000000004441 ) ;
#6247=AXIS2_PLACEMENT_3D ( 'NONE', #13210, #23025, #11369 ) ;
#6250=ORIENTED_EDGE ( 'NONE', *, *, #20484, .T. ) ;
#6254=DIRECTION ( 'NONE',  ( 1.000000000000000000, 0.000000000000000000, 0.000000000000000000 ) ) ;
#6256=AXIS2_PLACEMENT_3D ( 'NONE', #22513, #6682, #14672 ) ;
#6257=CIRCLE ( 'NONE', #23782, 31.10000000000000142 ) ;
#6258=ORIENTED_EDGE ( 'NONE', *, *, #10353, .T. ) ;
#6259=ORIENTED_EDGE ( 'NONE', *, *, #5664, .T. ) ;
#6260=VERTEX_POINT ( 'NONE', #14566 ) ;
#6261=LINE ( 'NONE', #7713, #14730 ) ;
#6263=AXIS2_PLACEMENT_3D ( 'NONE', #15686, #24041, #11754 ) ;
#6272=DIRECTION ( 'NONE',  ( 0.000000000000000000, 0.000000000000000000, 1.000000000000000000 ) ) ;
#6275=LINE ( 'NONE', #14266, #15480 ) ;
#6277=CARTESIAN_POINT ( 'NONE',  ( 20.92219106202043122, -23.01025686871645348, 1.000000000000000000 ) ) ;
#6282=AXIS2_PLACEMENT_3D ( 'NONE', #60, #24236, #6322 ) ;
#6283=CARTESIAN_POINT ( 'NONE',  ( -20.92219106202016476, 23.01025686871669507, -2.750000000000000000 ) ) ;
#6285=EDGE_LOOP ( 'NONE', ( #13987, #9602, #2460, #15231 ) ) ;
#6288=CYLINDRICAL_SURFACE ( 'NONE', #7482, 0.5000000000000004441 ) ;
#6289=ORIENTED_EDGE ( 'NONE', *, *, #22830, .T. ) ;
#6290=CIRCLE ( 'NONE', #21743, 0.5000000000000006661 ) ;
#6291=VECTOR ( 'NONE', #6769, 1000.000000000000000 ) ;
#6293=ORIENTED_EDGE ( 'NONE', *, *, #20736, .T. ) ;
#6294=VERTEX_POINT ( 'NONE', #2286 ) ;
#6296=CARTESIAN_POINT ( 'NONE',  ( 0.000000000000000000, 0.000000000000000000, -6.500000000000000000 ) ) ;
#6298=ORIENTED_EDGE ( 'NONE', *, *, #21496, .F. ) ;
#6304=AXIS2_PLACEMENT_3D ( 'NONE', #17385, #15418, #23647 ) ;
#6306=VECTOR ( 'NONE', #4744, 1000.000000000000000 ) ;
#6310=AXIS2_PLACEMENT_3D ( 'NONE', #3208, #7394, #3598 ) ;
#6314=EDGE_CURVE ( 'NONE', #3260, #19788, #55, .T. ) ;
#6317=EDGE_CURVE ( 'NONE', #9218, #20930, #6723, .T. ) ;
#6318=CIRCLE ( 'NONE', #11313, 0.5000000000000003331 ) ;
#6321=EDGE_LOOP ( 'NONE', ( #21146, #4388, #14760, #11756 ) ) ;
#6322=DIRECTION ( 'NONE',  ( -0.9510565162951518658, 0.3090169943749528914, 0.000000000000000000 ) ) ;
#6326=AXIS2_PLACEMENT_3D ( 'NONE', #9654, #15410, #9274 ) ;
#6331=DIRECTION ( 'NONE',  ( 0.000000000000000000, -0.000000000000000000, 1.000000000000000000 ) ) ;
#6333=DIRECTION ( 'NONE',  ( 0.000000000000000000, 0.000000000000000000, 1.000000000000000000 ) ) ;
#6334=CARTESIAN_POINT ( 'NONE',  ( -24.27856662945480792, 19.43607991389014344, -6.500000000000000000 ) ) ;
#6336=AXIS2_PLACEMENT_3D ( 'NONE', #7926, #19941, #451 ) ;
#6347=ORIENTED_EDGE ( 'NONE', *, *, #6574, .F. ) ;
#6354=AXIS2_PLACEMENT_3D ( 'NONE', #3817, #15849, #20275 ) ;
#6356=CYLINDRICAL_SURFACE ( 'NONE', #23835, 31.10000000000000142 ) ;
#6361=AXIS2_PLACEMENT_3D ( 'NONE', #3627, #25470, #19330 ) ;
#6363=CARTESIAN_POINT ( 'NONE',  ( -30.12293631110035363, 7.734255490827311341, 1.000000000000000000 ) ) ;
#6364=AXIS2_PLACEMENT_3D ( 'NONE', #15034, #23014, #3131 ) ;
#6365=ADVANCED_FACE ( 'NONE', ( #6976 ), #22932, .F. ) ;
#6366=CARTESIAN_POINT ( 'NONE',  ( 29.57785765677931167, 9.610428525060783045, 1.000000000000000000 ) ) ;
#6369=DIRECTION ( 'NONE',  ( 0.000000000000000000, 0.000000000000000000, -1.000000000000000000 ) ) ;
#6371=VECTOR ( 'NONE', #23750, 1000.000000000000000 ) ;
#6384=CARTESIAN_POINT ( 'NONE',  ( 20.20656826142266738, -23.64116323484245541, 1.000000000000000000 ) ) ;
#6385=VERTEX_POINT ( 'NONE', #13385 ) ;
#6389=DIRECTION ( 'NONE',  ( 1.000000000000000000, 0.000000000000000000, 0.000000000000000000 ) ) ;
#6391=ADVANCED_FACE ( 'NONE', ( #13250 ), #3303, .F. ) ;
#6392=AXIS2_PLACEMENT_3D ( 'NONE', #10885, #11027, #6711 ) ;
#6393=VERTEX_POINT ( 'NONE', #11028 ) ;
#6395=EDGE_LOOP ( 'NONE', ( #21419, #17397, #20143, #22060 ) ) ;
#6407=DIRECTION ( 'NONE',  ( 1.000000000000000000, 0.000000000000000000, 0.000000000000000000 ) ) ;
#6411=DIRECTION ( 'NONE',  ( 1.000000000000000000, 0.000000000000000000, 0.000000000000000000 ) ) ;
#6413=FACE_OUTER_BOUND ( 'NONE', #24072, .T. ) ;
#6415=ORIENTED_EDGE ( 'NONE', *, *, #22425, .T. ) ;
#6416=DIRECTION ( 'NONE',  ( 0.000000000000000000, -0.000000000000000000, 1.000000000000000000 ) ) ;
#6418=EDGE_LOOP ( 'NONE', ( #2715, #9504, #23976, #12853 ) ) ;
#6419=EDGE_CURVE ( 'NONE', #19701, #23209, #23310, .T. ) ;
#6420=ORIENTED_EDGE ( 'NONE', *, *, #4489, .F. ) ;
#6421=ORIENTED_EDGE ( 'NONE', *, *, #10921, .F. ) ;
#6422=ORIENTED_EDGE ( 'NONE', *, *, #12246, .F. ) ;
#6426=EDGE_CURVE ( 'NONE', #6185, #6210, #19676, .T. ) ;
#6429=ADVANCED_FACE ( 'NONE', ( #19008 ), #23188, .F. ) ;
#6435=EDGE_CURVE ( 'NONE', #20277, #8351, #25400, .T. ) ;
#6436=DIRECTION ( 'NONE',  ( 0.5358267949790093132, 0.8443279255020070817, 0.000000000000000000 ) ) ;
#6440=CARTESIAN_POINT ( 'NONE',  ( -3.897863563849436552, 30.85476721088031482, -6.500000000000000000 ) ) ;
#6446=ORIENTED_EDGE ( 'NONE', *, *, #15233, .F. ) ;
#6447=ORIENTED_EDGE ( 'NONE', *, *, #16714, .F. ) ;
#6451=ORIENTED_EDGE ( 'NONE', *, *, #20547, .F. ) ;
#6453=ORIENTED_EDGE ( 'NONE', *, *, #14801, .F. ) ;
#6457=VERTEX_POINT ( 'NONE', #7242 ) ;
#6459=ADVANCED_FACE ( 'NONE', ( #2927 ), #15094, .F. ) ;
#6461=DIRECTION ( 'NONE',  ( 0.000000000000000000, 0.000000000000000000, 1.000000000000000000 ) ) ;
#6463=DIRECTION ( 'NONE',  ( 0.000000000000000000, 0.000000000000000000, 1.000000000000000000 ) ) ;
#6466=ADVANCED_FACE ( 'NONE', ( #23578 ), #7748, .F. ) ;
#6469=VECTOR ( 'NONE', #15361, 1000.000000000000000 ) ;
#6473=CYLINDRICAL_SURFACE ( 'NONE', #17536, 31.10000000000000142 ) ;
#6483=ORIENTED_EDGE ( 'NONE', *, *, #18211, .F. ) ;
#6488=ADVANCED_FACE ( 'NONE', ( #4071 ), #13761, .F. ) ;
#6490=EDGE_CURVE ( 'NONE', #22605, #23233, #15922, .T. ) ;
#6495=DIRECTION ( 'NONE',  ( 0.000000000000000000, 0.000000000000000000, 1.000000000000000000 ) ) ;
#6499=DIRECTION ( 'NONE',  ( 1.000000000000000000, 0.000000000000000000, 0.000000000000000000 ) ) ;
#6501=DIRECTION ( 'NONE',  ( 1.000000000000000000, 0.000000000000000000, 0.000000000000000000 ) ) ;
#6502=ORIENTED_EDGE ( 'NONE', *, *, #11231, .T. ) ;
#6508=CARTESIAN_POINT ( 'NONE',  ( 0.000000000000000000, 0.000000000000000000, -6.500000000000000000 ) ) ;
#6517=DIRECTION ( 'NONE',  ( 1.000000000000000000, 0.000000000000000000, 0.000000000000000000 ) ) ;
#6520=EDGE_CURVE ( 'NONE', #20598, #3781, #22207, .T. ) ;
#6523=DIRECTION ( 'NONE',  ( 0.000000000000000000, 0.000000000000000000, 1.000000000000000000 ) ) ;
#6525=EDGE_CURVE ( 'NONE', #5290, #23357, #10922, .T. ) ;
#6530=DIRECTION ( 'NONE',  ( -0.3681245526846659843, 0.9297764858882561212, 0.000000000000000000 ) ) ;
#6534=DIRECTION ( 'NONE',  ( -0.3681245526846659843, 0.9297764858882561212, 0.000000000000000000 ) ) ;
#6536=LINE ( 'NONE', #6927, #25437 ) ;
#6538=ORIENTED_EDGE ( 'NONE', *, *, #4434, .T. ) ;
#6539=CARTESIAN_POINT ( 'NONE',  ( -14.98253926456298579, 27.25313774936435962, -6.500000000000000000 ) ) ;
#6541=ORIENTED_EDGE ( 'NONE', *, *, #20248, .F. ) ;
#6542=VERTEX_POINT ( 'NONE', #13638 ) ;
#6545=ORIENTED_EDGE ( 'NONE', *, *, #5241, .F. ) ;
#6547=DIRECTION ( 'NONE',  ( 1.000000000000000000, 0.000000000000000000, 0.000000000000000000 ) ) ;
#6549=CARTESIAN_POINT ( 'NONE',  ( -27.10000000000000142, 0.000000000000000000, 0.000000000000000000 ) ) ;
#6550=CARTESIAN_POINT ( 'NONE',  ( 0.000000000000000000, 0.000000000000000000, -6.500000000000000000 ) ) ;
#6565=EDGE_CURVE ( 'NONE', #19625, #18150, #11767, .T. ) ;
#6568=ORIENTED_EDGE ( 'NONE', *, *, #14610, .T. ) ;
#6572=VERTEX_POINT ( 'NONE', #868 ) ;
#6573=DIRECTION ( 'NONE',  ( 0.000000000000000000, 0.000000000000000000, 1.000000000000000000 ) ) ;
#6574=EDGE_CURVE ( 'NONE', #10324, #19323, #18037, .T. ) ;
#6575=ORIENTED_EDGE ( 'NONE', *, *, #11151, .T. ) ;
#6577=DIRECTION ( 'NONE',  ( 0.000000000000000000, 0.000000000000000000, 1.000000000000000000 ) ) ;
#6578=ORIENTED_EDGE ( 'NONE', *, *, #15011, .F. ) ;
#6581=CYLINDRICAL_SURFACE ( 'NONE', #23898, 31.10000000000000142 ) ;
#6590=EDGE_CURVE ( 'NONE', #21352, #25423, #1759, .T. ) ;
#6595=ORIENTED_EDGE ( 'NONE', *, *, #17953, .F. ) ;
#6598=EDGE_CURVE ( 'NONE', #14914, #5737, #6747, .T. ) ;
#6600=ORIENTED_EDGE ( 'NONE', *, *, #6052, .T. ) ;
#6601=ORIENTED_EDGE ( 'NONE', *, *, #12325, .T. ) ;
#6602=DIRECTION ( 'NONE',  ( 1.000000000000000000, 0.000000000000000000, 0.000000000000000000 ) ) ;
#6603=CIRCLE ( 'NONE', #2854, 0.4999999999999998890 ) ;
#6607=DIRECTION ( 'NONE',  ( 0.000000000000000000, -0.000000000000000000, 1.000000000000000000 ) ) ;
#6615=DIRECTION ( 'NONE',  ( 0.3681245526846875782, 0.9297764858882475725, 0.000000000000000000 ) ) ;
#6616=CARTESIAN_POINT ( 'NONE',  ( -3.897863563849436552, 30.85476721088031482, 1.000000000000000000 ) ) ;
#6617=VECTOR ( 'NONE', #19720, 1000.000000000000000 ) ;
#6618=CARTESIAN_POINT ( 'NONE',  ( -19.82388608118446527, -23.96296185032687376, 1.000000000000000000 ) ) ;
#6624=CARTESIAN_POINT ( 'NONE',  ( -30.91344420362549172, -3.401318489840897019, 1.000000000000000000 ) ) ;
#6626=DIRECTION ( 'NONE',  ( 0.000000000000000000, 0.000000000000000000, -1.000000000000000000 ) ) ;
#6628=ORIENTED_EDGE ( 'NONE', *, *, #14268, .T. ) ;
#6634=ORIENTED_EDGE ( 'NONE', *, *, #9319, .F. ) ;
#6637=VECTOR ( 'NONE', #2173, 1000.000000000000000 ) ;
#6640=ORIENTED_EDGE ( 'NONE', *, *, #12893, .F. ) ;
#6642=CARTESIAN_POINT ( 'NONE',  ( -5.827558883616271501, -30.54913349766217934, 1.000000000000000000 ) ) ;
#6646=ADVANCED_FACE ( 'NONE', ( #21798 ), #7797, .F. ) ;
#6647=CIRCLE ( 'NONE', #16269, 0.4999999999999993894 ) ;
#6655=DIRECTION ( 'NONE',  ( 0.000000000000000000, 0.000000000000000000, 1.000000000000000000 ) ) ;
#6658=CARTESIAN_POINT ( 'NONE',  ( -0.4999838450259764255, 31.09598070739550124, 1.000000000000000000 ) ) ;
#6661=CARTESIAN_POINT ( 'NONE',  ( -7.734255490827218971, -30.12293631110037140, -6.500000000000000000 ) ) ;
#6663=DIRECTION ( 'NONE',  ( 0.000000000000000000, -0.000000000000000000, 1.000000000000000000 ) ) ;
#6665=ORIENTED_EDGE ( 'NONE', *, *, #17800, .F. ) ;
#6666=DIRECTION ( 'NONE',  ( 0.000000000000000000, 0.000000000000000000, 1.000000000000000000 ) ) ;
#6670=EDGE_LOOP ( 'NONE', ( #9857, #20964, #21991, #10810 ) ) ;
#6671=VERTEX_POINT ( 'NONE', #17482 ) ;
#6672=VERTEX_POINT ( 'NONE', #10012 ) ;
#6673=VERTEX_POINT ( 'NONE', #7675 ) ;
#6675=AXIS2_PLACEMENT_3D ( 'NONE', #21199, #3277, #11250 ) ;
#6677=CARTESIAN_POINT ( 'NONE',  ( 23.64116323484238080, 20.20656826142275264, -2.750000000000000000 ) ) ;
#6680=EDGE_CURVE ( 'NONE', #4728, #4688, #19267, .T. ) ;
#6682=DIRECTION ( 'NONE',  ( 0.000000000000000000, 0.000000000000000000, 1.000000000000000000 ) ) ;
#6687=DIRECTION ( 'NONE',  ( 0.000000000000000000, 0.000000000000000000, 1.000000000000000000 ) ) ;
#6689=FACE_OUTER_BOUND ( 'NONE', #19441, .T. ) ;
#6690=DIRECTION ( 'NONE',  ( 0.000000000000000000, -0.000000000000000000, -1.000000000000000000 ) ) ;
#6693=AXIS2_PLACEMENT_3D ( 'NONE', #5197, #22853, #7288 ) ;
#6696=ORIENTED_EDGE ( 'NONE', *, *, #4698, .T. ) ;
#6699=AXIS2_PLACEMENT_3D ( 'NONE', #8537, #20684, #8928 ) ;
#6700=EDGE_LOOP ( 'NONE', ( #15869, #6600, #24648, #23026 ) ) ;
#6707=VERTEX_POINT ( 'NONE', #15776 ) ;
#6708=EDGE_CURVE ( 'NONE', #10320, #21754, #10085, .T. ) ;
#6711=DIRECTION ( 'NONE',  ( 1.000000000000000000, 0.000000000000000000, 0.000000000000000000 ) ) ;
#6712=AXIS2_PLACEMENT_3D ( 'NONE', #14512, #20258, #22233 ) ;
#6714=DIRECTION ( 'NONE',  ( 1.387778780781445044E-14, 1.000000000000000000, 0.000000000000000000 ) ) ;
#6715=CARTESIAN_POINT ( 'NONE',  ( 29.72853858738285737, 9.133673601486364646, -2.750000000000000000 ) ) ;
#6717=CIRCLE ( 'NONE', #2136, 0.4999999999999991118 ) ;
#6719=CIRCLE ( 'NONE', #5466, 0.4999999999999991118 ) ;
#6722=CARTESIAN_POINT ( 'NONE',  ( -23.01025686871616216, 20.92219106202074741, -2.750000000000000000 ) ) ;
#6723=CIRCLE ( 'NONE', #10898, 31.10000000000000142 ) ;
#6724=CARTESIAN_POINT ( 'NONE',  ( 0.000000000000000000, 0.000000000000000000, 1.000000000000000000 ) ) ;
#6729=AXIS2_PLACEMENT_3D ( 'NONE', #18439, #19574, #11094 ) ;
#6731=ORIENTED_EDGE ( 'NONE', *, *, #21422, .F. ) ;
#6733=EDGE_CURVE ( 'NONE', #23985, #7474, #20545, .T. ) ;
#6734=CARTESIAN_POINT ( 'NONE',  ( -30.35476721088022600, 3.897863563850190616, -6.500000000000000000 ) ) ;
#6736=ORIENTED_EDGE ( 'NONE', *, *, #5664, .F. ) ;
#6739=AXIS2_PLACEMENT_3D ( 'NONE', #9995, #17989, #4107 ) ;
#6740=EDGE_CURVE ( 'NONE', #13215, #364, #23865, .T. ) ;
#6744=CARTESIAN_POINT ( 'NONE',  ( 7.734255490827002255, 30.12293631110042469, -6.500000000000000000 ) ) ;
#6746=ADVANCED_FACE ( 'NONE', ( #9637, #23626 ), #15914, .T. ) ;
#6747=CIRCLE ( 'NONE', #14289, 0.4999999999999997224 ) ;
#6750=EDGE_CURVE ( 'NONE', #15121, #9972, #13030, .T. ) ;
#6751=AXIS2_PLACEMENT_3D ( 'NONE', #10640, #22300, #18634 ) ;
#6752=CIRCLE ( 'NONE', #5503, 0.5000000000000002220 ) ;
#6756=AXIS2_PLACEMENT_3D ( 'NONE', #12326, #24965, #17000 ) ;
#6757=DIRECTION ( 'NONE',  ( 0.8763066800438640280, -0.4817536741017146018, 0.000000000000000000 ) ) ;
#6759=DIRECTION ( 'NONE',  ( 1.000000000000000000, 0.000000000000000000, 0.000000000000000000 ) ) ;
#6762=DIRECTION ( 'NONE',  ( 0.000000000000000000, -0.000000000000000000, 1.000000000000000000 ) ) ;
#6765=DIRECTION ( 'NONE',  ( -0.000000000000000000, 0.000000000000000000, -1.000000000000000000 ) ) ;
#6766=VERTEX_POINT ( 'NONE', #19700 ) ;
#6767=CIRCLE ( 'NONE', #95, 0.5000000000000003331 ) ;
#6769=DIRECTION ( 'NONE',  ( 0.000000000000000000, 0.000000000000000000, -1.000000000000000000 ) ) ;
#6770=ORIENTED_EDGE ( 'NONE', *, *, #9923, .F. ) ;
#6778=CIRCLE ( 'NONE', #5932, 0.4999999999999998890 ) ;
#6781=ORIENTED_EDGE ( 'NONE', *, *, #12288, .T. ) ;
#6784=AXIS2_PLACEMENT_3D ( 'NONE', #22959, #733, #19153 ) ;
#6786=DIRECTION ( 'NONE',  ( 0.000000000000000000, 0.000000000000000000, 1.000000000000000000 ) ) ;
#6792=EDGE_CURVE ( 'NONE', #23568, #14371, #4658, .T. ) ;
#6793=VECTOR ( 'NONE', #14276, 1000.000000000000000 ) ;
#6800=CARTESIAN_POINT ( 'NONE',  ( -27.25313774936430633, -14.98253926456308172, 1.000000000000000000 ) ) ;
#6803=DIRECTION ( 'NONE',  ( 0.000000000000000000, 0.000000000000000000, 1.000000000000000000 ) ) ;
#6806=DIRECTION ( 'NONE',  ( 0.000000000000000000, 0.000000000000000000, 1.000000000000000000 ) ) ;
#6807=ORIENTED_EDGE ( 'NONE', *, *, #13641, .T. ) ;
#6808=FACE_OUTER_BOUND ( 'NONE', #24296, .T. ) ;
#6809=DIRECTION ( 'NONE',  ( 0.000000000000000000, 0.000000000000000000, 1.000000000000000000 ) ) ;
#6810=VERTEX_POINT ( 'NONE', #3741 ) ;
#6811=AXIS2_PLACEMENT_3D ( 'NONE', #25307, #7385, #17074 ) ;
#6813=ORIENTED_EDGE ( 'NONE', *, *, #9008, .F. ) ;
#6815=ORIENTED_EDGE ( 'NONE', *, *, #24365, .T. ) ;
#6821=CIRCLE ( 'NONE', #17674, 0.5000000000000005551 ) ;
#6833=FACE_OUTER_BOUND ( 'NONE', #13337, .T. ) ;
#6837=EDGE_LOOP ( 'NONE', ( #24164, #1700, #16785, #17966 ) ) ;
#6838=ORIENTED_EDGE ( 'NONE', *, *, #11478, .T. ) ;
#6843=ORIENTED_EDGE ( 'NONE', *, *, #21664, .T. ) ;
#6846=DIRECTION ( 'NONE',  ( 0.000000000000000000, 0.000000000000000000, 1.000000000000000000 ) ) ;
#6847=CIRCLE ( 'NONE', #5595, 0.4999999999999991118 ) ;
#6848=ORIENTED_EDGE ( 'NONE', *, *, #6110, .T. ) ;
#6852=CARTESIAN_POINT ( 'NONE',  ( -30.63887302793251521, -5.335677986744475021, -2.750000000000000000 ) ) ;
#6859=CARTESIAN_POINT ( 'NONE',  ( -19.82388608118395013, 23.96296185032730364, 1.000000000000000000 ) ) ;
#6861=ORIENTED_EDGE ( 'NONE', *, *, #15696, .T. ) ;
#6866=CARTESIAN_POINT ( 'NONE',  ( 8.217531866531214035, 29.99470236596028982, -2.750000000000000000 ) ) ;
#6868=DIRECTION ( 'NONE',  ( 0.000000000000000000, 0.000000000000000000, 1.000000000000000000 ) ) ;
#6870=ORIENTED_EDGE ( 'NONE', *, *, #2406, .T. ) ;
#6873=CARTESIAN_POINT ( 'NONE',  ( 3.897863563849651936, -30.85476721088028640, -6.500000000000000000 ) ) ;
#6876=DIRECTION ( 'NONE',  ( 0.000000000000000000, 0.000000000000000000, 1.000000000000000000 ) ) ;
#6880=DIRECTION ( 'NONE',  ( 0.2486898871648653975, 0.9685831611286285225, 0.000000000000000000 ) ) ;
#6886=CARTESIAN_POINT ( 'NONE',  ( 11.91206721063051432, 28.72825533807128551, -6.500000000000000000 ) ) ;
#6887=DIRECTION ( 'NONE',  ( 0.000000000000000000, 0.000000000000000000, 1.000000000000000000 ) ) ;
#6893=DIRECTION ( 'NONE',  ( 0.000000000000000000, 0.000000000000000000, 1.000000000000000000 ) ) ;
#6894=EDGE_CURVE ( 'NONE', #18387, #12818, #11335, .T. ) ;
#6900=CARTESIAN_POINT ( 'NONE',  ( -25.16042852506104666, -18.28012134629567598, 1.000000000000000000 ) ) ;
#6902=DIRECTION ( 'NONE',  ( 0.8443279255020154084, -0.5358267949789962126, 0.000000000000000000 ) ) ;
#6903=ORIENTED_EDGE ( 'NONE', *, *, #4530, .T. ) ;
#6907=ORIENTED_EDGE ( 'NONE', *, *, #17726, .F. ) ;
#6908=DIRECTION ( 'NONE',  ( 0.000000000000000000, 0.000000000000000000, 1.000000000000000000 ) ) ;
#6910=CARTESIAN_POINT ( 'NONE',  ( -14.98253926456356666, -27.25313774936403988, -6.500000000000000000 ) ) ;
#6913=EDGE_CURVE ( 'NONE', #16170, #12311, #7100, .T. ) ;
#6920=CARTESIAN_POINT ( 'NONE',  ( 19.82388608118411710, -23.96296185032715798, 1.000000000000000000 ) ) ;
#6927=CARTESIAN_POINT ( 'NONE',  ( 22.32573188046904633, -21.65113613650351709, -2.750000000000000000 ) ) ;
#6930=ORIENTED_EDGE ( 'NONE', *, *, #2909, .F. ) ;
#6931=AXIS2_PLACEMENT_3D ( 'NONE', #18042, #4418, #20497 ) ;
#6933=DIRECTION ( 'NONE',  ( -0.8763066800438656934, -0.4817536741017116597, 0.000000000000000000 ) ) ;
#6937=EDGE_LOOP ( 'NONE', ( #3883, #24733, #5771, #1346 ) ) ;
#6939=VERTEX_POINT ( 'NONE', #4879 ) ;
#6944=ADVANCED_FACE ( 'NONE', ( #18879 ), #2665, .F. ) ;
#6949=LINE ( 'NONE', #562, #23796 ) ;
#6957=CARTESIAN_POINT ( 'NONE',  ( -26.25859848311282363, -16.66421332384654974, -6.500000000000000000 ) ) ;
#6959=CYLINDRICAL_SURFACE ( 'NONE', #12874, 0.5000000000000004441 ) ;
#6961=ORIENTED_EDGE ( 'NONE', *, *, #1682, .T. ) ;
#6962=ORIENTED_EDGE ( 'NONE', *, *, #22803, .T. ) ;
#6963=ORIENTED_EDGE ( 'NONE', *, *, #19852, .F. ) ;
#6967=ADVANCED_FACE ( 'NONE', ( #23062 ), #18498, .F. ) ;
#6969=DIRECTION ( 'NONE',  ( 0.000000000000000000, -0.000000000000000000, 1.000000000000000000 ) ) ;
#6970=EDGE_CURVE ( 'NONE', #9505, #25113, #8434, .T. ) ;
#6971=ORIENTED_EDGE ( 'NONE', *, *, #25063, .T. ) ;
#6972=DIRECTION ( 'NONE',  ( 0.000000000000000000, 0.000000000000000000, 1.000000000000000000 ) ) ;
#6976=FACE_OUTER_BOUND ( 'NONE', #15743, .T. ) ;
#6979=DIRECTION ( 'NONE',  ( 1.000000000000000000, 0.000000000000000000, 0.000000000000000000 ) ) ;
#6990=EDGE_LOOP ( 'NONE', ( #13780, #1474, #5491, #16402 ) ) ;
#6991=ADVANCED_FACE ( 'NONE', ( #25394 ), #7236, .F. ) ;
#6992=ORIENTED_EDGE ( 'NONE', *, *, #21739, .F. ) ;
#6993=FACE_OUTER_BOUND ( 'NONE', #24232, .T. ) ;
#6994=EDGE_CURVE ( 'NONE', #1492, #24730, #25148, .T. ) ;
#6995=CARTESIAN_POINT ( 'NONE',  ( -9.133673601486059113, 29.72853858738294619, -2.750000000000000000 ) ) ;
#6998=CARTESIAN_POINT ( 'NONE',  ( -1.452785157361865531, -31.03863125411923463, -6.500000000000000000 ) ) ;
#7000=DIRECTION ( 'NONE',  ( 0.2486898871648519360, -0.9685831611286318532, 0.000000000000000000 ) ) ;
#7006=CYLINDRICAL_SURFACE ( 'NONE', #2157, 31.10000000000000142 ) ;
#7012=CARTESIAN_POINT ( 'NONE',  ( 0.000000000000000000, 0.000000000000000000, -6.500000000000000000 ) ) ;
#7019=CARTESIAN_POINT ( 'NONE',  ( -21.28941499438242246, -22.67092431280570963, -6.500000000000000000 ) ) ;
#7022=DIRECTION ( 'NONE',  ( -0.8763066800438602533, 0.4817536741017213187, 0.000000000000000000 ) ) ;
#7028=ORIENTED_EDGE ( 'NONE', *, *, #18367, .F. ) ;
#7031=AXIS2_PLACEMENT_3D ( 'NONE', #19342, #11491, #19463 ) ;
#7034=AXIS2_PLACEMENT_3D ( 'NONE', #18111, #24491, #18227 ) ;
#7035=VECTOR ( 'NONE', #7184, 1000.000000000000000 ) ;
#7037=EDGE_CURVE ( 'NONE', #21732, #5974, #2165, .T. ) ;
#7040=CARTESIAN_POINT ( 'NONE',  ( 0.000000000000000000, 0.000000000000000000, -6.500000000000000000 ) ) ;
#7041=CARTESIAN_POINT ( 'NONE',  ( -14.98253926456356666, -27.25313774936403988, -6.500000000000000000 ) ) ;
#7045=DIRECTION ( 'NONE',  ( 0.000000000000000000, 0.000000000000000000, 1.000000000000000000 ) ) ;
#7046=LINE ( 'NONE', #9400, #13722 ) ;
#7047=CARTESIAN_POINT ( 'NONE',  ( 0.000000000000000000, 0.000000000000000000, -6.500000000000000000 ) ) ;
#7048=CARTESIAN_POINT ( 'NONE',  ( 0.000000000000000000, 0.000000000000000000, 1.000000000000000000 ) ) ;
#7060=AXIS2_PLACEMENT_3D ( 'NONE', #16560, #12762, #4385 ) ;
#7067=ORIENTED_EDGE ( 'NONE', *, *, #8131, .T. ) ;
#7068=DIRECTION ( 'NONE',  ( 0.000000000000000000, 0.000000000000000000, 1.000000000000000000 ) ) ;
#7074=EDGE_CURVE ( 'NONE', #8556, #19701, #13454, .T. ) ;
#7076=AXIS2_PLACEMENT_3D ( 'NONE', #11923, #10091, #8143 ) ;
#7081=CARTESIAN_POINT ( 'NONE',  ( -1.952785157361865753, -31.03863125411923463, -6.500000000000000000 ) ) ;
#7082=ADVANCED_FACE ( 'NONE', ( #11533 ), #11410, .T. ) ;
#7087=DIRECTION ( 'NONE',  ( 0.000000000000000000, 0.000000000000000000, 1.000000000000000000 ) ) ;
#7090=VERTEX_POINT ( 'NONE', #13632 ) ;
#7091=ORIENTED_EDGE ( 'NONE', *, *, #1628, .T. ) ;
#7093=AXIS2_PLACEMENT_3D ( 'NONE', #12645, #16841, #10930 ) ;
#7094=CIRCLE ( 'NONE', #13775, 0.4999999999999991673 ) ;
#7097=VERTEX_POINT ( 'NONE', #3173 ) ;
#7099=ORIENTED_EDGE ( 'NONE', *, *, #5478, .T. ) ;
#7100=LINE ( 'NONE', #22802, #14694 ) ;
#7101=AXIS2_PLACEMENT_3D ( 'NONE', #8013, #18091, #17820 ) ;
#7102=CIRCLE ( 'NONE', #2504, 31.10000000000000142 ) ;
#7103=VERTEX_POINT ( 'NONE', #13245 ) ;
#7104=CARTESIAN_POINT ( 'NONE',  ( 0.000000000000000000, 0.000000000000000000, -6.500000000000000000 ) ) ;
#7108=CARTESIAN_POINT ( 'NONE',  ( -22.67092431280609688, -21.28941499438201745, -6.500000000000000000 ) ) ;
#7109=CARTESIAN_POINT ( 'NONE',  ( -27.10000000000000142, 0.000000000000000000, 1.000000000000000000 ) ) ;
#7111=CIRCLE ( 'NONE', #4171, 0.5000000000000003331 ) ;
#7114=EDGE_CURVE ( 'NONE', #18048, #1796, #11758, .T. ) ;
#7128=ORIENTED_EDGE ( 'NONE', *, *, #15842, .T. ) ;
#7130=FACE_OUTER_BOUND ( 'NONE', #17510, .T. ) ;
#7132=AXIS2_PLACEMENT_3D ( 'NONE', #25672, #4074, #12047 ) ;
#7134=VERTEX_POINT ( 'NONE', #7617 ) ;
#7138=CIRCLE ( 'NONE', #17174, 0.5000000000000005551 ) ;
#7139=CARTESIAN_POINT ( 'NONE',  ( -17.87326343783962201, -25.45105997952905597, 1.000000000000000000 ) ) ;
#7142=CYLINDRICAL_SURFACE ( 'NONE', #11285, 0.5000000000000004441 ) ;
#7143=DIRECTION ( 'NONE',  ( 0.3681245526846875782, 0.9297764858882475725, 0.000000000000000000 ) ) ;
#7147=CYLINDRICAL_SURFACE ( 'NONE', #5066, 31.10000000000000142 ) ;
#7154=DIRECTION ( 'NONE',  ( 0.000000000000000000, -0.000000000000000000, 1.000000000000000000 ) ) ;
#7161=CARTESIAN_POINT ( 'NONE',  ( 5.335677986744788548, 30.63887302793246548, 1.000000000000000000 ) ) ;
#7162=VERTEX_POINT ( 'NONE', #16773 ) ;
#7165=AXIS2_PLACEMENT_3D ( 'NONE', #7108, #23071, #5156 ) ;
#7166=ORIENTED_EDGE ( 'NONE', *, *, #362, .T. ) ;
#7174=AXIS2_PLACEMENT_3D ( 'NONE', #13799, #5685, #1781 ) ;
#7176=AXIS2_PLACEMENT_3D ( 'NONE', #1783, #18243, #4634 ) ;
#7181=DIRECTION ( 'NONE',  ( -0.000000000000000000, 0.000000000000000000, 1.000000000000000000 ) ) ;
#7184=DIRECTION ( 'NONE',  ( -0.000000000000000000, 0.000000000000000000, -1.000000000000000000 ) ) ;
#7188=VECTOR ( 'NONE', #8743, 1000.000000000000000 ) ;
#7192=DIRECTION ( 'NONE',  ( 0.000000000000000000, 0.000000000000000000, 1.000000000000000000 ) ) ;
#7193=DIRECTION ( 'NONE',  ( -0.9048270524660170233, 0.4257792915650782661, 0.000000000000000000 ) ) ;
#7194=DIRECTION ( 'NONE',  ( 0.000000000000000000, -0.000000000000000000, 1.000000000000000000 ) ) ;
#7195=ORIENTED_EDGE ( 'NONE', *, *, #10760, .T. ) ;
#7196=AXIS2_PLACEMENT_3D ( 'NONE', #1243, #17216, #23097 ) ;
#7197=CARTESIAN_POINT ( 'NONE',  ( 31.03863125411925239, 1.952785157361540236, -6.500000000000000000 ) ) ;
#7199=ORIENTED_EDGE ( 'NONE', *, *, #20821, .T. ) ;
#7200=AXIS2_PLACEMENT_3D ( 'NONE', #4408, #6241, #23768 ) ;
#7202=ORIENTED_EDGE ( 'NONE', *, *, #25667, .F. ) ;
#7204=VERTEX_POINT ( 'NONE', #19678 ) ;
#7207=VECTOR ( 'NONE', #12959, 1000.000000000000000 ) ;
#7208=DIRECTION ( 'NONE',  ( 1.000000000000000000, 0.000000000000000000, 0.000000000000000000 ) ) ;
#7209=CIRCLE ( 'NONE', #3448, 31.10000000000000142 ) ;
#7214=CYLINDRICAL_SURFACE ( 'NONE', #25483, 31.10000000000000142 ) ;
#7217=CYLINDRICAL_SURFACE ( 'NONE', #22980, 0.5000000000000004441 ) ;
#7219=DIRECTION ( 'NONE',  ( 1.000000000000000000, 0.000000000000000000, 0.000000000000000000 ) ) ;
#7220=DIRECTION ( 'NONE',  ( 0.000000000000000000, -0.000000000000000000, 1.000000000000000000 ) ) ;
#7222=CIRCLE ( 'NONE', #15164, 0.5000000000000011102 ) ;
#7225=ORIENTED_EDGE ( 'NONE', *, *, #24143, .F. ) ;
#7228=AXIS2_PLACEMENT_3D ( 'NONE', #17548, #19875, #1975 ) ;
#7232=ORIENTED_EDGE ( 'NONE', *, *, #6314, .T. ) ;
#7233=DIRECTION ( 'NONE',  ( 1.000000000000000000, 0.000000000000000000, 0.000000000000000000 ) ) ;
#7235=ORIENTED_EDGE ( 'NONE', *, *, #25271, .T. ) ;
#7236=CYLINDRICAL_SURFACE ( 'NONE', #79, 0.5000000000000002220 ) ;
#7237=ORIENTED_EDGE ( 'NONE', *, *, #3425, .T. ) ;
#7238=EDGE_CURVE ( 'NONE', #21069, #25296, #3009, .T. ) ;
#7241=CIRCLE ( 'NONE', #22716, 0.4999999999999992784 ) ;
#7242=CARTESIAN_POINT ( 'NONE',  ( 31.09598070739550479, -0.4999838450259578293, 1.000000000000000000 ) ) ;
#7246=CARTESIAN_POINT ( 'NONE',  ( -31.06601413805600842, 1.453535542772947942, 1.000000000000000000 ) ) ;
#7250=DIRECTION ( 'NONE',  ( 1.000000000000000000, 0.000000000000000000, 0.000000000000000000 ) ) ;
#7252=ORIENTED_EDGE ( 'NONE', *, *, #4704, .F. ) ;
#7254=AXIS2_PLACEMENT_3D ( 'NONE', #11102, #9019, #15420 ) ;
#7263=ORIENTED_EDGE ( 'NONE', *, *, #7770, .T. ) ;
#7264=DIRECTION ( 'NONE',  ( -0.000000000000000000, -0.000000000000000000, 1.000000000000000000 ) ) ;
#7265=DIRECTION ( 'NONE',  ( 1.000000000000000000, 0.000000000000000000, 0.000000000000000000 ) ) ;
#7266=VERTEX_POINT ( 'NONE', #24363 ) ;
#7267=EDGE_CURVE ( 'NONE', #6707, #7998, #22788, .T. ) ;
#7270=DIRECTION ( 'NONE',  ( -0.5877852522924775780, -0.8090169943749443426, 0.000000000000000000 ) ) ;
#7277=DIRECTION ( 'NONE',  ( 0.000000000000000000, -0.000000000000000000, -1.000000000000000000 ) ) ;
#7285=FACE_OUTER_BOUND ( 'NONE', #22422, .T. ) ;
#7288=DIRECTION ( 'NONE',  ( 0.9297764858882561212, 0.3681245526846659843, 0.000000000000000000 ) ) ;
#7293=DIRECTION ( 'NONE',  ( 0.000000000000000000, 0.000000000000000000, 1.000000000000000000 ) ) ;
#7294=ORIENTED_EDGE ( 'NONE', *, *, #54, .F. ) ;
#7298=ORIENTED_EDGE ( 'NONE', *, *, #6426, .F. ) ;
#7299=ORIENTED_EDGE ( 'NONE', *, *, #21623, .T. ) ;
#7303=AXIS2_PLACEMENT_3D ( 'NONE', #17339, #19526, #25305 ) ;
#7307=DIRECTION ( 'NONE',  ( -0.6374239897486919659, -0.7705132427757873659, 0.000000000000000000 ) ) ;
#7308=CARTESIAN_POINT ( 'NONE',  ( 30.24338421796784004, 7.248980000274092284, -2.750000000000000000 ) ) ;
#7311=LINE ( 'NONE', #25098, #20393 ) ;
#7321=CARTESIAN_POINT ( 'NONE',  ( 18.68225429291714690, -24.86329371854781201, 1.000000000000000000 ) ) ;
#7322=ORIENTED_EDGE ( 'NONE', *, *, #21921, .T. ) ;
#7323=VERTEX_POINT ( 'NONE', #12322 ) ;
#7324=ORIENTED_EDGE ( 'NONE', *, *, #532, .T. ) ;
#7326=ORIENTED_EDGE ( 'NONE', *, *, #6680, .T. ) ;
#7327=EDGE_CURVE ( 'NONE', #7090, #19352, #1329, .T. ) ;
#7331=EDGE_CURVE ( 'NONE', #14404, #11374, #8437, .T. ) ;
#7334=LINE ( 'NONE', #23547, #20612 ) ;
#7336=EDGE_CURVE ( 'NONE', #22817, #5616, #10926, .T. ) ;
#7337=DIRECTION ( 'NONE',  ( 0.000000000000000000, 0.000000000000000000, 1.000000000000000000 ) ) ;
#7340=CIRCLE ( 'NONE', #12341, 0.4999999999999993339 ) ;
#7341=DIRECTION ( 'NONE',  ( 0.000000000000000000, 0.000000000000000000, 1.000000000000000000 ) ) ;
#7348=DIRECTION ( 'NONE',  ( 0.000000000000000000, 0.000000000000000000, 1.000000000000000000 ) ) ;
#7350=DIRECTION ( 'NONE',  ( 0.9980267284282714479, -0.06279051952931540004, 0.000000000000000000 ) ) ;
#7352=ORIENTED_EDGE ( 'NONE', *, *, #21065, .T. ) ;
#7353=DIRECTION ( 'NONE',  ( 1.000000000000000000, 0.000000000000000000, 0.000000000000000000 ) ) ;
#7359=CARTESIAN_POINT ( 'NONE',  ( -30.85476721088030061, -3.897863563849544466, -6.500000000000000000 ) ) ;
#7360=VERTEX_POINT ( 'NONE', #14303 ) ;
#7362=CARTESIAN_POINT ( 'NONE',  ( 12.78762572734037484, -28.34936733434209444, -6.500000000000000000 ) ) ;
#7363=EDGE_CURVE ( 'NONE', #23296, #6393, #492, .T. ) ;
#7365=DIRECTION ( 'NONE',  ( 1.000000000000000000, 0.000000000000000000, 0.000000000000000000 ) ) ;
#7383=EDGE_LOOP ( 'NONE', ( #16892, #2588, #1981, #13973 ) ) ;
#7385=DIRECTION ( 'NONE',  ( 0.000000000000000000, 0.000000000000000000, 1.000000000000000000 ) ) ;
#7386=CYLINDRICAL_SURFACE ( 'NONE', #4696, 31.10000000000000142 ) ;
#7388=DIRECTION ( 'NONE',  ( -0.000000000000000000, -0.000000000000000000, 1.000000000000000000 ) ) ;
#7391=ADVANCED_FACE ( 'NONE', ( #6689 ), #692, .F. ) ;
#7392=EDGE_CURVE ( 'NONE', #8164, #19322, #436, .T. ) ;
#7393=CARTESIAN_POINT ( 'NONE',  ( 19.43607991388988765, 24.27856662945500688, 1.000000000000000000 ) ) ;
#7394=DIRECTION ( 'NONE',  ( 0.000000000000000000, -0.000000000000000000, 1.000000000000000000 ) ) ;
#7396=DIRECTION ( 'NONE',  ( 1.000000000000000000, 0.000000000000000000, 0.000000000000000000 ) ) ;
#7402=CARTESIAN_POINT ( 'NONE',  ( -24.86329371854788661, -18.68225429291705098, -6.500000000000000000 ) ) ;
#7414=EDGE_LOOP ( 'NONE', ( #2205, #18139, #25306, #7583 ) ) ;
#7423=CARTESIAN_POINT ( 'NONE',  ( 5.827558883615830965, -30.54913349766226105, -6.500000000000000000 ) ) ;
#7424=DIRECTION ( 'NONE',  ( 0.8763066800438640280, -0.4817536741017146018, 0.000000000000000000 ) ) ;
#7432=DIRECTION ( 'NONE',  ( 0.000000000000000000, 0.000000000000000000, 1.000000000000000000 ) ) ;
#7434=CARTESIAN_POINT ( 'NONE',  ( 23.64116323484232751, -20.20656826142281659, 1.000000000000000000 ) ) ;
#7435=CARTESIAN_POINT ( 'NONE',  ( 14.54246377227358877, 27.49048467073853175, -2.750000000000000000 ) ) ;
#7439=LINE ( 'NONE', #15427, #18375 ) ;
#7440=DIRECTION ( 'NONE',  ( 1.000000000000000000, 0.000000000000000000, 0.000000000000000000 ) ) ;
#7441=ORIENTED_EDGE ( 'NONE', *, *, #4104, .T. ) ;
#7442=EDGE_CURVE ( 'NONE', #4853, #18321, #8656, .T. ) ;
#7443=EDGE_LOOP ( 'NONE', ( #21989, #15425, #12232, #15814 ) ) ;
#7444=EDGE_CURVE ( 'NONE', #2906, #18910, #18218, .T. ) ;
#7445=AXIS2_PLACEMENT_3D ( 'NONE', #21719, #6027, #17545 ) ;
#7450=CARTESIAN_POINT ( 'NONE',  ( -25.16042852506104666, -18.28012134629567598, -6.500000000000000000 ) ) ;
#7452=DIRECTION ( 'NONE',  ( 1.000000000000000000, 0.000000000000000000, 0.000000000000000000 ) ) ;
#7456=CARTESIAN_POINT ( 'NONE',  ( 0.000000000000000000, 0.000000000000000000, 1.000000000000000000 ) ) ;
#7460=AXIS2_PLACEMENT_3D ( 'NONE', #23729, #22028, #8052 ) ;
#7461=CARTESIAN_POINT ( 'NONE',  ( -7.734255490826573265, 30.12293631110053838, -6.500000000000000000 ) ) ;
#7463=DIRECTION ( 'NONE',  ( 0.000000000000000000, 0.000000000000000000, 1.000000000000000000 ) ) ;
#7467=ADVANCED_FACE ( 'NONE', ( #13230 ), #22910, .T. ) ;
#7468=DIRECTION ( 'NONE',  ( 1.000000000000000000, 0.000000000000000000, 0.000000000000000000 ) ) ;
#7472=VERTEX_POINT ( 'NONE', #4995 ) ;
#7473=CARTESIAN_POINT ( 'NONE',  ( 31.00322564728514507, 2.451530025009026392, 1.000000000000000000 ) ) ;
#7474=VERTEX_POINT ( 'NONE', #25378 ) ;
#7477=ORIENTED_EDGE ( 'NONE', *, *, #22102, .F. ) ;
#7479=ORIENTED_EDGE ( 'NONE', *, *, #19066, .T. ) ;
#7480=DIRECTION ( 'NONE',  ( 1.000000000000000000, 0.000000000000000000, 0.000000000000000000 ) ) ;
#7481=EDGE_CURVE ( 'NONE', #16527, #22953, #23868, .T. ) ;
#7482=AXIS2_PLACEMENT_3D ( 'NONE', #8638, #16616, #4725 ) ;
#7486=AXIS2_PLACEMENT_3D ( 'NONE', #22762, #6663, #16495 ) ;
#7494=CIRCLE ( 'NONE', #16281, 31.10000000000000142 ) ;
#7496=ORIENTED_EDGE ( 'NONE', *, *, #14702, .T. ) ;
#7498=VECTOR ( 'NONE', #17256, 1000.000000000000000 ) ;
#7501=CARTESIAN_POINT ( 'NONE',  ( 30.85476721088025442, -3.897863563849982782, -6.500000000000000000 ) ) ;
#7502=CIRCLE ( 'NONE', #22118, 0.5000000000000005551 ) ;
#7508=CARTESIAN_POINT ( 'NONE',  ( 0.000000000000000000, 0.000000000000000000, -6.500000000000000000 ) ) ;
#7509=VECTOR ( 'NONE', #15840, 1000.000000000000000 ) ;
#7514=AXIS2_PLACEMENT_3D ( 'NONE', #20688, #6687, #1071 ) ;
#7521=VECTOR ( 'NONE', #3321, 1000.000000000000000 ) ;
#7526=CARTESIAN_POINT ( 'NONE',  ( -30.85476721088030061, -3.897863563849544466, 1.000000000000000000 ) ) ;
#7528=CYLINDRICAL_SURFACE ( 'NONE', #800, 31.10000000000000142 ) ;
#7536=LINE ( 'NONE', #17479, #1246 ) ;
#7539=EDGE_CURVE ( 'NONE', #7580, #12699, #20115, .T. ) ;
#7543=ORIENTED_EDGE ( 'NONE', *, *, #8244, .F. ) ;
#7545=EDGE_CURVE ( 'NONE', #25452, #5651, #11343, .T. ) ;
#7549=CIRCLE ( 'NONE', #12138, 0.4999999999999997224 ) ;
#7551=ADVANCED_FACE ( 'NONE', ( #3415 ), #23288, .T. ) ;
#7552=AXIS2_PLACEMENT_3D ( 'NONE', #8863, #22849, #4923 ) ;
#7553=CIRCLE ( 'NONE', #4626, 0.4999999999999993894 ) ;
#7557=FACE_OUTER_BOUND ( 'NONE', #18946, .T. ) ;
#7558=CIRCLE ( 'NONE', #5047, 30.10000000000000142 ) ;
#7560=FACE_OUTER_BOUND ( 'NONE', #6321, .T. ) ;
#7567=DIRECTION ( 'NONE',  ( 0.000000000000000000, -0.000000000000000000, -1.000000000000000000 ) ) ;
#7573=ORIENTED_EDGE ( 'NONE', *, *, #2294, .T. ) ;
#7575=CARTESIAN_POINT ( 'NONE',  ( 17.87326343783943017, 25.45105997952919097, -2.750000000000000000 ) ) ;
#7579=CIRCLE ( 'NONE', #8402, 0.5000000000000003331 ) ;
#7580=VERTEX_POINT ( 'NONE', #3279 ) ;
#7581=EDGE_CURVE ( 'NONE', #1055, #17423, #6752, .T. ) ;
#7582=VERTEX_POINT ( 'NONE', #12841 ) ;
#7583=ORIENTED_EDGE ( 'NONE', *, *, #16902, .T. ) ;
#7584=ORIENTED_EDGE ( 'NONE', *, *, #10727, .T. ) ;
#7585=DIRECTION ( 'NONE',  ( 1.000000000000000000, 0.000000000000000000, 0.000000000000000000 ) ) ;
#7586=AXIS2_PLACEMENT_3D ( 'NONE', #2965, #16697, #6757 ) ;
#7587=CARTESIAN_POINT ( 'NONE',  ( 0.000000000000000000, 0.000000000000000000, -6.500000000000000000 ) ) ;
#7589=CARTESIAN_POINT ( 'NONE',  ( -23.96296185032681336, 19.82388608118453632, -6.500000000000000000 ) ) ;
#7591=AXIS2_PLACEMENT_3D ( 'NONE', #24891, #6969, #14949 ) ;
#7594=CIRCLE ( 'NONE', #24736, 31.10000000000000142 ) ;
#7596=VECTOR ( 'NONE', #21353, 1000.000000000000000 ) ;
#7600=CARTESIAN_POINT ( 'NONE',  ( 0.000000000000000000, 0.000000000000000000, -6.500000000000000000 ) ) ;
#7601=DIRECTION ( 'NONE',  ( 0.000000000000000000, 0.000000000000000000, -1.000000000000000000 ) ) ;
#7604=AXIS2_PLACEMENT_3D ( 'NONE', #19723, #17384, #5222 ) ;
#7607=CARTESIAN_POINT ( 'NONE',  ( -14.54246377227319442, 27.49048467073874491, -2.750000000000000000 ) ) ;
#7608=VERTEX_POINT ( 'NONE', #11394 ) ;
#7611=AXIS2_PLACEMENT_3D ( 'NONE', #25365, #9538, #19598 ) ;
#7617=CARTESIAN_POINT ( 'NONE',  ( 28.72825533807124287, -11.91206721063061913, -6.500000000000000000 ) ) ;
#7618=AXIS2_PLACEMENT_3D ( 'NONE', #2865, #17382, #3633 ) ;
#7619=ADVANCED_FACE ( 'NONE', ( #23940 ), #25766, .F. ) ;
#7622=CARTESIAN_POINT ( 'NONE',  ( -17.78012134629558716, 25.16042852506110705, -6.500000000000000000 ) ) ;
#7623=EDGE_CURVE ( 'NONE', #7162, #14349, #3030, .T. ) ;
#7625=DIRECTION ( 'NONE',  ( 1.000000000000000000, 0.000000000000000000, 0.000000000000000000 ) ) ;
#7628=CARTESIAN_POINT ( 'NONE',  ( -5.827558883615604479, 30.54913349766230724, 1.000000000000000000 ) ) ;
#7631=EDGE_CURVE ( 'NONE', #4731, #19766, #6778, .T. ) ;
#7632=CIRCLE ( 'NONE', #20588, 0.5000000000000000000 ) ;
#7635=ORIENTED_EDGE ( 'NONE', *, *, #10998, .F. ) ;
#7636=ORIENTED_EDGE ( 'NONE', *, *, #16361, .F. ) ;
#7638=ORIENTED_EDGE ( 'NONE', *, *, #11592, .T. ) ;
#7639=CARTESIAN_POINT ( 'NONE',  ( -25.45105997952899912, 17.87326343783971083, -2.750000000000000000 ) ) ;
#7641=DIRECTION ( 'NONE',  ( 0.9822872507286911636, 0.1873813145857119722, 0.000000000000000000 ) ) ;
#7642=ORIENTED_EDGE ( 'NONE', *, *, #21118, .T. ) ;
#7645=DIRECTION ( 'NONE',  ( 1.000000000000000000, 0.000000000000000000, 0.000000000000000000 ) ) ;
#7646=ORIENTED_EDGE ( 'NONE', *, *, #4698, .F. ) ;
#7649=DIRECTION ( 'NONE',  ( 1.000000000000000000, 0.000000000000000000, 0.000000000000000000 ) ) ;
#7658=CARTESIAN_POINT ( 'NONE',  ( 0.000000000000000000, 0.000000000000000000, -6.500000000000000000 ) ) ;
#7659=VECTOR ( 'NONE', #3119, 1000.000000000000000 ) ;
#7669=ORIENTED_EDGE ( 'NONE', *, *, #18367, .T. ) ;
#7673=VERTEX_POINT ( 'NONE', #11517 ) ;
#7675=CARTESIAN_POINT ( 'NONE',  ( -27.49048467073863833, -14.54246377227340048, 1.000000000000000000 ) ) ;
#7678=FACE_OUTER_BOUND ( 'NONE', #6418, .T. ) ;
#7684=EDGE_CURVE ( 'NONE', #9053, #7861, #11361, .T. ) ;
#7687=ADVANCED_FACE ( 'NONE', ( #3663 ), #15587, .F. ) ;
#7691=EDGE_CURVE ( 'NONE', #9386, #20150, #17221, .T. ) ;
#7692=CARTESIAN_POINT ( 'NONE',  ( -19.82388608118446527, -23.96296185032687376, -6.500000000000000000 ) ) ;
#7693=DIRECTION ( 'NONE',  ( 1.000000000000000000, 0.000000000000000000, 0.000000000000000000 ) ) ;
#7696=VERTEX_POINT ( 'NONE', #11641 ) ;
#7697=DIRECTION ( 'NONE',  ( 0.000000000000000000, 0.000000000000000000, 1.000000000000000000 ) ) ;
#7700=FACE_OUTER_BOUND ( 'NONE', #19653, .T. ) ;
#7703=VERTEX_POINT ( 'NONE', #21716 ) ;
#7706=LINE ( 'NONE', #9912, #24219 ) ;
#7707=DIRECTION ( 'NONE',  ( 0.9510565162951586382, 0.3090169943749320192, 0.000000000000000000 ) ) ;
#7712=EDGE_LOOP ( 'NONE', ( #8550, #12792, #10850, #6843 ) ) ;
#7713=CARTESIAN_POINT ( 'NONE',  ( -29.41953157733101065, -10.08469938919468945, -2.750000000000000000 ) ) ;
#7714=FACE_OUTER_BOUND ( 'NONE', #24075, .T. ) ;
#7716=ADVANCED_FACE ( 'NONE', ( #19616 ), #23422, .T. ) ;
#7725=FACE_OUTER_BOUND ( 'NONE', #17657, .T. ) ;
#7732=CARTESIAN_POINT ( 'NONE',  ( 0.000000000000000000, 0.000000000000000000, -6.500000000000000000 ) ) ;
#7734=EDGE_CURVE ( 'NONE', #10526, #16921, #9283, .T. ) ;
#7737=EDGE_CURVE ( 'NONE', #14144, #13306, #1854, .T. ) ;
#7738=VERTEX_POINT ( 'NONE', #14514 ) ;
#7744=VERTEX_POINT ( 'NONE', #2357 ) ;
#7748=CYLINDRICAL_SURFACE ( 'NONE', #13845, 0.5000000000000004441 ) ;
#7753=CARTESIAN_POINT ( 'NONE',  ( 11.44867358849351113, 28.91604871112461339, -6.500000000000000000 ) ) ;
#7757=DIRECTION ( 'NONE',  ( -0.6845471059286831750, 0.7289686274214168815, 0.000000000000000000 ) ) ;
#7759=EDGE_CURVE ( 'NONE', #19902, #8252, #20129, .T. ) ;
#7760=VERTEX_POINT ( 'NONE', #18190 ) ;
#7763=EDGE_LOOP ( 'NONE', ( #1803, #3619, #18452, #17108 ) ) ;
#7770=EDGE_CURVE ( 'NONE', #4455, #10488, #8028, .T. ) ;
#7771=DIRECTION ( 'NONE',  ( -0.000000000000000000, 0.000000000000000000, 1.000000000000000000 ) ) ;
#7785=LINE ( 'NONE', #1787, #13452 ) ;
#7791=VERTEX_POINT ( 'NONE', #20526 ) ;
#7797=CYLINDRICAL_SURFACE ( 'NONE', #21372, 0.5000000000000004441 ) ;
#7800=ORIENTED_EDGE ( 'NONE', *, *, #7863, .F. ) ;
#7801=ORIENTED_EDGE ( 'NONE', *, *, #24725, .T. ) ;
#7807=CARTESIAN_POINT ( 'NONE',  ( -26.25859848311247902, 16.66421332384710752, -6.500000000000000000 ) ) ;
#7810=CARTESIAN_POINT ( 'NONE',  ( 0.000000000000000000, 0.000000000000000000, 1.000000000000000000 ) ) ;
#7814=DIRECTION ( 'NONE',  ( 0.000000000000000000, -0.000000000000000000, 1.000000000000000000 ) ) ;
#7821=DIRECTION ( 'NONE',  ( 0.000000000000000000, 0.000000000000000000, 1.000000000000000000 ) ) ;
#7823=ORIENTED_EDGE ( 'NONE', *, *, #21096, .T. ) ;
#7825=DIRECTION ( 'NONE',  ( 0.000000000000000000, 0.000000000000000000, 1.000000000000000000 ) ) ;
#7832=LINE ( 'NONE', #23925, #11378 ) ;
#7835=CYLINDRICAL_SURFACE ( 'NONE', #1833, 0.5000000000000004441 ) ;
#7841=DIRECTION ( 'NONE',  ( 1.000000000000000000, 0.000000000000000000, 0.000000000000000000 ) ) ;
#7846=CARTESIAN_POINT ( 'NONE',  ( -7.734255490827218971, -30.12293631110037140, 1.000000000000000000 ) ) ;
#7850=CIRCLE ( 'NONE', #5354, 31.10000000000000142 ) ;
#7851=CYLINDRICAL_SURFACE ( 'NONE', #4137, 0.5000000000000004441 ) ;
#7852=DIRECTION ( 'NONE',  ( 1.000000000000000000, 0.000000000000000000, 0.000000000000000000 ) ) ;
#7855=ORIENTED_EDGE ( 'NONE', *, *, #21496, .T. ) ;
#7856=ORIENTED_EDGE ( 'NONE', *, *, #4104, .F. ) ;
#7857=DIRECTION ( 'NONE',  ( 0.000000000000000000, -0.000000000000000000, 1.000000000000000000 ) ) ;
#7861=VERTEX_POINT ( 'NONE', #6277 ) ;
#7862=DIRECTION ( 'NONE',  ( 0.000000000000000000, -0.000000000000000000, 1.000000000000000000 ) ) ;
#7863=EDGE_CURVE ( 'NONE', #2607, #22740, #13870, .T. ) ;
#7865=EDGE_CURVE ( 'NONE', #6294, #7134, #19292, .T. ) ;
#7867=CARTESIAN_POINT ( 'NONE',  ( -20.78941499438242246, -22.67092431280570963, -6.500000000000000000 ) ) ;
#7876=VECTOR ( 'NONE', #1429, 1000.000000000000000 ) ;
#7881=ORIENTED_EDGE ( 'NONE', *, *, #7539, .T. ) ;
#7882=ORIENTED_EDGE ( 'NONE', *, *, #10714, .F. ) ;
#7884=VERTEX_POINT ( 'NONE', #16097 ) ;
#7889=CARTESIAN_POINT ( 'NONE',  ( -30.24338421796786847, -7.248980000273999025, 1.000000000000000000 ) ) ;
#7890=ORIENTED_EDGE ( 'NONE', *, *, #7327, .T. ) ;
#7891=ORIENTED_EDGE ( 'NONE', *, *, #13499, .T. ) ;
#7894=CIRCLE ( 'NONE', #9153, 31.10000000000000142 ) ;
#7897=CARTESIAN_POINT ( 'NONE',  ( -28.34936733434213707, -12.78762572734027181, -2.750000000000000000 ) ) ;
#7899=CARTESIAN_POINT ( 'NONE',  ( 1.952785157361432100, -31.03863125411925949, 1.000000000000000000 ) ) ;
#7900=DIRECTION ( 'NONE',  ( 1.000000000000000000, 0.000000000000000000, 0.000000000000000000 ) ) ;
#7904=CIRCLE ( 'NONE', #19177, 31.10000000000000142 ) ;
#7907=AXIS2_PLACEMENT_3D ( 'NONE', #25818, #12346, #7900 ) ;
#7908=DIRECTION ( 'NONE',  ( 0.000000000000000000, 0.000000000000000000, 1.000000000000000000 ) ) ;
#7909=VECTOR ( 'NONE', #25804, 1000.000000000000000 ) ;
#7917=CARTESIAN_POINT ( 'NONE',  ( 0.000000000000000000, 0.000000000000000000, -6.500000000000000000 ) ) ;
#7923=ORIENTED_EDGE ( 'NONE', *, *, #15852, .F. ) ;
#7926=CARTESIAN_POINT ( 'NONE',  ( -19.82388608118395013, 23.96296185032730364, -6.500000000000000000 ) ) ;
#7927=CIRCLE ( 'NONE', #22551, 31.10000000000000142 ) ;
#7929=CARTESIAN_POINT ( 'NONE',  ( 0.000000000000000000, 0.000000000000000000, -6.500000000000000000 ) ) ;
#7931=ORIENTED_EDGE ( 'NONE', *, *, #8670, .T. ) ;
#7938=VECTOR ( 'NONE', #13595, 1000.000000000000000 ) ;
#7939=CYLINDRICAL_SURFACE ( 'NONE', #14190, 0.5000000000000004441 ) ;
#7941=AXIS2_PLACEMENT_3D ( 'NONE', #9692, #15709, #21333 ) ;
#7942=VECTOR ( 'NONE', #5401, 1000.000000000000000 ) ;
#7944=CARTESIAN_POINT ( 'NONE',  ( -9.110428525061097460, -29.57785765677920509, -6.500000000000000000 ) ) ;
#7945=DIRECTION ( 'NONE',  ( 1.000000000000000000, 0.000000000000000000, 0.000000000000000000 ) ) ;
#7947=CARTESIAN_POINT ( 'NONE',  ( -1.453535542772826039, -31.06601413805601908, -2.750000000000000000 ) ) ;
#7953=AXIS2_PLACEMENT_3D ( 'NONE', #21710, #11634, #9166 ) ;
#7957=CARTESIAN_POINT ( 'NONE',  ( 11.44867358849351113, 28.91604871112461339, -6.500000000000000000 ) ) ;
#7959=DIRECTION ( 'NONE',  ( 1.000000000000000000, 0.000000000000000000, 0.000000000000000000 ) ) ;
#7963=EDGE_LOOP ( 'NONE', ( #6422, #10231, #18525, #15208 ) ) ;
#7964=CIRCLE ( 'NONE', #19640, 0.4999999999999991673 ) ;
#7966=ORIENTED_EDGE ( 'NONE', *, *, #13529, .T. ) ;
#7968=ORIENTED_EDGE ( 'NONE', *, *, #10435, .F. ) ;
#7969=DIRECTION ( 'NONE',  ( 1.000000000000000000, 0.000000000000000000, 0.000000000000000000 ) ) ;
#7971=DIRECTION ( 'NONE',  ( 0.000000000000000000, 0.000000000000000000, 1.000000000000000000 ) ) ;
#7972=VECTOR ( 'NONE', #8536, 1000.000000000000000 ) ;
#7980=EDGE_CURVE ( 'NONE', #11427, #6457, #18472, .T. ) ;
#7981=LINE ( 'NONE', #14393, #5881 ) ;
#7982=AXIS2_PLACEMENT_3D ( 'NONE', #9578, #17951, #14028 ) ;
#7987=DIRECTION ( 'NONE',  ( 1.000000000000000000, 0.000000000000000000, 0.000000000000000000 ) ) ;
#7989=CIRCLE ( 'NONE', #15500, 0.5000000000000003331 ) ;
#7991=AXIS2_PLACEMENT_3D ( 'NONE', #8328, #10544, #625 ) ;
#7992=DIRECTION ( 'NONE',  ( 0.000000000000000000, 0.000000000000000000, 1.000000000000000000 ) ) ;
#7994=FACE_OUTER_BOUND ( 'NONE', #2657, .T. ) ;
#7995=FACE_OUTER_BOUND ( 'NONE', #9671, .T. ) ;
#7996=VERTEX_POINT ( 'NONE', #25099 ) ;
#7997=CARTESIAN_POINT ( 'NONE',  ( 26.25859848311259981, -16.66421332384692278, -6.500000000000000000 ) ) ;
#7998=VERTEX_POINT ( 'NONE', #3004 ) ;
#8000=ORIENTED_EDGE ( 'NONE', *, *, #12007, .F. ) ;
#8004=ORIENTED_EDGE ( 'NONE', *, *, #11799, .F. ) ;
#8005=LINE ( 'NONE', #289, #23020 ) ;
#8007=ORIENTED_EDGE ( 'NONE', *, *, #4324, .T. ) ;
#8010=CIRCLE ( 'NONE', #17623, 0.5000000000000001110 ) ;
#8013=CARTESIAN_POINT ( 'NONE',  ( -16.66421332384701515, -26.25859848311253941, 1.000000000000000000 ) ) ;
#8015=DIRECTION ( 'NONE',  ( 0.000000000000000000, 0.000000000000000000, 1.000000000000000000 ) ) ;
#8020=EDGE_CURVE ( 'NONE', #5409, #9972, #15155, .T. ) ;
#8027=AXIS2_PLACEMENT_3D ( 'NONE', #22751, #21047, #3122 ) ;
#8028=CIRCLE ( 'NONE', #4691, 31.10000000000000142 ) ;
#8036=ORIENTED_EDGE ( 'NONE', *, *, #2436, .F. ) ;
#8037=VECTOR ( 'NONE', #349, 1000.000000000000000 ) ;
#8039=ORIENTED_EDGE ( 'NONE', *, *, #21096, .F. ) ;
#8040=DIRECTION ( 'NONE',  ( 1.000000000000000000, 0.000000000000000000, 0.000000000000000000 ) ) ;
#8043=CIRCLE ( 'NONE', #8468, 0.5000000000000000000 ) ;
#8046=ADVANCED_FACE ( 'NONE', ( #18828 ), #13324, .T. ) ;
#8048=AXIS2_PLACEMENT_3D ( 'NONE', #22668, #10738, #19927 ) ;
#8050=DIRECTION ( 'NONE',  ( -0.000000000000000000, 0.000000000000000000, 1.000000000000000000 ) ) ;
#8052=DIRECTION ( 'NONE',  ( 1.000000000000000000, 0.000000000000000000, 0.000000000000000000 ) ) ;
#8055=ADVANCED_FACE ( 'NONE', ( #16881 ), #5221, .F. ) ;
#8060=ORIENTED_EDGE ( 'NONE', *, *, #16115, .F. ) ;
#8063=EDGE_CURVE ( 'NONE', #6029, #13686, #943, .T. ) ;
#8065=ORIENTED_EDGE ( 'NONE', *, *, #15086, .T. ) ;
#8067=ADVANCED_FACE ( 'NONE', ( #13199 ), #1157, .F. ) ;
#8068=CIRCLE ( 'NONE', #12656, 0.4999999999999997780 ) ;
#8069=DIRECTION ( 'NONE',  ( 0.000000000000000000, 0.000000000000000000, 1.000000000000000000 ) ) ;
#8077=CIRCLE ( 'NONE', #6811, 0.5000000000000007772 ) ;
#8083=DIRECTION ( 'NONE',  ( 0.000000000000000000, 0.000000000000000000, 1.000000000000000000 ) ) ;
#8085=LINE ( 'NONE', #7947, #6617 ) ;
#8092=CYLINDRICAL_SURFACE ( 'NONE', #22073, 0.5000000000000004441 ) ;
#8095=CARTESIAN_POINT ( 'NONE',  ( 0.000000000000000000, 0.000000000000000000, 1.000000000000000000 ) ) ;
#8096=ORIENTED_EDGE ( 'NONE', *, *, #136, .F. ) ;
#8098=DIRECTION ( 'NONE',  ( 0.000000000000000000, -0.000000000000000000, 1.000000000000000000 ) ) ;
#8100=ADVANCED_FACE ( 'NONE', ( #24846 ), #22758, .F. ) ;
#8102=ORIENTED_EDGE ( 'NONE', *, *, #13932, .F. ) ;
#8104=AXIS2_PLACEMENT_3D ( 'NONE', #8741, #6786, #14771 ) ;
#8106=ORIENTED_EDGE ( 'NONE', *, *, #1716, .F. ) ;
#8109=EDGE_CURVE ( 'NONE', #7744, #16500, #3858, .T. ) ;
#8110=DIRECTION ( 'NONE',  ( -0.000000000000000000, -0.000000000000000000, 1.000000000000000000 ) ) ;
#8111=CARTESIAN_POINT ( 'NONE',  ( 27.25313774936419620, 14.98253926456328244, 1.000000000000000000 ) ) ;
#8118=CARTESIAN_POINT ( 'NONE',  ( -27.64012133169333651, -13.24173596767349359, -6.500000000000000000 ) ) ;
#8120=DIRECTION ( 'NONE',  ( 0.000000000000000000, 0.000000000000000000, 1.000000000000000000 ) ) ;
#8122=DIRECTION ( 'NONE',  ( 1.000000000000000000, 0.000000000000000000, 0.000000000000000000 ) ) ;
#8129=CARTESIAN_POINT ( 'NONE',  ( 8.217531866530997320, -29.99470236596036088, -2.750000000000000000 ) ) ;
#8130=ORIENTED_EDGE ( 'NONE', *, *, #16516, .T. ) ;
#8131=EDGE_CURVE ( 'NONE', #16191, #14853, #10954, .T. ) ;
#8132=ADVANCED_FACE ( 'NONE', ( #1939 ), #9658, .F. ) ;
#8135=ORIENTED_EDGE ( 'NONE', *, *, #642, .T. ) ;
#8139=DIRECTION ( 'NONE',  ( 0.000000000000000000, -0.000000000000000000, 1.000000000000000000 ) ) ;
#8143=DIRECTION ( 'NONE',  ( 1.000000000000000000, 0.000000000000000000, 0.000000000000000000 ) ) ;
#8145=DIRECTION ( 'NONE',  ( 1.000000000000000000, 0.000000000000000000, 0.000000000000000000 ) ) ;
#8146=CYLINDRICAL_SURFACE ( 'NONE', #10442, 0.5000000000000004441 ) ;
#8149=CARTESIAN_POINT ( 'NONE',  ( -17.08421000182741878, 25.98730014090460116, -2.750000000000000000 ) ) ;
#8154=EDGE_LOOP ( 'NONE', ( #21210, #23240, #16505, #6807 ) ) ;
#8156=ORIENTED_EDGE ( 'NONE', *, *, #25063, .F. ) ;
#8157=CARTESIAN_POINT ( 'NONE',  ( -30.54913349766228592, -5.827558883615738594, -6.500000000000000000 ) ) ;
#8160=DIRECTION ( 'NONE',  ( 0.000000000000000000, 0.000000000000000000, 1.000000000000000000 ) ) ;
#8163=FACE_OUTER_BOUND ( 'NONE', #23370, .T. ) ;
#8164=VERTEX_POINT ( 'NONE', #12845 ) ;
#8166=AXIS2_PLACEMENT_3D ( 'NONE', #2123, #8139, #22256 ) ;
#8167=CYLINDRICAL_SURFACE ( 'NONE', #16843, 0.5000000000000004441 ) ;
#8170=CARTESIAN_POINT ( 'NONE',  ( -29.57785765677936851, -9.610428525060582317, -6.500000000000000000 ) ) ;
#8173=AXIS2_PLACEMENT_3D ( 'NONE', #7450, #21071, #12603 ) ;
#8177=PRODUCT ( 'bezel', 'bezel', '', ( #21014 ) ) ;
#8178=FACE_OUTER_BOUND ( 'NONE', #11884, .T. ) ;
#8182=DIRECTION ( 'NONE',  ( 0.000000000000000000, 0.000000000000000000, 1.000000000000000000 ) ) ;
#8192=ORIENTED_EDGE ( 'NONE', *, *, #19852, .T. ) ;
#8193=ORIENTED_EDGE ( 'NONE', *, *, #16100, .T. ) ;
#8194=CARTESIAN_POINT ( 'NONE',  ( 21.28941499438209206, -22.67092431280601872, -6.500000000000000000 ) ) ;
#8202=ADVANCED_FACE ( 'NONE', ( #4112 ), #4250, .F. ) ;
#8203=CARTESIAN_POINT ( 'NONE',  ( 30.54913349766219710, -5.827558883616158703, -6.500000000000000000 ) ) ;
#8204=CARTESIAN_POINT ( 'NONE',  ( -17.78012134629613783, -25.16042852506070560, 1.000000000000000000 ) ) ;
#8211=CARTESIAN_POINT ( 'NONE',  ( 0.000000000000000000, 0.000000000000000000, 1.000000000000000000 ) ) ;
#8212=DIRECTION ( 'NONE',  ( 1.000000000000000000, 0.000000000000000000, 0.000000000000000000 ) ) ;
#8217=FACE_OUTER_BOUND ( 'NONE', #22251, .T. ) ;
#8222=DIRECTION ( 'NONE',  ( 0.7289686274214101092, -0.6845471059286901694, 0.000000000000000000 ) ) ;
#8226=ORIENTED_EDGE ( 'NONE', *, *, #3234, .F. ) ;
#8227=DIRECTION ( 'NONE',  ( 0.000000000000000000, 0.000000000000000000, 1.000000000000000000 ) ) ;
#8228=FACE_OUTER_BOUND ( 'NONE', #15082, .T. ) ;
#8233=EDGE_CURVE ( 'NONE', #24375, #4269, #19319, .T. ) ;
#8236=ADVANCED_FACE ( 'NONE', ( #10870 ), #326, .F. ) ;
#8240=DIRECTION ( 'NONE',  ( 0.000000000000000000, 0.000000000000000000, 1.000000000000000000 ) ) ;
#8241=FACE_OUTER_BOUND ( 'NONE', #20969, .T. ) ;
#8244=EDGE_CURVE ( 'NONE', #16170, #6260, #10967, .T. ) ;
#8247=DIRECTION ( 'NONE',  ( 0.000000000000000000, -0.000000000000000000, 1.000000000000000000 ) ) ;
#8250=CARTESIAN_POINT ( 'NONE',  ( 13.24173596767359662, -28.14012133169329388, -6.500000000000000000 ) ) ;
#8251=FACE_OUTER_BOUND ( 'NONE', #17584, .T. ) ;
#8252=VERTEX_POINT ( 'NONE', #18133 ) ;
#8258=CARTESIAN_POINT ( 'NONE',  ( -29.99470236596038220, -8.217531866530892515, -2.750000000000000000 ) ) ;
#8262=ADVANCED_FACE ( 'NONE', ( #8178 ), #17994, .F. ) ;
#8265=CARTESIAN_POINT ( 'NONE',  ( 15.41874213889396117, -27.00874656207311020, -2.750000000000000000 ) ) ;
#8267=DIRECTION ( 'NONE',  ( 0.000000000000000000, 0.000000000000000000, 1.000000000000000000 ) ) ;
#8275=AXIS2_PLACEMENT_3D ( 'NONE', #16680, #725, #8834 ) ;
#8276=EDGE_LOOP ( 'NONE', ( #13151, #17485, #6007, #14110 ) ) ;
#8277=ORIENTED_EDGE ( 'NONE', *, *, #20905, .F. ) ;
#8280=VERTEX_POINT ( 'NONE', #83 ) ;
#8281=DIRECTION ( 'NONE',  ( 0.3681245526846732008, -0.9297764858882532346, 0.000000000000000000 ) ) ;
#8284=ORIENTED_EDGE ( 'NONE', *, *, #900, .T. ) ;
#8285=AXIS2_PLACEMENT_3D ( 'NONE', #20139, #10451, #16494 ) ;
#8286=CARTESIAN_POINT ( 'NONE',  ( 1.952785157361650370, 31.03863125411924528, -6.500000000000000000 ) ) ;
#8287=ORIENTED_EDGE ( 'NONE', *, *, #23723, .F. ) ;
#8291=AXIS2_PLACEMENT_3D ( 'NONE', #18875, #21091, #16920 ) ;
#8293=DIRECTION ( 'NONE',  ( 0.000000000000000000, 0.000000000000000000, 1.000000000000000000 ) ) ;
#8296=EDGE_CURVE ( 'NONE', #21691, #9505, #23999, .T. ) ;
#8298=CIRCLE ( 'NONE', #8285, 31.10000000000000142 ) ;
#8299=CIRCLE ( 'NONE', #23754, 0.4999999999999987232 ) ;
#8303=VECTOR ( 'NONE', #8695, 1000.000000000000000 ) ;
#8304=FACE_OUTER_BOUND ( 'NONE', #3461, .T. ) ;
#8305=DIRECTION ( 'NONE',  ( -0.9921147013144768767, 0.1253332335643120576, 0.000000000000000000 ) ) ;
#8307=ORIENTED_EDGE ( 'NONE', *, *, #16598, .F. ) ;
#8311=ORIENTED_EDGE ( 'NONE', *, *, #5790, .F. ) ;
#8312=ORIENTED_EDGE ( 'NONE', *, *, #12498, .T. ) ;
#8314=DIRECTION ( 'NONE',  ( 0.000000000000000000, 0.000000000000000000, 1.000000000000000000 ) ) ;
#8315=ORIENTED_EDGE ( 'NONE', *, *, #19124, .F. ) ;
#8321=CARTESIAN_POINT ( 'NONE',  ( -31.10000000000000142, 3.257552089140643357E-13, -6.500000000000000000 ) ) ;
#8322=AXIS2_PLACEMENT_3D ( 'NONE', #975, #4771, #21102 ) ;
#8323=VECTOR ( 'NONE', #12875, 1000.000000000000000 ) ;
#8326=LINE ( 'NONE', #13697, #15524 ) ;
#8327=EDGE_CURVE ( 'NONE', #8668, #22605, #24758, .T. ) ;
#8328=CARTESIAN_POINT ( 'NONE',  ( 0.000000000000000000, 0.000000000000000000, -6.500000000000000000 ) ) ;
#8330=CARTESIAN_POINT ( 'NONE',  ( -9.110428525060477511, 29.57785765677940404, 1.000000000000000000 ) ) ;
#8336=DIRECTION ( 'NONE',  ( 1.000000000000000000, 0.000000000000000000, 0.000000000000000000 ) ) ;
#8338=DIRECTION ( 'NONE',  ( 0.000000000000000000, 0.000000000000000000, 1.000000000000000000 ) ) ;
#8339=ORIENTED_EDGE ( 'NONE', *, *, #1391, .F. ) ;
#8340=EDGE_CURVE ( 'NONE', #13787, #1315, #14329, .T. ) ;
#8343=ORIENTED_EDGE ( 'NONE', *, *, #15631, .F. ) ;
#8349=EDGE_CURVE ( 'NONE', #15624, #20629, #5143, .T. ) ;
#8350=CIRCLE ( 'NONE', #425, 0.5000000000000006661 ) ;
#8351=VERTEX_POINT ( 'NONE', #5139 ) ;
#8358=AXIS2_PLACEMENT_3D ( 'NONE', #19104, #5249, #22661 ) ;
#8364=DIRECTION ( 'NONE',  ( 0.9980267284282724471, 0.06279051952930156388, 0.000000000000000000 ) ) ;
#8367=CARTESIAN_POINT ( 'NONE',  ( -5.827558883616271501, -30.54913349766217934, -6.500000000000000000 ) ) ;
#8368=DIRECTION ( 'NONE',  ( -0.4817536741017063306, 0.8763066800438685799, 0.000000000000000000 ) ) ;
#8371=CYLINDRICAL_SURFACE ( 'NONE', #2729, 0.5000000000000004441 ) ;
#8373=EDGE_CURVE ( 'NONE', #7266, #1051, #13116, .T. ) ;
#8377=FACE_OUTER_BOUND ( 'NONE', #19731, .T. ) ;
#8378=LINE ( 'NONE', #8763, #16261 ) ;
#8380=AXIS2_PLACEMENT_3D ( 'NONE', #5719, #15674, #1428 ) ;
#8381=CIRCLE ( 'NONE', #6729, 31.10000000000000142 ) ;
#8383=ORIENTED_EDGE ( 'NONE', *, *, #18594, .T. ) ;
#8389=AXIS2_PLACEMENT_3D ( 'NONE', #3895, #9896, #18270 ) ;
#8391=ORIENTED_EDGE ( 'NONE', *, *, #22992, .F. ) ;
#8397=CARTESIAN_POINT ( 'NONE',  ( 0.000000000000000000, 0.000000000000000000, -6.500000000000000000 ) ) ;
#8400=VECTOR ( 'NONE', #5475, 1000.000000000000000 ) ;
#8401=DIRECTION ( 'NONE',  ( 0.000000000000000000, 0.000000000000000000, 1.000000000000000000 ) ) ;
#8402=AXIS2_PLACEMENT_3D ( 'NONE', #6957, #4752, #12722 ) ;
#8406=DIRECTION ( 'NONE',  ( 0.000000000000000000, 0.000000000000000000, 1.000000000000000000 ) ) ;
#8408=AXIS2_PLACEMENT_3D ( 'NONE', #25314, #5570, #21016 ) ;
#8412=VERTEX_POINT ( 'NONE', #3164 ) ;
#8415=AXIS2_PLACEMENT_3D ( 'NONE', #25282, #21363, #21219 ) ;
#8416=EDGE_LOOP ( 'NONE', ( #5325, #19115, #15079, #20768 ) ) ;
#8421=VERTEX_POINT ( 'NONE', #22916 ) ;
#8422=DIRECTION ( 'NONE',  ( -0.5358267949790012086, -0.8443279255020122998, 0.000000000000000000 ) ) ;
#8425=DIRECTION ( 'NONE',  ( 0.06279051952932236669, 0.9980267284282710039, 0.000000000000000000 ) ) ;
#8429=CARTESIAN_POINT ( 'NONE',  ( 0.000000000000000000, 0.000000000000000000, -6.500000000000000000 ) ) ;
#8430=CIRCLE ( 'NONE', #18458, 0.4999999999999983902 ) ;
#8432=LINE ( 'NONE', #20055, #25434 ) ;
#8434=CIRCLE ( 'NONE', #18873, 0.5000000000000003331 ) ;
#8436=VECTOR ( 'NONE', #6140, 1000.000000000000000 ) ;
#8437=CIRCLE ( 'NONE', #24306, 31.10000000000000142 ) ;
#8442=CIRCLE ( 'NONE', #20556, 0.5000000000000011102 ) ;
#8463=ADVANCED_FACE ( 'NONE', ( #25001 ), #17302, .T. ) ;
#8466=DIRECTION ( 'NONE',  ( 0.000000000000000000, -0.000000000000000000, 1.000000000000000000 ) ) ;
#8468=AXIS2_PLACEMENT_3D ( 'NONE', #6129, #21959, #12144 ) ;
#8470=DIRECTION ( 'NONE',  ( 1.387778780781445044E-14, 1.000000000000000000, 0.000000000000000000 ) ) ;
#8477=CARTESIAN_POINT ( 'NONE',  ( 0.000000000000000000, 0.000000000000000000, 1.000000000000000000 ) ) ;
#8478=VERTEX_POINT ( 'NONE', #13368 ) ;
#8480=DIRECTION ( 'NONE',  ( -0.9685831611286319642, -0.2486898871648515197, 0.000000000000000000 ) ) ;
#8486=ORIENTED_EDGE ( 'NONE', *, *, #12733, .T. ) ;
#8488=CIRCLE ( 'NONE', #16861, 31.10000000000000142 ) ;
#8489=ORIENTED_EDGE ( 'NONE', *, *, #2510, .T. ) ;
#8496=EDGE_CURVE ( 'NONE', #25184, #6156, #13623, .T. ) ;
#8498=EDGE_CURVE ( 'NONE', #14582, #25359, #21590, .T. ) ;
#8499=ADVANCED_FACE ( 'NONE', ( #9559 ), #3669, .T. ) ;
#8508=CARTESIAN_POINT ( 'NONE',  ( 0.000000000000000000, 0.000000000000000000, 1.000000000000000000 ) ) ;
#8511=DIRECTION ( 'NONE',  ( 1.000000000000000000, 0.000000000000000000, 0.000000000000000000 ) ) ;
#8513=DIRECTION ( 'NONE',  ( 1.000000000000000000, 0.000000000000000000, 0.000000000000000000 ) ) ;
#8514=DIRECTION ( 'NONE',  ( 0.000000000000000000, 0.000000000000000000, 1.000000000000000000 ) ) ;
#8517=ORIENTED_EDGE ( 'NONE', *, *, #4897, .F. ) ;
#8519=CARTESIAN_POINT ( 'NONE',  ( 31.00322564728514507, 2.451530025009026836, -2.750000000000000000 ) ) ;
#8520=ORIENTED_EDGE ( 'NONE', *, *, #12071, .F. ) ;
#8521=ORIENTED_EDGE ( 'NONE', *, *, #7238, .T. ) ;
#8522=ORIENTED_EDGE ( 'NONE', *, *, #19673, .F. ) ;
#8523=ORIENTED_EDGE ( 'NONE', *, *, #13932, .T. ) ;
#8524=ADVANCED_FACE ( 'NONE', ( #25771 ), #17805, .F. ) ;
#8525=EDGE_LOOP ( 'NONE', ( #19459, #14079, #5235, #18117 ) ) ;
#8527=CARTESIAN_POINT ( 'NONE',  ( 10.08469938919499320, 29.41953157733090762, -2.750000000000000000 ) ) ;
#8536=DIRECTION ( 'NONE',  ( -0.000000000000000000, -0.000000000000000000, -1.000000000000000000 ) ) ;
#8537=CARTESIAN_POINT ( 'NONE',  ( 0.000000000000000000, 0.000000000000000000, -6.500000000000000000 ) ) ;
#8540=ADVANCED_FACE ( 'NONE', ( #7995 ), #10074, .F. ) ;
#8542=CARTESIAN_POINT ( 'NONE',  ( 22.32573188046920265, 21.65113613650335367, -6.500000000000000000 ) ) ;
#8548=ORIENTED_EDGE ( 'NONE', *, *, #8819, .F. ) ;
#8550=ORIENTED_EDGE ( 'NONE', *, *, #10784, .F. ) ;
#8554=CARTESIAN_POINT ( 'NONE',  ( -31.03863125411922752, 1.952785157361987878, 1.000000000000000000 ) ) ;
#8555=CYLINDRICAL_SURFACE ( 'NONE', #11095, 0.5000000000000004441 ) ;
#8556=VERTEX_POINT ( 'NONE', #4055 ) ;
#8567=DIRECTION ( 'NONE',  ( -0.000000000000000000, -0.000000000000000000, 1.000000000000000000 ) ) ;
#8571=ADVANCED_FACE ( 'NONE', ( #3940 ), #16103, .F. ) ;
#8580=LINE ( 'NONE', #6995, #23430 ) ;
#8586=CARTESIAN_POINT ( 'NONE',  ( -19.82388608118446527, -23.96296185032687376, 1.000000000000000000 ) ) ;
#8591=DIRECTION ( 'NONE',  ( -0.000000000000000000, 0.000000000000000000, 1.000000000000000000 ) ) ;
#8595=DIRECTION ( 'NONE',  ( -0.7289686274214034478, 0.6845471059286972748, 0.000000000000000000 ) ) ;
#8596=DIRECTION ( 'NONE',  ( 1.000000000000000000, 0.000000000000000000, 0.000000000000000000 ) ) ;
#8599=ORIENTED_EDGE ( 'NONE', *, *, #24415, .T. ) ;
#8603=VERTEX_POINT ( 'NONE', #407 ) ;
#8608=ORIENTED_EDGE ( 'NONE', *, *, #19673, .T. ) ;
#8616=CARTESIAN_POINT ( 'NONE',  ( 17.87326343783935911, -25.45105997952923715, 1.000000000000000000 ) ) ;
#8627=CARTESIAN_POINT ( 'NONE',  ( 0.000000000000000000, 0.000000000000000000, 1.000000000000000000 ) ) ;
#8628=DIRECTION ( 'NONE',  ( 0.000000000000000000, 0.000000000000000000, 1.000000000000000000 ) ) ;
#8633=DIRECTION ( 'NONE',  ( 1.000000000000000000, 0.000000000000000000, 0.000000000000000000 ) ) ;
#8634=CARTESIAN_POINT ( 'NONE',  ( 20.92219106202033529, -23.01025686871653875, -2.750000000000000000 ) ) ;
#8635=EDGE_CURVE ( 'NONE', #4853, #24341, #7209, .T. ) ;
#8638=CARTESIAN_POINT ( 'NONE',  ( -7.734255490826573265, 30.12293631110053838, -6.500000000000000000 ) ) ;
#8639=ORIENTED_EDGE ( 'NONE', *, *, #25465, .F. ) ;
#8641=ORIENTED_EDGE ( 'NONE', *, *, #2762, .T. ) ;
#8643=ORIENTED_EDGE ( 'NONE', *, *, #25329, .T. ) ;
#8645=EDGE_CURVE ( 'NONE', #7861, #19004, #24334, .T. ) ;
#8646=VERTEX_POINT ( 'NONE', #14402 ) ;
#8647=LINE ( 'NONE', #6677, #12775 ) ;
#8654=CARTESIAN_POINT ( 'NONE',  ( -13.69242354489161251, -27.92360179968368428, 1.000000000000000000 ) ) ;
#8656=LINE ( 'NONE', #2265, #25128 ) ;
#8657=LINE ( 'NONE', #16780, #14273 ) ;
#8661=DIRECTION ( 'NONE',  ( 0.000000000000000000, 0.000000000000000000, 1.000000000000000000 ) ) ;
#8662=EDGE_LOOP ( 'NONE', ( #23270, #10741, #3293, #23504 ) ) ;
#8663=ORIENTED_EDGE ( 'NONE', *, *, #9649, .F. ) ;
#8666=ORIENTED_EDGE ( 'NONE', *, *, #25118, .F. ) ;
#8668=VERTEX_POINT ( 'NONE', #14789 ) ;
#8670=EDGE_CURVE ( 'NONE', #13117, #822, #8760, .T. ) ;
#8671=ORIENTED_EDGE ( 'NONE', *, *, #10506, .T. ) ;
#8673=ORIENTED_EDGE ( 'NONE', *, *, #3234, .T. ) ;
#8684=CARTESIAN_POINT ( 'NONE',  ( -14.98253926456298579, 27.25313774936435962, -6.500000000000000000 ) ) ;
#8687=AXIS2_PLACEMENT_3D ( 'NONE', #12327, #16398, #22391 ) ;
#8689=ORIENTED_EDGE ( 'NONE', *, *, #1870, .F. ) ;
#8693=ORIENTED_EDGE ( 'NONE', *, *, #18211, .T. ) ;
#8694=VERTEX_POINT ( 'NONE', #4841 ) ;
#8695=DIRECTION ( 'NONE',  ( -0.000000000000000000, -0.000000000000000000, 1.000000000000000000 ) ) ;
#8702=CYLINDRICAL_SURFACE ( 'NONE', #25159, 31.10000000000000142 ) ;
#8707=VECTOR ( 'NONE', #3096, 1000.000000000000000 ) ;
#8709=DIRECTION ( 'NONE',  ( 0.000000000000000000, -0.000000000000000000, 1.000000000000000000 ) ) ;
#8710=AXIS2_PLACEMENT_3D ( 'NONE', #1595, #5648, #21348 ) ;
#8716=CARTESIAN_POINT ( 'NONE',  ( -24.66042852506104310, -18.28012134629567598, -6.500000000000000000 ) ) ;
#8719=DIRECTION ( 'NONE',  ( 1.000000000000000000, 0.000000000000000000, 0.000000000000000000 ) ) ;
#8720=ORIENTED_EDGE ( 'NONE', *, *, #1575, .T. ) ;
#8723=ORIENTED_EDGE ( 'NONE', *, *, #18735, .F. ) ;
#8724=CARTESIAN_POINT ( 'NONE',  ( -11.44867358849371541, -28.91604871112453168, 1.000000000000000000 ) ) ;
#8727=DIRECTION ( 'NONE',  ( 1.000000000000000000, 0.000000000000000000, 0.000000000000000000 ) ) ;
#8729=CARTESIAN_POINT ( 'NONE',  ( 26.52310962334739486, -16.23990935651726275, -2.750000000000000000 ) ) ;
#8732=EDGE_CURVE ( 'NONE', #22681, #10320, #7632, .T. ) ;
#8735=CIRCLE ( 'NONE', #5331, 31.10000000000000142 ) ;
#8740=EDGE_CURVE ( 'NONE', #24433, #10494, #9022, .T. ) ;
#8741=CARTESIAN_POINT ( 'NONE',  ( 0.000000000000000000, 0.000000000000000000, -6.500000000000000000 ) ) ;
#8743=DIRECTION ( 'NONE',  ( 0.000000000000000000, -0.000000000000000000, 1.000000000000000000 ) ) ;
#8746=EDGE_CURVE ( 'NONE', #18387, #19344, #24852, .T. ) ;
#8747=CARTESIAN_POINT ( 'NONE',  ( -31.03863125411927371, -1.952785157361310198, 1.000000000000000000 ) ) ;
#8748=VECTOR ( 'NONE', #15045, 1000.000000000000000 ) ;
#8749=CARTESIAN_POINT ( 'NONE',  ( 10.08469938919499320, 29.41953157733090762, -6.500000000000000000 ) ) ;
#8752=CARTESIAN_POINT ( 'NONE',  ( -13.69242354489114177, 27.92360179968391165, -6.500000000000000000 ) ) ;
#8755=DIRECTION ( 'NONE',  ( 0.000000000000000000, -0.000000000000000000, 1.000000000000000000 ) ) ;
#8758=CIRCLE ( 'NONE', #1669, 31.10000000000000142 ) ;
#8759=CARTESIAN_POINT ( 'NONE',  ( -3.397863563849436108, 30.85476721088031482, 1.000000000000000000 ) ) ;
#8760=LINE ( 'NONE', #18451, #6793 ) ;
#8761=ORIENTED_EDGE ( 'NONE', *, *, #2952, .F. ) ;
#8762=DIRECTION ( 'NONE',  ( 1.000000000000000000, 0.000000000000000000, 0.000000000000000000 ) ) ;
#8763=CARTESIAN_POINT ( 'NONE',  ( -28.72825533807142051, -11.91206721063020701, -2.750000000000000000 ) ) ;
#8766=VERTEX_POINT ( 'NONE', #14913 ) ;
#8772=DIRECTION ( 'NONE',  ( 0.000000000000000000, 0.000000000000000000, -1.000000000000000000 ) ) ;
#8774=CIRCLE ( 'NONE', #2515, 31.10000000000000142 ) ;
#8776=CARTESIAN_POINT ( 'NONE',  ( -29.07785765677917311, 9.610428525061202265, -6.500000000000000000 ) ) ;
#8779=EDGE_CURVE ( 'NONE', #18169, #5530, #3387, .T. ) ;
#8791=CARTESIAN_POINT ( 'NONE',  ( -14.98253926456356666, -27.25313774936403988, -6.500000000000000000 ) ) ;
#8793=CIRCLE ( 'NONE', #23409, 0.4999999999999998890 ) ;
#8794=CARTESIAN_POINT ( 'NONE',  ( 27.92360179968377309, 13.69242354489143665, 1.000000000000000000 ) ) ;
#8795=DIRECTION ( 'NONE',  ( 0.7289686274214101092, -0.6845471059286901694, 0.000000000000000000 ) ) ;
#8796=VERTEX_POINT ( 'NONE', #23263 ) ;
#8802=ORIENTED_EDGE ( 'NONE', *, *, #4870, .F. ) ;
#8804=ORIENTED_EDGE ( 'NONE', *, *, #17695, .F. ) ;
#8808=DIRECTION ( 'NONE',  ( 0.000000000000000000, 0.000000000000000000, 1.000000000000000000 ) ) ;
#8810=DIRECTION ( 'NONE',  ( -0.9048270524660170233, 0.4257792915650782661, 0.000000000000000000 ) ) ;
#8811=AXIS2_PLACEMENT_3D ( 'NONE', #20488, #2584, #18547 ) ;
#8812=CIRCLE ( 'NONE', #16346, 31.10000000000000142 ) ;
#8818=CIRCLE ( 'NONE', #24249, 31.10000000000000142 ) ;
#8819=EDGE_CURVE ( 'NONE', #24829, #21754, #8907, .T. ) ;
#8822=CARTESIAN_POINT ( 'NONE',  ( 2.451530025008918923, -31.00322564728515928, -6.500000000000000000 ) ) ;
#8824=ORIENTED_EDGE ( 'NONE', *, *, #10435, .T. ) ;
#8831=CYLINDRICAL_SURFACE ( 'NONE', #15856, 0.5000000000000004441 ) ;
#8833=DIRECTION ( 'NONE',  ( 0.8443279255020205154, 0.5358267949789882190, 0.000000000000000000 ) ) ;
#8834=DIRECTION ( 'NONE',  ( -1.000000000000000000, 0.000000000000000000, 0.000000000000000000 ) ) ;
#8835=VERTEX_POINT ( 'NONE', #20929 ) ;
#8836=EDGE_LOOP ( 'NONE', ( #3812, #10006, #16946, #5070 ) ) ;
#8837=LINE ( 'NONE', #20330, #10372 ) ;
#8838=AXIS2_PLACEMENT_3D ( 'NONE', #2166, #21905, #16034 ) ;
#8839=CYLINDRICAL_SURFACE ( 'NONE', #9225, 0.5000000000000000000 ) ;
#8840=ORIENTED_EDGE ( 'NONE', *, *, #23445, .F. ) ;
#8851=DIRECTION ( 'NONE',  ( 1.000000000000000000, 0.000000000000000000, 0.000000000000000000 ) ) ;
#8853=EDGE_CURVE ( 'NONE', #7580, #25532, #11493, .T. ) ;
#8855=CIRCLE ( 'NONE', #3017, 31.10000000000000142 ) ;
#8856=LINE ( 'NONE', #4402, #5902 ) ;
#8863=CARTESIAN_POINT ( 'NONE',  ( -3.897863563850083146, -30.85476721088024021, -6.500000000000000000 ) ) ;
#8865=EDGE_CURVE ( 'NONE', #17200, #10488, #8068, .T. ) ;
#8866=CYLINDRICAL_SURFACE ( 'NONE', #23340, 31.10000000000000142 ) ;
#8867=AXIS2_PLACEMENT_3D ( 'NONE', #23406, #11376, #24981 ) ;
#8870=EDGE_LOOP ( 'NONE', ( #10083, #3353, #21650, #21089 ) ) ;
#8874=CARTESIAN_POINT ( 'NONE',  ( 30.24338421796780807, 7.248980000274215740, 1.000000000000000000 ) ) ;
#8877=LINE ( 'NONE', #16860, #24174 ) ;
#8878=VERTEX_POINT ( 'NONE', #11878 ) ;
#8880=ORIENTED_EDGE ( 'NONE', *, *, #4692, .T. ) ;
#8881=ORIENTED_EDGE ( 'NONE', *, *, #21260, .F. ) ;
#8882=CYLINDRICAL_SURFACE ( 'NONE', #16417, 0.5000000000000004441 ) ;
#8885=DIRECTION ( 'NONE',  ( 1.000000000000000000, 0.000000000000000000, 0.000000000000000000 ) ) ;
#8886=AXIS2_PLACEMENT_3D ( 'NONE', #5740, #25633, #14250 ) ;
#8891=AXIS2_PLACEMENT_3D ( 'NONE', #15838, #14135, #5643 ) ;
#8893=CARTESIAN_POINT ( 'NONE',  ( -23.64116323484252291, -20.20656826142258211, -6.500000000000000000 ) ) ;
#8894=UNCERTAINTY_MEASURE_WITH_UNIT (LENGTH_MEASURE( 1.000000000000000082E-05 ), #1543, 'distance_accuracy_value', 'NONE');
#8897=DIRECTION ( 'NONE',  ( -0.7705132427757935831, -0.6374239897486843054, 0.000000000000000000 ) ) ;
#8898=CARTESIAN_POINT ( 'NONE',  ( -29.99470236596038220, -8.217531866530892515, -6.500000000000000000 ) ) ;
#8900=EDGE_CURVE ( 'NONE', #13187, #4613, #17258, .T. ) ;
#8904=CYLINDRICAL_SURFACE ( 'NONE', #20385, 0.5000000000000004441 ) ;
#8905=AXIS2_PLACEMENT_3D ( 'NONE', #7589, #11380, #7452 ) ;
#8906=CARTESIAN_POINT ( 'NONE',  ( 0.000000000000000000, 0.000000000000000000, 1.000000000000000000 ) ) ;
#8907=LINE ( 'NONE', #25105, #1387 ) ;
#8908=ORIENTED_EDGE ( 'NONE', *, *, #8732, .T. ) ;
#8910=CARTESIAN_POINT ( 'NONE',  ( -11.91206721063072216, -28.72825533807120735, -2.750000000000000000 ) ) ;
#8913=CIRCLE ( 'NONE', #21017, 0.5000000000000007772 ) ;
#8915=ORIENTED_EDGE ( 'NONE', *, *, #12866, .F. ) ;
#8917=EDGE_LOOP ( 'NONE', ( #23023, #3577, #703, #12627 ) ) ;
#8918=CARTESIAN_POINT ( 'NONE',  ( -24.27856662945513477, -19.43607991388973488, 1.000000000000000000 ) ) ;
#8919=ORIENTED_EDGE ( 'NONE', *, *, #17773, .F. ) ;
#8928=DIRECTION ( 'NONE',  ( 1.000000000000000000, 0.000000000000000000, 0.000000000000000000 ) ) ;
#8930=CARTESIAN_POINT ( 'NONE',  ( 3.897863563849651936, -30.85476721088028640, -6.500000000000000000 ) ) ;
#8937=EDGE_CURVE ( 'NONE', #14948, #15879, #18102, .T. ) ;
#8939=CARTESIAN_POINT ( 'NONE',  ( -1.952785157361201618, 31.03863125411927371, -6.500000000000000000 ) ) ;
#8940=ORIENTED_EDGE ( 'NONE', *, *, #24313, .F. ) ;
#8941=ORIENTED_EDGE ( 'NONE', *, *, #5630, .F. ) ;
#8944=DIRECTION ( 'NONE',  ( 0.000000000000000000, 0.000000000000000000, 1.000000000000000000 ) ) ;
#8949=EDGE_CURVE ( 'NONE', #13787, #4937, #19331, .T. ) ;
#8950=VECTOR ( 'NONE', #7388, 1000.000000000000000 ) ;
#8956=CARTESIAN_POINT ( 'NONE',  ( 21.65113613650334301, 22.32573188046921331, 1.000000000000000000 ) ) ;
#8961=DIRECTION ( 'NONE',  ( 1.000000000000000000, 0.000000000000000000, 0.000000000000000000 ) ) ;
#8965=LINE ( 'NONE', #25297, #8323 ) ;
#8971=ORIENTED_EDGE ( 'NONE', *, *, #12288, .F. ) ;
#8972=DIRECTION ( 'NONE',  ( 0.6374239897486995154, 0.7705132427757811486, 0.000000000000000000 ) ) ;
#8978=CARTESIAN_POINT ( 'NONE',  ( -11.91206721063010754, 28.72825533807145959, -2.750000000000000000 ) ) ;
#8984=DIRECTION ( 'NONE',  ( 0.000000000000000000, 0.000000000000000000, 1.000000000000000000 ) ) ;
#8986=CARTESIAN_POINT ( 'NONE',  ( -7.234255490826573265, 30.12293631110053838, -6.500000000000000000 ) ) ;
#8989=CARTESIAN_POINT ( 'NONE',  ( 0.000000000000000000, 0.000000000000000000, 1.000000000000000000 ) ) ;
#8994=CARTESIAN_POINT ( 'NONE',  ( 3.897863563849872204, 30.85476721088026508, -6.500000000000000000 ) ) ;
#8997=FACE_OUTER_BOUND ( 'NONE', #14691, .T. ) ;
#8999=CARTESIAN_POINT ( 'NONE',  ( -25.98730014090454432, -17.08421000182750760, 1.000000000000000000 ) ) ;
#9003=VERTEX_POINT ( 'NONE', #21948 ) ;
#9004=VERTEX_POINT ( 'NONE', #4027 ) ;
#9008=EDGE_CURVE ( 'NONE', #17868, #2787, #11695, .T. ) ;
#9012=CYLINDRICAL_SURFACE ( 'NONE', #1289, 31.10000000000000142 ) ;
#9016=DIRECTION ( 'NONE',  ( 1.000000000000000000, 0.000000000000000000, 0.000000000000000000 ) ) ;
#9017=CARTESIAN_POINT ( 'NONE',  ( -9.133673601486680838, -29.72853858738275434, -6.500000000000000000 ) ) ;
#9019=DIRECTION ( 'NONE',  ( 0.000000000000000000, 0.000000000000000000, 1.000000000000000000 ) ) ;
#9020=CARTESIAN_POINT ( 'NONE',  ( -30.12293631110050995, -7.734255490826679846, -6.500000000000000000 ) ) ;
#9021=CARTESIAN_POINT ( 'NONE',  ( -17.87326343783962201, -25.45105997952905597, -2.750000000000000000 ) ) ;
#9022=LINE ( 'NONE', #1304, #21427 ) ;
#9025=DIRECTION ( 'NONE',  ( 1.000000000000000000, 0.000000000000000000, 0.000000000000000000 ) ) ;
#9026=EDGE_LOOP ( 'NONE', ( #21156, #17034, #6961, #16298 ) ) ;
#9027=ORIENTED_EDGE ( 'NONE', *, *, #13139, .F. ) ;
#9028=ORIENTED_EDGE ( 'NONE', *, *, #208, .T. ) ;
#9032=CARTESIAN_POINT ( 'NONE',  ( 22.67092431280578779, -21.28941499438234786, -6.500000000000000000 ) ) ;
#9034=ORIENTED_EDGE ( 'NONE', *, *, #2689, .F. ) ;
#9041=EDGE_CURVE ( 'NONE', #9149, #20576, #4682, .T. ) ;
#9045=FACE_OUTER_BOUND ( 'NONE', #20329, .T. ) ;
#9046=CARTESIAN_POINT ( 'NONE',  ( 24.86329371854774806, 18.68225429291723216, 1.000000000000000000 ) ) ;
#9048=CARTESIAN_POINT ( 'NONE',  ( 31.00322564728513086, -2.451530025009243108, -2.750000000000000000 ) ) ;
#9050=CARTESIAN_POINT ( 'NONE',  ( 0.000000000000000000, 0.000000000000000000, 1.000000000000000000 ) ) ;
#9051=DIRECTION ( 'NONE',  ( 0.000000000000000000, 0.000000000000000000, -1.000000000000000000 ) ) ;
#9053=VERTEX_POINT ( 'NONE', #6384 ) ;
#9056=ORIENTED_EDGE ( 'NONE', *, *, #15274, .T. ) ;
#9060=EDGE_CURVE ( 'NONE', #14404, #9218, #4296, .T. ) ;
#9062=CARTESIAN_POINT ( 'NONE',  ( -13.24173596767339767, 28.14012133169338270, -6.500000000000000000 ) ) ;
#9065=ADVANCED_FACE ( 'NONE', ( #8217 ), #18283, .F. ) ;
#9066=DIRECTION ( 'NONE',  ( 0.000000000000000000, -0.000000000000000000, 1.000000000000000000 ) ) ;
#9074=FACE_OUTER_BOUND ( 'NONE', #12132, .T. ) ;
#9082=VERTEX_POINT ( 'NONE', #2451 ) ;
#9083=ORIENTED_EDGE ( 'NONE', *, *, #4278, .F. ) ;
#9084=DIRECTION ( 'NONE',  ( 1.000000000000000000, 0.000000000000000000, 0.000000000000000000 ) ) ;
#9089=DIRECTION ( 'NONE',  ( 1.000000000000000000, 0.000000000000000000, 0.000000000000000000 ) ) ;
#9093=CARTESIAN_POINT ( 'NONE',  ( -5.327558883616270613, -30.54913349766217934, -6.500000000000000000 ) ) ;
#9097=AXIS2_PLACEMENT_3D ( 'NONE', #13881, #9437, #15834 ) ;
#9111=DIRECTION ( 'NONE',  ( 1.000000000000000000, 0.000000000000000000, 0.000000000000000000 ) ) ;
#9121=CIRCLE ( 'NONE', #22076, 0.5000000000000005551 ) ;
#9123=CIRCLE ( 'NONE', #8710, 0.5000000000000001110 ) ;
#9134=DIRECTION ( 'NONE',  ( 0.000000000000000000, 0.000000000000000000, 1.000000000000000000 ) ) ;
#9135=CARTESIAN_POINT ( 'NONE',  ( -30.12293631110035363, 7.734255490827311341, -6.500000000000000000 ) ) ;
#9137=CARTESIAN_POINT ( 'NONE',  ( -7.734255490827218971, -30.12293631110037140, -6.500000000000000000 ) ) ;
#9138=CARTESIAN_POINT ( 'NONE',  ( -30.04913349766215802, 5.827558883616378083, -6.500000000000000000 ) ) ;
#9141=VECTOR ( 'NONE', #16372, 1000.000000000000000 ) ;
#9142=CARTESIAN_POINT ( 'NONE',  ( -13.24173596767398742, -28.14012133169310559, 1.000000000000000000 ) ) ;
#9144=CIRCLE ( 'NONE', #382, 31.10000000000000142 ) ;
#9145=ORIENTED_EDGE ( 'NONE', *, *, #14033, .F. ) ;
#9146=EDGE_CURVE ( 'NONE', #10041, #16921, #2949, .T. ) ;
#9148=DIRECTION ( 'NONE',  ( 0.000000000000000000, -0.000000000000000000, 1.000000000000000000 ) ) ;
#9149=VERTEX_POINT ( 'NONE', #2837 ) ;
#9152=ORIENTED_EDGE ( 'NONE', *, *, #25260, .T. ) ;
#9153=AXIS2_PLACEMENT_3D ( 'NONE', #15682, #22208, #5862 ) ;
#9157=CARTESIAN_POINT ( 'NONE',  ( 0.000000000000000000, 0.000000000000000000, 1.000000000000000000 ) ) ;
#9165=AXIS2_PLACEMENT_3D ( 'NONE', #21491, #9199, #7625 ) ;
#9166=DIRECTION ( 'NONE',  ( 1.000000000000000000, 0.000000000000000000, 0.000000000000000000 ) ) ;
#9170=CARTESIAN_POINT ( 'NONE',  ( -23.96296185032722548, -19.82388608118403539, -6.500000000000000000 ) ) ;
#9178=ORIENTED_EDGE ( 'NONE', *, *, #8645, .F. ) ;
#9189=VERTEX_POINT ( 'NONE', #21269 ) ;
#9192=AXIS2_PLACEMENT_3D ( 'NONE', #12206, #187, #4478 ) ;
#9196=DIRECTION ( 'NONE',  ( 0.000000000000000000, 0.000000000000000000, 1.000000000000000000 ) ) ;
#9197=CIRCLE ( 'NONE', #14219, 0.5000000000000005551 ) ;
#9199=DIRECTION ( 'NONE',  ( -0.000000000000000000, -0.000000000000000000, 1.000000000000000000 ) ) ;
#9201=AXIS2_PLACEMENT_3D ( 'NONE', #7600, #7341, #19366 ) ;
#9205=AXIS2_PLACEMENT_3D ( 'NONE', #21578, #25257, #3409 ) ;
#9207=DIRECTION ( 'NONE',  ( 0.9980267284282724471, 0.06279051952930156388, 0.000000000000000000 ) ) ;
#9208=EDGE_CURVE ( 'NONE', #25179, #1141, #13795, .T. ) ;
#9209=ORIENTED_EDGE ( 'NONE', *, *, #6525, .T. ) ;
#9210=ORIENTED_EDGE ( 'NONE', *, *, #7623, .F. ) ;
#9213=EDGE_CURVE ( 'NONE', #21597, #6260, #21026, .T. ) ;
#9214=CARTESIAN_POINT ( 'NONE',  ( -29.09636799667067564, 10.98232076577254368, 1.000000000000000000 ) ) ;
#9215=VECTOR ( 'NONE', #21800, 1000.000000000000000 ) ;
#9218=VERTEX_POINT ( 'NONE', #4811 ) ;
#9220=CARTESIAN_POINT ( 'NONE',  ( 0.000000000000000000, 0.000000000000000000, 1.000000000000000000 ) ) ;
#9222=CIRCLE ( 'NONE', #15904, 31.10000000000000142 ) ;
#9223=CARTESIAN_POINT ( 'NONE',  ( 0.000000000000000000, 0.000000000000000000, -6.500000000000000000 ) ) ;
#9224=ORIENTED_EDGE ( 'NONE', *, *, #4278, .T. ) ;
#9225=AXIS2_PLACEMENT_3D ( 'NONE', #6873, #22831, #7265 ) ;
#9229=CIRCLE ( 'NONE', #12567, 0.5000000000000007772 ) ;
#9236=DIRECTION ( 'NONE',  ( -0.9510565162951518658, 0.3090169943749528914, 0.000000000000000000 ) ) ;
#9237=AXIS2_PLACEMENT_3D ( 'NONE', #22203, #4290, #8336 ) ;
#9238=AXIS2_PLACEMENT_3D ( 'NONE', #20221, #13835, #14225 ) ;
#9239=FACE_OUTER_BOUND ( 'NONE', #7963, .T. ) ;
#9255=FACE_OUTER_BOUND ( 'NONE', #24299, .T. ) ;
#9259=VERTEX_POINT ( 'NONE', #2975 ) ;
#9261=EDGE_LOOP ( 'NONE', ( #21068, #5901, #20118, #13572 ) ) ;
#9264=AXIS2_PLACEMENT_3D ( 'NONE', #10293, #13981, #21950 ) ;
#9270=( LENGTH_UNIT ( ) NAMED_UNIT ( * ) SI_UNIT ( .MILLI., .METRE. ) );
#9273=AXIS2_PLACEMENT_3D ( 'NONE', #10303, #12009, #22084 ) ;
#9274=DIRECTION ( 'NONE',  ( 1.000000000000000000, 0.000000000000000000, 0.000000000000000000 ) ) ;
#9276=DIRECTION ( 'NONE',  ( -0.3090169943749528914, -0.9510565162951518658, 0.000000000000000000 ) ) ;
#9277=LINE ( 'NONE', #23141, #7876 ) ;
#9283=CIRCLE ( 'NONE', #10512, 31.10000000000000142 ) ;
#9284=LINE ( 'NONE', #14911, #4964 ) ;
#9285=DIRECTION ( 'NONE',  ( 1.000000000000000000, 0.000000000000000000, 0.000000000000000000 ) ) ;
#9290=DIRECTION ( 'NONE',  ( 1.000000000000000000, 0.000000000000000000, 0.000000000000000000 ) ) ;
#9291=ORIENTED_EDGE ( 'NONE', *, *, #21260, .T. ) ;
#9292=EDGE_CURVE ( 'NONE', #10594, #2244, #19048, .T. ) ;
#9294=EDGE_LOOP ( 'NONE', ( #12026, #11071, #898, #9634 ) ) ;
#9296=ORIENTED_EDGE ( 'NONE', *, *, #3390, .F. ) ;
#9297=CARTESIAN_POINT ( 'NONE',  ( 27.25313774936419620, 14.98253926456328244, -6.500000000000000000 ) ) ;
#9300=VECTOR ( 'NONE', #3532, 1000.000000000000000 ) ;
#9310=CARTESIAN_POINT ( 'NONE',  ( -13.24173596767339767, 28.14012133169338270, -6.500000000000000000 ) ) ;
#9315=AXIS2_PLACEMENT_3D ( 'NONE', #1840, #11888, #9677 ) ;
#9318=ORIENTED_EDGE ( 'NONE', *, *, #25140, .F. ) ;
#9319=EDGE_CURVE ( 'NONE', #22273, #19788, #20907, .T. ) ;
#9324=DIRECTION ( 'NONE',  ( 0.000000000000000000, -0.000000000000000000, 1.000000000000000000 ) ) ;
#9325=ORIENTED_EDGE ( 'NONE', *, *, #22246, .T. ) ;
#9336=DIRECTION ( 'NONE',  ( 0.000000000000000000, 0.000000000000000000, -1.000000000000000000 ) ) ;
#9345=ORIENTED_EDGE ( 'NONE', *, *, #1634, .T. ) ;
#9346=ORIENTED_EDGE ( 'NONE', *, *, #14439, .F. ) ;
#9349=VECTOR ( 'NONE', #9393, 1000.000000000000000 ) ;
#9355=ORIENTED_EDGE ( 'NONE', *, *, #14577, .T. ) ;
#9362=CARTESIAN_POINT ( 'NONE',  ( 30.12293631110045311, 7.734255490826897450, -6.500000000000000000 ) ) ;
#9367=EDGE_CURVE ( 'NONE', #24860, #5409, #5445, .T. ) ;
#9368=CARTESIAN_POINT ( 'NONE',  ( -28.41604871112448549, 11.44867358849382910, -6.500000000000000000 ) ) ;
#9376=CARTESIAN_POINT ( 'NONE',  ( -10.98232076577192196, 29.09636799667091012, 1.000000000000000000 ) ) ;
#9378=EDGE_CURVE ( 'NONE', #20930, #11374, #11459, .T. ) ;
#9385=DIRECTION ( 'NONE',  ( 0.000000000000000000, 0.000000000000000000, 1.000000000000000000 ) ) ;
#9386=VERTEX_POINT ( 'NONE', #13811 ) ;
#9389=VERTEX_POINT ( 'NONE', #19433 ) ;
#9390=VERTEX_POINT ( 'NONE', #3608 ) ;
#9393=DIRECTION ( 'NONE',  ( -0.000000000000000000, 0.000000000000000000, -1.000000000000000000 ) ) ;
#9394=EDGE_CURVE ( 'NONE', #11934, #24237, #17149, .T. ) ;
#9396=CARTESIAN_POINT ( 'NONE',  ( 0.000000000000000000, 0.000000000000000000, 1.000000000000000000 ) ) ;
#9399=DIRECTION ( 'NONE',  ( 0.000000000000000000, 0.000000000000000000, 1.000000000000000000 ) ) ;
#9400=CARTESIAN_POINT ( 'NONE',  ( -29.72853858738272592, 9.133673601486785643, -2.750000000000000000 ) ) ;
#9403=VERTEX_POINT ( 'NONE', #1791 ) ;
#9405=DIRECTION ( 'NONE',  ( -0.000000000000000000, -0.000000000000000000, 1.000000000000000000 ) ) ;
#9407=DIRECTION ( 'NONE',  ( -0.000000000000000000, -0.000000000000000000, 1.000000000000000000 ) ) ;
#9409=DIRECTION ( 'NONE',  ( 1.000000000000000000, 0.000000000000000000, 0.000000000000000000 ) ) ;
#9414=DIRECTION ( 'NONE',  ( -0.8763066800438656934, -0.4817536741017116597, 0.000000000000000000 ) ) ;
#9415=VERTEX_POINT ( 'NONE', #23313 ) ;
#9417=EDGE_LOOP ( 'NONE', ( #10179, #10957, #13718, #15326 ) ) ;
#9418=ORIENTED_EDGE ( 'NONE', *, *, #105, .T. ) ;
#9419=ORIENTED_EDGE ( 'NONE', *, *, #5525, .T. ) ;
#9420=CARTESIAN_POINT ( 'NONE',  ( 0.000000000000000000, 0.000000000000000000, -6.500000000000000000 ) ) ;
#9423=CIRCLE ( 'NONE', #18208, 0.4999999999999997224 ) ;
#9431=ADVANCED_FACE ( 'NONE', ( #15344 ), #5023, .T. ) ;
#9433=DIRECTION ( 'NONE',  ( 1.000000000000000000, 0.000000000000000000, 0.000000000000000000 ) ) ;
#9437=DIRECTION ( 'NONE',  ( 0.000000000000000000, 0.000000000000000000, 1.000000000000000000 ) ) ;
#9440=EDGE_LOOP ( 'NONE', ( #25803, #19374, #22919, #21486 ) ) ;
#9443=EDGE_CURVE ( 'NONE', #51, #23094, #8793, .T. ) ;
#9444=ORIENTED_EDGE ( 'NONE', *, *, #20059, .F. ) ;
#9458=EDGE_CURVE ( 'NONE', #14350, #12673, #4888, .T. ) ;
#9463=ORIENTED_EDGE ( 'NONE', *, *, #15852, .T. ) ;
#9464=VERTEX_POINT ( 'NONE', #22813 ) ;
#9473=ORIENTED_EDGE ( 'NONE', *, *, #16940, .F. ) ;
#9475=ORIENTED_EDGE ( 'NONE', *, *, #15387, .T. ) ;
#9479=CARTESIAN_POINT ( 'NONE',  ( 0.000000000000000000, 0.000000000000000000, -6.500000000000000000 ) ) ;
#9482=CARTESIAN_POINT ( 'NONE',  ( -14.98253926456298579, 27.25313774936435962, 1.000000000000000000 ) ) ;
#9483=CARTESIAN_POINT ( 'NONE',  ( 0.000000000000000000, 0.000000000000000000, -6.500000000000000000 ) ) ;
#9490=FACE_OUTER_BOUND ( 'NONE', #21981, .T. ) ;
#9496=ADVANCED_FACE ( 'NONE', ( #15225 ), #13004, .F. ) ;
#9497=DIRECTION ( 'NONE',  ( 1.000000000000000000, 0.000000000000000000, 0.000000000000000000 ) ) ;
#9498=ORIENTED_EDGE ( 'NONE', *, *, #16501, .T. ) ;
#9500=EDGE_CURVE ( 'NONE', #485, #1055, #21223, .T. ) ;
#9504=ORIENTED_EDGE ( 'NONE', *, *, #13555, .F. ) ;
#9505=VERTEX_POINT ( 'NONE', #7246 ) ;
#9509=CIRCLE ( 'NONE', #25382, 0.5000000000000013323 ) ;
#9511=DIRECTION ( 'NONE',  ( 1.000000000000000000, 0.000000000000000000, 0.000000000000000000 ) ) ;
#9515=DIRECTION ( 'NONE',  ( 0.000000000000000000, 0.000000000000000000, 1.000000000000000000 ) ) ;
#9516=CARTESIAN_POINT ( 'NONE',  ( 27.25313774936409317, -14.98253926456347074, 1.000000000000000000 ) ) ;
#9517=DIRECTION ( 'NONE',  ( -0.000000000000000000, -0.000000000000000000, 1.000000000000000000 ) ) ;
#9519=ORIENTED_EDGE ( 'NONE', *, *, #8233, .F. ) ;
#9524=DIRECTION ( 'NONE',  ( 0.000000000000000000, -0.000000000000000000, 1.000000000000000000 ) ) ;
#9525=EDGE_CURVE ( 'NONE', #18011, #7791, #5276, .T. ) ;
#9530=CARTESIAN_POINT ( 'NONE',  ( -10.98232076577242466, -29.09636799667071116, -6.500000000000000000 ) ) ;
#9532=ADVANCED_FACE ( 'NONE', ( #15100 ), #11031, .T. ) ;
#9534=AXIS2_PLACEMENT_3D ( 'NONE', #18448, #24456, #6534 ) ;
#9535=ORIENTED_EDGE ( 'NONE', *, *, #18400, .F. ) ;
#9538=DIRECTION ( 'NONE',  ( 0.000000000000000000, 0.000000000000000000, 1.000000000000000000 ) ) ;
#9539=CARTESIAN_POINT ( 'NONE',  ( 28.14012133169314822, -13.24173596767388794, 1.000000000000000000 ) ) ;
#9542=CARTESIAN_POINT ( 'NONE',  ( -22.67092431280563503, 21.28941499438250062, 1.000000000000000000 ) ) ;
#9550=CARTESIAN_POINT ( 'NONE',  ( 0.000000000000000000, 0.000000000000000000, -6.500000000000000000 ) ) ;
#9556=FACE_BOUND ( 'NONE', #14922, .T. ) ;
#9558=CIRCLE ( 'NONE', #14158, 31.10000000000000142 ) ;
#9559=FACE_OUTER_BOUND ( 'NONE', #24729, .T. ) ;
#9566=EDGE_LOOP ( 'NONE', ( #8343, #11080, #5736, #16083 ) ) ;
#9569=DIRECTION ( 'NONE',  ( 0.5358267949790093132, 0.8443279255020070817, 0.000000000000000000 ) ) ;
#9574=CARTESIAN_POINT ( 'NONE',  ( -30.53863125411927371, -1.952785157361310198, -6.500000000000000000 ) ) ;
#9577=VECTOR ( 'NONE', #5106, 1000.000000000000000 ) ;
#9578=CARTESIAN_POINT ( 'NONE',  ( -30.12293631110050995, -7.734255490826679846, -6.500000000000000000 ) ) ;
#9579=DIRECTION ( 'NONE',  ( -0.5877852522924652545, 0.8090169943749532244, 0.000000000000000000 ) ) ;
#9581=CARTESIAN_POINT ( 'NONE',  ( 0.000000000000000000, 0.000000000000000000, -6.500000000000000000 ) ) ;
#9582=AXIS2_PLACEMENT_3D ( 'NONE', #8250, #14014, #15984 ) ;
#9584=VECTOR ( 'NONE', #23221, 1000.000000000000000 ) ;
#9587=CIRCLE ( 'NONE', #25456, 0.5000000000000017764 ) ;
#9591=CIRCLE ( 'NONE', #12944, 0.4999999999999999445 ) ;
#9593=AXIS2_PLACEMENT_3D ( 'NONE', #7917, #23618, #1650 ) ;
#9597=ORIENTED_EDGE ( 'NONE', *, *, #13421, .F. ) ;
#9600=FACE_OUTER_BOUND ( 'NONE', #826, .T. ) ;
#9601=AXIS2_PLACEMENT_3D ( 'NONE', #13850, #4031, #14106 ) ;
#9602=ORIENTED_EDGE ( 'NONE', *, *, #15921, .F. ) ;
#9603=CARTESIAN_POINT ( 'NONE',  ( -25.98730014090425300, 17.08421000182794813, 1.000000000000000000 ) ) ;
#9607=AXIS2_PLACEMENT_3D ( 'NONE', #9170, #17160, #23169 ) ;
#9612=AXIS2_PLACEMENT_3D ( 'NONE', #24087, #297, #13907 ) ;
#9613=EDGE_CURVE ( 'NONE', #11934, #19625, #12147, .T. ) ;
#9615=DIRECTION ( 'NONE',  ( 0.8763066800438685799, 0.4817536741017063306, 0.000000000000000000 ) ) ;
#9622=CARTESIAN_POINT ( 'NONE',  ( 30.91344420362548107, 3.401318489840985837, -2.750000000000000000 ) ) ;
#9624=CIRCLE ( 'NONE', #24244, 0.5000000000000005551 ) ;
#9629=ORIENTED_EDGE ( 'NONE', *, *, #6132, .T. ) ;
#9634=ORIENTED_EDGE ( 'NONE', *, *, #20217, .T. ) ;
#9637=FACE_OUTER_BOUND ( 'NONE', #11912, .T. ) ;
#9640=ORIENTED_EDGE ( 'NONE', *, *, #4807, .T. ) ;
#9641=ORIENTED_EDGE ( 'NONE', *, *, #707, .T. ) ;
#9645=AXIS2_PLACEMENT_3D ( 'NONE', #24878, #7220, #24607 ) ;
#9646=AXIS2_PLACEMENT_3D ( 'NONE', #18823, #16603, #16487 ) ;
#9647=FACE_OUTER_BOUND ( 'NONE', #13261, .T. ) ;
#9649=EDGE_CURVE ( 'NONE', #16676, #18810, #25519, .T. ) ;
#9652=ADVANCED_FACE ( 'NONE', ( #11925 ), #23831, .T. ) ;
#9654=CARTESIAN_POINT ( 'NONE',  ( -30.54913349766228592, -5.827558883615738594, -6.500000000000000000 ) ) ;
#9656=DIRECTION ( 'NONE',  ( -0.9980267284282710039, 0.06279051952932233893, 0.000000000000000000 ) ) ;
#9658=CYLINDRICAL_SURFACE ( 'NONE', #9713, 0.5000000000000004441 ) ;
#9660=DIRECTION ( 'NONE',  ( -0.4257792915650642218, 0.9048270524660235736, 0.000000000000000000 ) ) ;
#9661=CARTESIAN_POINT ( 'NONE',  ( 11.91206721063051432, 28.72825533807128551, -2.750000000000000000 ) ) ;
#9664=AXIS2_PLACEMENT_3D ( 'NONE', #22685, #4770, #16541 ) ;
#9667=ORIENTED_EDGE ( 'NONE', *, *, #10121, .F. ) ;
#9668=CARTESIAN_POINT ( 'NONE',  ( -9.133673601486059113, 29.72853858738294619, -6.500000000000000000 ) ) ;
#9669=CARTESIAN_POINT ( 'NONE',  ( -1.952785157361201618, 31.03863125411927371, -6.500000000000000000 ) ) ;
#9671=EDGE_LOOP ( 'NONE', ( #16472, #10261, #6838, #25013 ) ) ;
#9672=CIRCLE ( 'NONE', #10905, 31.10000000000000142 ) ;
#9673=VERTEX_POINT ( 'NONE', #9963 ) ;
#9677=DIRECTION ( 'NONE',  ( 0.1873813145857189666, -0.9822872507286897203, 0.000000000000000000 ) ) ;
#9678=AXIS2_PLACEMENT_3D ( 'NONE', #21680, #7697, #5723 ) ;
#9679=DIRECTION ( 'NONE',  ( -0.000000000000000000, 0.000000000000000000, -1.000000000000000000 ) ) ;
#9682=AXIS2_PLACEMENT_3D ( 'NONE', #4003, #25842, #21922 ) ;
#9686=AXIS2_PLACEMENT_3D ( 'NONE', #25130, #3659, #1714 ) ;
#9692=CARTESIAN_POINT ( 'NONE',  ( 0.000000000000000000, 0.000000000000000000, 1.000000000000000000 ) ) ;
#9696=EDGE_CURVE ( 'NONE', #16624, #3323, #5877, .T. ) ;
#9697=AXIS2_PLACEMENT_3D ( 'NONE', #11988, #2325, #13974 ) ;
#9699=DIRECTION ( 'NONE',  ( 0.000000000000000000, 0.000000000000000000, 1.000000000000000000 ) ) ;
#9702=ORIENTED_EDGE ( 'NONE', *, *, #17934, .F. ) ;
#9705=AXIS2_PLACEMENT_3D ( 'NONE', #6296, #12037, #2374 ) ;
#9706=ORIENTED_EDGE ( 'NONE', *, *, #19420, .T. ) ;
#9708=ORIENTED_EDGE ( 'NONE', *, *, #25661, .F. ) ;
#9710=EDGE_LOOP ( 'NONE', ( #18082, #6992, #17551, #15727 ) ) ;
#9711=DIRECTION ( 'NONE',  ( -0.1253332335642912687, 0.9921147013144795412, 0.000000000000000000 ) ) ;
#9713=AXIS2_PLACEMENT_3D ( 'NONE', #15552, #17640, #21817 ) ;
#9714=ORIENTED_EDGE ( 'NONE', *, *, #10693, .F. ) ;
#9718=DIRECTION ( 'NONE',  ( 0.000000000000000000, 0.000000000000000000, 1.000000000000000000 ) ) ;
#9720=EDGE_CURVE ( 'NONE', #5290, #15106, #23001, .T. ) ;
#9725=DIRECTION ( 'NONE',  ( 1.000000000000000000, 0.000000000000000000, 0.000000000000000000 ) ) ;
#9726=VECTOR ( 'NONE', #2169, 1000.000000000000000 ) ;
#9729=VERTEX_POINT ( 'NONE', #16123 ) ;
#9733=ORIENTED_EDGE ( 'NONE', *, *, #7770, .F. ) ;
#9734=DIRECTION ( 'NONE',  ( 1.000000000000000000, 0.000000000000000000, 0.000000000000000000 ) ) ;
#9735=VECTOR ( 'NONE', #11661, 1000.000000000000000 ) ;
#9736=EDGE_LOOP ( 'NONE', ( #25175, #1836, #10565, #7543 ) ) ;
#9739=DIRECTION ( 'NONE',  ( -0.000000000000000000, 0.000000000000000000, 1.000000000000000000 ) ) ;
#9740=ORIENTED_EDGE ( 'NONE', *, *, #107, .T. ) ;
#9749=AXIS2_PLACEMENT_3D ( 'NONE', #4944, #904, #8885 ) ;
#9750=EDGE_CURVE ( 'NONE', #1796, #8646, #1725, .T. ) ;
#9751=CARTESIAN_POINT ( 'NONE',  ( 31.09598070739550479, -0.4999838450260851164, -6.500000000000000000 ) ) ;
#9758=LINE ( 'NONE', #5963, #3319 ) ;
#9764=ORIENTED_EDGE ( 'NONE', *, *, #19449, .F. ) ;
#9770=CARTESIAN_POINT ( 'NONE',  ( -31.10000000000000142, 3.257552089140643357E-13, -6.500000000000000000 ) ) ;
#9771=ORIENTED_EDGE ( 'NONE', *, *, #20313, .F. ) ;
#9773=DIRECTION ( 'NONE',  ( -0.000000000000000000, 0.000000000000000000, -1.000000000000000000 ) ) ;
#9776=CARTESIAN_POINT ( 'NONE',  ( -16.23990935651680445, 26.52310962334767908, -2.750000000000000000 ) ) ;
#9778=DIRECTION ( 'NONE',  ( 0.000000000000000000, 0.000000000000000000, 1.000000000000000000 ) ) ;
#9788=CARTESIAN_POINT ( 'NONE',  ( -27.25313774936397948, 14.98253926456367502, 1.000000000000000000 ) ) ;
#9790=CARTESIAN_POINT ( 'NONE',  ( -5.327558883615603591, 30.54913349766230724, 1.000000000000000000 ) ) ;
#9791=DIRECTION ( 'NONE',  ( 0.000000000000000000, 0.000000000000000000, 1.000000000000000000 ) ) ;
#9793=CARTESIAN_POINT ( 'NONE',  ( 2.451530025008918923, -31.00322564728515928, -2.750000000000000000 ) ) ;
#9794=CARTESIAN_POINT ( 'NONE',  ( -28.14012133169306296, 13.24173596767408867, -6.500000000000000000 ) ) ;
#9797=ADVANCED_FACE ( 'NONE', ( #18215 ), #14155, .T. ) ;
#9798=EDGE_LOOP ( 'NONE', ( #11963, #12002, #24756, #22827 ) ) ;
#9800=ORIENTED_EDGE ( 'NONE', *, *, #15969, .F. ) ;
#9801=EDGE_CURVE ( 'NONE', #19150, #23030, #12190, .T. ) ;
#9812=DIRECTION ( 'NONE',  ( 0.000000000000000000, 0.000000000000000000, 1.000000000000000000 ) ) ;
#9814=CARTESIAN_POINT ( 'NONE',  ( -23.01025686871661335, -20.92219106202025714, -2.750000000000000000 ) ) ;
#9815=CARTESIAN_POINT ( 'NONE',  ( -19.43607991389006528, -24.27856662945486832, -2.750000000000000000 ) ) ;
#9819=DIRECTION ( 'NONE',  ( 0.9510565162951586382, 0.3090169943749320192, 0.000000000000000000 ) ) ;
#9820=DIRECTION ( 'NONE',  ( 0.000000000000000000, 0.000000000000000000, 1.000000000000000000 ) ) ;
#9822=ORIENTED_EDGE ( 'NONE', *, *, #18741, .T. ) ;
#9823=DIRECTION ( 'NONE',  ( 0.000000000000000000, 0.000000000000000000, 1.000000000000000000 ) ) ;
#9825=ORIENTED_EDGE ( 'NONE', *, *, #23587, .F. ) ;
#9829=EDGE_CURVE ( 'NONE', #6029, #6210, #9222, .T. ) ;
#9831=DIRECTION ( 'NONE',  ( 0.000000000000000000, 0.000000000000000000, 1.000000000000000000 ) ) ;
#9832=EDGE_CURVE ( 'NONE', #23923, #15811, #7553, .T. ) ;
#9833=ORIENTED_EDGE ( 'NONE', *, *, #10998, .T. ) ;
#9840=DIRECTION ( 'NONE',  ( 1.000000000000000000, 0.000000000000000000, 0.000000000000000000 ) ) ;
#9841=CYLINDRICAL_SURFACE ( 'NONE', #15061, 0.5000000000000004441 ) ;
#9846=DIRECTION ( 'NONE',  ( 0.6845471059286972748, 0.7289686274214034478, 0.000000000000000000 ) ) ;
#9847=CIRCLE ( 'NONE', #24037, 31.10000000000000142 ) ;
#9848=ORIENTED_EDGE ( 'NONE', *, *, #23472, .T. ) ;
#9849=ORIENTED_EDGE ( 'NONE', *, *, #11499, .F. ) ;
#9852=LINE ( 'NONE', #17835, #16694 ) ;
#9853=EDGE_CURVE ( 'NONE', #17013, #18550, #20161, .T. ) ;
#9857=ORIENTED_EDGE ( 'NONE', *, *, #22807, .F. ) ;
#9861=ORIENTED_EDGE ( 'NONE', *, *, #998, .F. ) ;
#9865=CARTESIAN_POINT ( 'NONE',  ( 0.000000000000000000, 0.000000000000000000, -6.500000000000000000 ) ) ;
#9875=CARTESIAN_POINT ( 'NONE',  ( -22.17092431280563503, 21.28941499438250062, 1.000000000000000000 ) ) ;
#9876=DIRECTION ( 'NONE',  ( -0.6845471059286831750, 0.7289686274214168815, 0.000000000000000000 ) ) ;
#9878=ORIENTED_EDGE ( 'NONE', *, *, #4843, .F. ) ;
#9887=ORIENTED_EDGE ( 'NONE', *, *, #24881, .T. ) ;
#9889=CARTESIAN_POINT ( 'NONE',  ( -0.4999838450259764255, 31.09598070739550124, -6.500000000000000000 ) ) ;
#9891=EDGE_CURVE ( 'NONE', #24264, #14407, #296, .T. ) ;
#9895=CARTESIAN_POINT ( 'NONE',  ( 0.000000000000000000, 0.000000000000000000, -6.500000000000000000 ) ) ;
#9896=DIRECTION ( 'NONE',  ( 0.000000000000000000, 0.000000000000000000, 1.000000000000000000 ) ) ;
#9897=LINE ( 'NONE', #12255, #21361 ) ;
#9908=CARTESIAN_POINT ( 'NONE',  ( -30.45149776762723448, 6.317933499823641164, 1.000000000000000000 ) ) ;
#9912=CARTESIAN_POINT ( 'NONE',  ( -10.08469938919519926, -29.41953157733083302, -2.750000000000000000 ) ) ;
#9913=CARTESIAN_POINT ( 'NONE',  ( -30.12293631110035363, 7.734255490827311341, -6.500000000000000000 ) ) ;
#9914=ORIENTED_EDGE ( 'NONE', *, *, #17759, .F. ) ;
#9916=ORIENTED_EDGE ( 'NONE', *, *, #4755, .T. ) ;
#9918=CARTESIAN_POINT ( 'NONE',  ( -3.897863563849436552, 30.85476721088031482, 1.000000000000000000 ) ) ;
#9921=VECTOR ( 'NONE', #3185, 1000.000000000000000 ) ;
#9923=EDGE_CURVE ( 'NONE', #13585, #1315, #10336, .T. ) ;
#9927=ADVANCED_FACE ( 'NONE', ( #2646 ), #24357, .F. ) ;
#9935=ADVANCED_FACE ( 'NONE', ( #2859 ), #3000, .T. ) ;
#9936=DIRECTION ( 'NONE',  ( 0.000000000000000000, 0.000000000000000000, 1.000000000000000000 ) ) ;
#9939=DIRECTION ( 'NONE',  ( 0.000000000000000000, 0.000000000000000000, 1.000000000000000000 ) ) ;
#9940=CIRCLE ( 'NONE', #766, 0.5000000000000003331 ) ;
#9957=AXIS2_PLACEMENT_3D ( 'NONE', #22981, #10940, #24539 ) ;
#9959=AXIS2_PLACEMENT_3D ( 'NONE', #6237, #2321, #3898 ) ;
#9963=CARTESIAN_POINT ( 'NONE',  ( -29.07785765677936851, -9.610428525060582317, -6.500000000000000000 ) ) ;
#9964=VECTOR ( 'NONE', #11793, 1000.000000000000000 ) ;
#9968=EDGE_CURVE ( 'NONE', #16896, #3917, #4212, .T. ) ;
#9972=VERTEX_POINT ( 'NONE', #2737 ) ;
#9973=ORIENTED_EDGE ( 'NONE', *, *, #13013, .T. ) ;
#9975=VERTEX_POINT ( 'NONE', #12409 ) ;
#9978=AXIS2_PLACEMENT_3D ( 'NONE', #15932, #10029, #12122 ) ;
#9980=VERTEX_POINT ( 'NONE', #4953 ) ;
#9983=ORIENTED_EDGE ( 'NONE', *, *, #6110, .F. ) ;
#9986=CYLINDRICAL_SURFACE ( 'NONE', #1807, 31.10000000000000142 ) ;
#9988=DIRECTION ( 'NONE',  ( 1.000000000000000000, 0.000000000000000000, 0.000000000000000000 ) ) ;
#9990=CIRCLE ( 'NONE', #420, 0.5000000000000017764 ) ;
#9994=EDGE_CURVE ( 'NONE', #25291, #19323, #2131, .T. ) ;
#9995=CARTESIAN_POINT ( 'NONE',  ( 0.000000000000000000, 0.000000000000000000, 1.000000000000000000 ) ) ;
#9997=DIRECTION ( 'NONE',  ( 0.000000000000000000, 0.000000000000000000, 1.000000000000000000 ) ) ;
#10002=CARTESIAN_POINT ( 'NONE',  ( 0.000000000000000000, 0.000000000000000000, -6.500000000000000000 ) ) ;
#10005=CIRCLE ( 'NONE', #14606, 0.4999999999999992784 ) ;
#10006=ORIENTED_EDGE ( 'NONE', *, *, #13200, .F. ) ;
#10012=CARTESIAN_POINT ( 'NONE',  ( -29.72853858738272592, 9.133673601486785643, -6.500000000000000000 ) ) ;
#10016=EDGE_LOOP ( 'NONE', ( #17710, #3146, #1165, #18973 ) ) ;
#10022=EDGE_CURVE ( 'NONE', #6810, #24237, #20071, .T. ) ;
#10023=DIRECTION ( 'NONE',  ( 0.000000000000000000, 0.000000000000000000, 1.000000000000000000 ) ) ;
#10024=CIRCLE ( 'NONE', #19236, 0.4999999999999996114 ) ;
#10028=CARTESIAN_POINT ( 'NONE',  ( 0.000000000000000000, 0.000000000000000000, -6.500000000000000000 ) ) ;
#10029=DIRECTION ( 'NONE',  ( -0.000000000000000000, -0.000000000000000000, 1.000000000000000000 ) ) ;
#10033=VERTEX_POINT ( 'NONE', #8893 ) ;
#10035=CARTESIAN_POINT ( 'NONE',  ( 0.000000000000000000, 0.000000000000000000, 1.000000000000000000 ) ) ;
#10037=AXIS2_PLACEMENT_3D ( 'NONE', #2768, #14538, #22518 ) ;
#10041=VERTEX_POINT ( 'NONE', #16877 ) ;
#10042=LINE ( 'NONE', #16193, #3977 ) ;
#10045=ORIENTED_EDGE ( 'NONE', *, *, #20352, .F. ) ;
#10046=EDGE_CURVE ( 'NONE', #4583, #7760, #8812, .T. ) ;
#10047=AXIS2_PLACEMENT_3D ( 'NONE', #19702, #2182, #3882 ) ;
#10049=VERTEX_POINT ( 'NONE', #4712 ) ;
#10051=ORIENTED_EDGE ( 'NONE', *, *, #22674, .F. ) ;
#10052=CARTESIAN_POINT ( 'NONE',  ( 29.41953157733086854, -10.08469938919509801, -2.750000000000000000 ) ) ;
#10053=DIRECTION ( 'NONE',  ( 0.000000000000000000, 0.000000000000000000, 1.000000000000000000 ) ) ;
#10057=CARTESIAN_POINT ( 'NONE',  ( -30.12293631110035363, 7.734255490827311341, 1.000000000000000000 ) ) ;
#10062=CARTESIAN_POINT ( 'NONE',  ( 0.000000000000000000, 0.000000000000000000, -6.500000000000000000 ) ) ;
#10066=DIRECTION ( 'NONE',  ( 1.000000000000000000, 0.000000000000000000, 0.000000000000000000 ) ) ;
#10071=CIRCLE ( 'NONE', #19259, 27.10000000000000142 ) ;
#10074=CYLINDRICAL_SURFACE ( 'NONE', #18491, 0.5000000000000004441 ) ;
#10075=VERTEX_POINT ( 'NONE', #534 ) ;
#10077=CARTESIAN_POINT ( 'NONE',  ( -12.74173596767339767, 28.14012133169338270, -6.500000000000000000 ) ) ;
#10079=VERTEX_POINT ( 'NONE', #8749 ) ;
#10082=ORIENTED_EDGE ( 'NONE', *, *, #576, .F. ) ;
#10083=ORIENTED_EDGE ( 'NONE', *, *, #9367, .T. ) ;
#10085=CIRCLE ( 'NONE', #6336, 0.5000000000000000000 ) ;
#10086=ORIENTED_EDGE ( 'NONE', *, *, #12424, .F. ) ;
#10089=VECTOR ( 'NONE', #4346, 1000.000000000000000 ) ;
#10091=DIRECTION ( 'NONE',  ( 0.000000000000000000, 0.000000000000000000, 1.000000000000000000 ) ) ;
#10093=CIRCLE ( 'NONE', #18052, 0.5000000000000000000 ) ;
#10098=EDGE_CURVE ( 'NONE', #22312, #21505, #5058, .T. ) ;
#10105=ORIENTED_EDGE ( 'NONE', *, *, #11393, .T. ) ;
#10114=VECTOR ( 'NONE', #3201, 1000.000000000000000 ) ;
#10117=VERTEX_POINT ( 'NONE', #2474 ) ;
#10118=CIRCLE ( 'NONE', #4700, 0.5000000000000002220 ) ;
#10121=EDGE_CURVE ( 'NONE', #9415, #1627, #8381, .T. ) ;
#10130=CARTESIAN_POINT ( 'NONE',  ( 27.49048467073858859, 14.54246377227349463, -2.750000000000000000 ) ) ;
#10132=CARTESIAN_POINT ( 'NONE',  ( -23.46296185032681336, 19.82388608118453632, 1.000000000000000000 ) ) ;
#10136=ORIENTED_EDGE ( 'NONE', *, *, #15699, .T. ) ;
#10145=ORIENTED_EDGE ( 'NONE', *, *, #20012, .F. ) ;
#10151=AXIS2_PLACEMENT_3D ( 'NONE', #11144, #12998, #19007 ) ;
#10155=CARTESIAN_POINT ( 'NONE',  ( 30.85476721088027929, 3.897863563849760737, 1.000000000000000000 ) ) ;
#10156=CYLINDRICAL_SURFACE ( 'NONE', #13770, 0.5000000000000004441 ) ;
#10159=ADVANCED_FACE ( 'NONE', ( #21547 ), #17495, .F. ) ;
#10160=CARTESIAN_POINT ( 'NONE',  ( 11.91206721063030649, -28.72825533807137433, 1.000000000000000000 ) ) ;
#10165=DIRECTION ( 'NONE',  ( 0.000000000000000000, 0.000000000000000000, 1.000000000000000000 ) ) ;
#10169=DIRECTION ( 'NONE',  ( 0.9297764858882504591, -0.3681245526846803617, 0.000000000000000000 ) ) ;
#10170=ORIENTED_EDGE ( 'NONE', *, *, #16798, .T. ) ;
#10175=ORIENTED_EDGE ( 'NONE', *, *, #8740, .F. ) ;
#10176=ORIENTED_EDGE ( 'NONE', *, *, #15604, .T. ) ;
#10178=ORIENTED_EDGE ( 'NONE', *, *, #17270, .F. ) ;
#10179=ORIENTED_EDGE ( 'NONE', *, *, #24020, .F. ) ;
#10180=DIRECTION ( 'NONE',  ( 0.000000000000000000, 0.000000000000000000, 1.000000000000000000 ) ) ;
#10184=DIRECTION ( 'NONE',  ( 0.000000000000000000, 0.000000000000000000, 1.000000000000000000 ) ) ;
#10188=ADVANCED_FACE ( 'NONE', ( #7560 ), #5602, .F. ) ;
#10192=DIRECTION ( 'NONE',  ( 1.000000000000000000, 0.000000000000000000, 0.000000000000000000 ) ) ;
#10196=DIRECTION ( 'NONE',  ( 0.000000000000000000, 0.000000000000000000, 1.000000000000000000 ) ) ;
#10199=ORIENTED_EDGE ( 'NONE', *, *, #3452, .T. ) ;
#10202=ORIENTED_EDGE ( 'NONE', *, *, #12366, .F. ) ;
#10203=ORIENTED_EDGE ( 'NONE', *, *, #11555, .F. ) ;
#10208=ORIENTED_EDGE ( 'NONE', *, *, #17759, .T. ) ;
#10215=CARTESIAN_POINT ( 'NONE',  ( -13.24173596767398742, -28.14012133169310559, -6.500000000000000000 ) ) ;
#10224=DIRECTION ( 'NONE',  ( 1.000000000000000000, 0.000000000000000000, 0.000000000000000000 ) ) ;
#10229=ORIENTED_EDGE ( 'NONE', *, *, #18537, .F. ) ;
#10231=ORIENTED_EDGE ( 'NONE', *, *, #20484, .F. ) ;
#10235=CARTESIAN_POINT ( 'NONE',  ( 31.06601413805602263, -1.453535542772716793, 1.000000000000000000 ) ) ;
#10237=CARTESIAN_POINT ( 'NONE',  ( -7.234255490826573265, 30.12293631110053838, -6.500000000000000000 ) ) ;
#10241=CARTESIAN_POINT ( 'NONE',  ( 8.217531866530997320, -29.99470236596036088, -6.500000000000000000 ) ) ;
#10244=ADVANCED_FACE ( 'NONE', ( #19195 ), #13073, .F. ) ;
#10245=AXIS2_PLACEMENT_3D ( 'NONE', #20578, #25250, #2668 ) ;
#10247=EDGE_CURVE ( 'NONE', #23781, #17588, #9672, .T. ) ;
#10250=CARTESIAN_POINT ( 'NONE',  ( 21.28941499438225904, 22.67092431280586240, -6.500000000000000000 ) ) ;
#10251=EDGE_CURVE ( 'NONE', #17688, #12485, #17636, .T. ) ;
#10256=ORIENTED_EDGE ( 'NONE', *, *, #6314, .F. ) ;
#10260=EDGE_LOOP ( 'NONE', ( #8548, #15384, #22956, #12749 ) ) ;
#10261=ORIENTED_EDGE ( 'NONE', *, *, #5399, .T. ) ;
#10262=DIRECTION ( 'NONE',  ( 0.000000000000000000, 0.000000000000000000, 1.000000000000000000 ) ) ;
#10264=DIRECTION ( 'NONE',  ( 0.000000000000000000, 0.000000000000000000, 1.000000000000000000 ) ) ;
#10266=ORIENTED_EDGE ( 'NONE', *, *, #20012, .T. ) ;
#10271=EDGE_CURVE ( 'NONE', #6029, #15121, #25607, .T. ) ;
#10272=DIRECTION ( 'NONE',  ( 0.000000000000000000, 0.000000000000000000, 1.000000000000000000 ) ) ;
#10273=PRODUCT_DEFINITION ( 'UNKNOWN', '', #15226, #14902 ) ;
#10278=DIRECTION ( 'NONE',  ( 1.000000000000000000, 0.000000000000000000, 0.000000000000000000 ) ) ;
#10283=EDGE_LOOP ( 'NONE', ( #9640, #5004, #17834, #17430 ) ) ;
#10284=CARTESIAN_POINT ( 'NONE',  ( 6.317933499823438659, 30.45149776762727356, -6.500000000000000000 ) ) ;
#10289=VERTEX_POINT ( 'NONE', #19455 ) ;
#10293=CARTESIAN_POINT ( 'NONE',  ( 5.827558883616049457, 30.54913349766221842, -6.500000000000000000 ) ) ;
#10296=ORIENTED_EDGE ( 'NONE', *, *, #13854, .T. ) ;
#10297=EDGE_LOOP ( 'NONE', ( #1624, #6483, #22505, #14767 ) ) ;
#10299=ORIENTED_EDGE ( 'NONE', *, *, #2204, .T. ) ;
#10303=CARTESIAN_POINT ( 'NONE',  ( -5.827558883615604479, 30.54913349766230724, 1.000000000000000000 ) ) ;
#10308=DIRECTION ( 'NONE',  ( 1.000000000000000000, 0.000000000000000000, 0.000000000000000000 ) ) ;
#10311=DIRECTION ( 'NONE',  ( 1.000000000000000000, 0.000000000000000000, 0.000000000000000000 ) ) ;
#10312=DIRECTION ( 'NONE',  ( -1.000000000000000000, 0.000000000000000000, 0.000000000000000000 ) ) ;
#10313=DIRECTION ( 'NONE',  ( 0.000000000000000000, 0.000000000000000000, 1.000000000000000000 ) ) ;
#10317=CARTESIAN_POINT ( 'NONE',  ( 12.78762572734049030, -28.34936733434204470, 1.000000000000000000 ) ) ;
#10320=VERTEX_POINT ( 'NONE', #2199 ) ;
#10321=CYLINDRICAL_SURFACE ( 'NONE', #13768, 0.5000000000000004441 ) ;
#10323=VERTEX_POINT ( 'NONE', #17758 ) ;
#10324=VERTEX_POINT ( 'NONE', #19717 ) ;
#10325=VERTEX_POINT ( 'NONE', #7944 ) ;
#10326=ORIENTED_EDGE ( 'NONE', *, *, #21775, .F. ) ;
#10329=FACE_OUTER_BOUND ( 'NONE', #25268, .T. ) ;
#10336=LINE ( 'NONE', #18333, #13408 ) ;
#10338=DIRECTION ( 'NONE',  ( 1.000000000000000000, 0.000000000000000000, 0.000000000000000000 ) ) ;
#10343=CYLINDRICAL_SURFACE ( 'NONE', #4094, 31.10000000000000142 ) ;
#10344=ORIENTED_EDGE ( 'NONE', *, *, #20164, .T. ) ;
#10347=ADVANCED_FACE ( 'NONE', ( #25856 ), #4016, .F. ) ;
#10349=CARTESIAN_POINT ( 'NONE',  ( 0.4999838450258491940, 31.09598070739550124, 1.000000000000000000 ) ) ;
#10353=EDGE_CURVE ( 'NONE', #25487, #8252, #18431, .T. ) ;
#10354=AXIS2_PLACEMENT_3D ( 'NONE', #10410, #4293, #24424 ) ;
#10355=DIRECTION ( 'NONE',  ( 0.000000000000000000, 0.000000000000000000, 1.000000000000000000 ) ) ;
#10359=CARTESIAN_POINT ( 'NONE',  ( -14.54246377227330456, 27.49048467073868451, 1.000000000000000000 ) ) ;
#10360=AXIS2_PLACEMENT_3D ( 'NONE', #14696, #12453, #701 ) ;
#10367=CIRCLE ( 'NONE', #17080, 0.5000000000000004441 ) ;
#10372=VECTOR ( 'NONE', #24790, 1000.000000000000000 ) ;
#10376=VERTEX_POINT ( 'NONE', #11982 ) ;
#10380=ORIENTED_EDGE ( 'NONE', *, *, #2915, .T. ) ;
#10381=ORIENTED_EDGE ( 'NONE', *, *, #20451, .T. ) ;
#10382=CARTESIAN_POINT ( 'NONE',  ( 0.000000000000000000, 0.000000000000000000, 1.000000000000000000 ) ) ;
#10384=CARTESIAN_POINT ( 'NONE',  ( -30.91344420362543843, 3.401318489841417048, -6.500000000000000000 ) ) ;
#10385=CARTESIAN_POINT ( 'NONE',  ( -5.327558883615603591, 30.54913349766230724, -6.500000000000000000 ) ) ;
#10386=EDGE_CURVE ( 'NONE', #9389, #16191, #9897, .T. ) ;
#10388=VERTEX_POINT ( 'NONE', #13698 ) ;
#10392=AXIS2_PLACEMENT_3D ( 'NONE', #9913, #23919, #11998 ) ;
#10393=CARTESIAN_POINT ( 'NONE',  ( -9.133673601486176352, 29.72853858738290711, 1.000000000000000000 ) ) ;
#10404=ADVANCED_FACE ( 'NONE', ( #11737 ), #4283, .T. ) ;
#10410=CARTESIAN_POINT ( 'NONE',  ( 0.000000000000000000, 0.000000000000000000, 1.000000000000000000 ) ) ;
#10415=ORIENTED_EDGE ( 'NONE', *, *, #23484, .T. ) ;
#10419=DIRECTION ( 'NONE',  ( 0.000000000000000000, 0.000000000000000000, 1.000000000000000000 ) ) ;
#10421=CIRCLE ( 'NONE', #11680, 31.10000000000000142 ) ;
#10422=EDGE_CURVE ( 'NONE', #22500, #27, #16060, .T. ) ;
#10423=AXIS2_PLACEMENT_3D ( 'NONE', #8157, #12596, #20573 ) ;
#10426=EDGE_LOOP ( 'NONE', ( #19252, #20425, #25745, #6180 ) ) ;
#10428=ORIENTED_EDGE ( 'NONE', *, *, #14693, .T. ) ;
#10430=CARTESIAN_POINT ( 'NONE',  ( 29.99470236596032535, 8.217531866531109230, -2.750000000000000000 ) ) ;
#10433=VECTOR ( 'NONE', #4969, 1000.000000000000000 ) ;
#10435=EDGE_CURVE ( 'NONE', #14766, #19279, #4642, .T. ) ;
#10442=AXIS2_PLACEMENT_3D ( 'NONE', #11926, #16391, #17955 ) ;
#10443=CARTESIAN_POINT ( 'NONE',  ( 0.000000000000000000, 0.000000000000000000, 0.000000000000000000 ) ) ;
#10447=CYLINDRICAL_SURFACE ( 'NONE', #21633, 0.5000000000000004441 ) ;
#10451=DIRECTION ( 'NONE',  ( 0.000000000000000000, 0.000000000000000000, 1.000000000000000000 ) ) ;
#10452=CIRCLE ( 'NONE', #453, 31.10000000000000142 ) ;
#10453=DIRECTION ( 'NONE',  ( 0.3681245526846875782, 0.9297764858882475725, 0.000000000000000000 ) ) ;
#10456=DIRECTION ( 'NONE',  ( 1.000000000000000000, 0.000000000000000000, 0.000000000000000000 ) ) ;
#10458=ORIENTED_EDGE ( 'NONE', *, *, #18411, .T. ) ;
#10460=VERTEX_POINT ( 'NONE', #20621 ) ;
#10471=ADVANCED_FACE ( 'NONE', ( #4801 ), #2966, .T. ) ;
#10473=CARTESIAN_POINT ( 'NONE',  ( 30.45149776762729488, 6.317933499823327637, 1.000000000000000000 ) ) ;
#10476=CIRCLE ( 'NONE', #12145, 0.5000000000000001110 ) ;
#10477=CARTESIAN_POINT ( 'NONE',  ( 27.10000000000000142, 3.318792825689327485E-15, 1.000000000000000000 ) ) ;
#10481=DIRECTION ( 'NONE',  ( 0.000000000000000000, 0.000000000000000000, 1.000000000000000000 ) ) ;
#10487=DIRECTION ( 'NONE',  ( 1.000000000000000000, 0.000000000000000000, 0.000000000000000000 ) ) ;
#10488=VERTEX_POINT ( 'NONE', #6886 ) ;
#10494=VERTEX_POINT ( 'NONE', #22587 ) ;
#10495=DIRECTION ( 'NONE',  ( 1.000000000000000000, 0.000000000000000000, 0.000000000000000000 ) ) ;
#10498=AXIS2_PLACEMENT_3D ( 'NONE', #12751, #18371, #2409 ) ;
#10504=CYLINDRICAL_SURFACE ( 'NONE', #15978, 0.5000000000000004441 ) ;
#10505=AXIS2_PLACEMENT_3D ( 'NONE', #19785, #13645, #25676 ) ;
#10506=EDGE_CURVE ( 'NONE', #23030, #14350, #18020, .T. ) ;
#10509=CARTESIAN_POINT ( 'NONE',  ( 0.000000000000000000, 0.000000000000000000, 1.000000000000000000 ) ) ;
#10512=AXIS2_PLACEMENT_3D ( 'NONE', #17678, #3800, #11780 ) ;
#10519=AXIS2_PLACEMENT_3D ( 'NONE', #20882, #4531, #8595 ) ;
#10526=VERTEX_POINT ( 'NONE', #4526 ) ;
#10528=CARTESIAN_POINT ( 'NONE',  ( -16.23990935651735867, -26.52310962334733446, -2.750000000000000000 ) ) ;
#10529=VECTOR ( 'NONE', #8772, 1000.000000000000000 ) ;
#10530=CARTESIAN_POINT ( 'NONE',  ( -27.00874656207282953, 15.41874213889444079, -6.500000000000000000 ) ) ;
#10532=ORIENTED_EDGE ( 'NONE', *, *, #14006, .T. ) ;
#10535=DIRECTION ( 'NONE',  ( 0.000000000000000000, 0.000000000000000000, 1.000000000000000000 ) ) ;
#10538=EDGE_CURVE ( 'NONE', #18550, #1524, #10071, .T. ) ;
#10544=DIRECTION ( 'NONE',  ( 0.000000000000000000, 0.000000000000000000, 1.000000000000000000 ) ) ;
#10552=ORIENTED_EDGE ( 'NONE', *, *, #15269, .T. ) ;
#10562=AXIS2_PLACEMENT_3D ( 'NONE', #23160, #5743, #21703 ) ;
#10563=VERTEX_POINT ( 'NONE', #2579 ) ;
#10565=ORIENTED_EDGE ( 'NONE', *, *, #9213, .T. ) ;
#10566=ORIENTED_EDGE ( 'NONE', *, *, #19948, .F. ) ;
#10567=DIRECTION ( 'NONE',  ( 0.000000000000000000, 0.000000000000000000, 1.000000000000000000 ) ) ;
#10570=ADVANCED_FACE ( 'NONE', ( #743 ), #12649, .T. ) ;
#10572=CARTESIAN_POINT ( 'NONE',  ( -30.54913349766215802, 5.827558883616378083, 1.000000000000000000 ) ) ;
#10580=CARTESIAN_POINT ( 'NONE',  ( 28.91604871112457076, -11.44867358849361416, -6.500000000000000000 ) ) ;
#10581=EDGE_CURVE ( 'NONE', #4812, #12308, #18100, .T. ) ;
#10583=FACE_OUTER_BOUND ( 'NONE', #10016, .T. ) ;
#10584=CARTESIAN_POINT ( 'NONE',  ( -31.03863125411927371, -1.952785157361310198, -6.500000000000000000 ) ) ;
#10592=ORIENTED_EDGE ( 'NONE', *, *, #1508, .T. ) ;
#10594=VERTEX_POINT ( 'NONE', #8542 ) ;
#10596=ORIENTED_EDGE ( 'NONE', *, *, #11954, .T. ) ;
#10597=VERTEX_POINT ( 'NONE', #18341 ) ;
#10598=ORIENTED_EDGE ( 'NONE', *, *, #18971, .F. ) ;
#10599=LINE ( 'NONE', #22646, #7207 ) ;
#10602=VERTEX_POINT ( 'NONE', #2386 ) ;
#10603=DIRECTION ( 'NONE',  ( 0.9048270524660262382, 0.4257792915650585042, 0.000000000000000000 ) ) ;
#10608=DIRECTION ( 'NONE',  ( 0.000000000000000000, -0.000000000000000000, 1.000000000000000000 ) ) ;
#10616=DIRECTION ( 'NONE',  ( 1.000000000000000000, 0.000000000000000000, 0.000000000000000000 ) ) ;
#10617=ORIENTED_EDGE ( 'NONE', *, *, #22743, .T. ) ;
#10622=ORIENTED_EDGE ( 'NONE', *, *, #9458, .F. ) ;
#10625=CYLINDRICAL_SURFACE ( 'NONE', #869, 0.5000000000000004441 ) ;
#10626=ORIENTED_EDGE ( 'NONE', *, *, #9292, .T. ) ;
#10628=CARTESIAN_POINT ( 'NONE',  ( -5.827558883615604479, 30.54913349766230724, -6.500000000000000000 ) ) ;
#10629=ORIENTED_EDGE ( 'NONE', *, *, #25723, .T. ) ;
#10635=DIRECTION ( 'NONE',  ( 1.000000000000000000, 0.000000000000000000, 0.000000000000000000 ) ) ;
#10640=CARTESIAN_POINT ( 'NONE',  ( 0.000000000000000000, 0.000000000000000000, 1.000000000000000000 ) ) ;
#10641=FACE_OUTER_BOUND ( 'NONE', #895, .T. ) ;
#10643=EDGE_CURVE ( 'NONE', #7884, #23630, #15515, .T. ) ;
#10652=DIRECTION ( 'NONE',  ( 1.000000000000000000, 0.000000000000000000, 0.000000000000000000 ) ) ;
#10657=EDGE_CURVE ( 'NONE', #18582, #6126, #7579, .T. ) ;
#10658=DIRECTION ( 'NONE',  ( 1.000000000000000000, 0.000000000000000000, 0.000000000000000000 ) ) ;
#10663=CARTESIAN_POINT ( 'NONE',  ( 31.06601413805602263, 1.453535542772627087, 1.000000000000000000 ) ) ;
#10666=DIRECTION ( 'NONE',  ( 0.000000000000000000, 0.000000000000000000, 1.000000000000000000 ) ) ;
#10670=EDGE_CURVE ( 'NONE', #12491, #2759, #20959, .T. ) ;
#10682=CARTESIAN_POINT ( 'NONE',  ( -12.78762572734076919, -28.34936733434192035, -2.750000000000000000 ) ) ;
#10684=CARTESIAN_POINT ( 'NONE',  ( 31.00322564728514507, 2.451530025009026392, -6.500000000000000000 ) ) ;
#10686=ORIENTED_EDGE ( 'NONE', *, *, #7865, .T. ) ;
#10691=CARTESIAN_POINT ( 'NONE',  ( -29.57785765677917311, 9.610428525061202265, -6.500000000000000000 ) ) ;
#10693=EDGE_CURVE ( 'NONE', #16373, #16896, #474, .T. ) ;
#10698=DIRECTION ( 'NONE',  ( -0.000000000000000000, -0.000000000000000000, 1.000000000000000000 ) ) ;
#10712=LINE ( 'NONE', #8519, #24593 ) ;
#10714=EDGE_CURVE ( 'NONE', #20266, #89, #8657, .T. ) ;
#10715=ORIENTED_EDGE ( 'NONE', *, *, #7734, .F. ) ;
#10716=ORIENTED_EDGE ( 'NONE', *, *, #17537, .F. ) ;
#10717=VERTEX_POINT ( 'NONE', #24997 ) ;
#10720=ADVANCED_FACE ( 'NONE', ( #6833 ), #20564, .F. ) ;
#10721=ORIENTED_EDGE ( 'NONE', *, *, #10670, .T. ) ;
#10727=EDGE_CURVE ( 'NONE', #21926, #21953, #15073, .T. ) ;
#10728=DIRECTION ( 'NONE',  ( 0.000000000000000000, 0.000000000000000000, 1.000000000000000000 ) ) ;
#10731=DIRECTION ( 'NONE',  ( 1.000000000000000000, 0.000000000000000000, 0.000000000000000000 ) ) ;
#10738=DIRECTION ( 'NONE',  ( 0.000000000000000000, 0.000000000000000000, 1.000000000000000000 ) ) ;
#10741=ORIENTED_EDGE ( 'NONE', *, *, #532, .F. ) ;
#10744=ORIENTED_EDGE ( 'NONE', *, *, #3069, .T. ) ;
#10750=EDGE_LOOP ( 'NONE', ( #12562, #16232, #3677, #24467 ) ) ;
#10751=DIRECTION ( 'NONE',  ( 0.000000000000000000, 0.000000000000000000, 1.000000000000000000 ) ) ;
#10755=AXIS2_PLACEMENT_3D ( 'NONE', #4082, #5927, #11931 ) ;
#10760=EDGE_CURVE ( 'NONE', #4269, #5905, #2900, .T. ) ;
#10763=LINE ( 'NONE', #6722, #16619 ) ;
#10764=ORIENTED_EDGE ( 'NONE', *, *, #23066, .F. ) ;
#10773=ORIENTED_EDGE ( 'NONE', *, *, #17833, .T. ) ;
#10774=VERTEX_POINT ( 'NONE', #955 ) ;
#10776=AXIS2_PLACEMENT_3D ( 'NONE', #691, #10481, #4863 ) ;
#10781=FACE_OUTER_BOUND ( 'NONE', #20038, .T. ) ;
#10784=EDGE_CURVE ( 'NONE', #16676, #18610, #19340, .T. ) ;
#10791=EDGE_CURVE ( 'NONE', #24696, #16618, #13407, .T. ) ;
#10792=AXIS2_PLACEMENT_3D ( 'NONE', #9220, #3079, #15118 ) ;
#10793=DIRECTION ( 'NONE',  ( -0.000000000000000000, -0.000000000000000000, 1.000000000000000000 ) ) ;
#10796=CARTESIAN_POINT ( 'NONE',  ( -29.72853858738291422, -9.133673601486165694, -2.750000000000000000 ) ) ;
#10802=FACE_OUTER_BOUND ( 'NONE', #16504, .T. ) ;
#10809=CYLINDRICAL_SURFACE ( 'NONE', #21705, 0.5000000000000004441 ) ;
#10810=ORIENTED_EDGE ( 'NONE', *, *, #10839, .T. ) ;
#10812=CIRCLE ( 'NONE', #12920, 31.10000000000000142 ) ;
#10813=ORIENTED_EDGE ( 'NONE', *, *, #21784, .T. ) ;
#10816=ORIENTED_EDGE ( 'NONE', *, *, #15631, .T. ) ;
#10817=DIRECTION ( 'NONE',  ( 1.000000000000000000, 0.000000000000000000, 0.000000000000000000 ) ) ;
#10819=AXIS2_PLACEMENT_3D ( 'NONE', #23945, #20386, #22635 ) ;
#10821=EDGE_CURVE ( 'NONE', #12737, #10488, #3517, .T. ) ;
#10822=EDGE_CURVE ( 'NONE', #6671, #21954, #19461, .T. ) ;
#10826=AXIS2_PLACEMENT_3D ( 'NONE', #1513, #15513, #17084 ) ;
#10829=AXIS2_PLACEMENT_3D ( 'NONE', #20499, #254, #8222 ) ;
#10830=DIRECTION ( 'NONE',  ( -0.8763066800438602533, 0.4817536741017213187, 0.000000000000000000 ) ) ;
#10836=CARTESIAN_POINT ( 'NONE',  ( 0.000000000000000000, 0.000000000000000000, 1.000000000000000000 ) ) ;
#10837=VECTOR ( 'NONE', #11862, 1000.000000000000000 ) ;
#10838=DIRECTION ( 'NONE',  ( 1.000000000000000000, 0.000000000000000000, 0.000000000000000000 ) ) ;
#10839=EDGE_CURVE ( 'NONE', #19344, #4678, #10476, .T. ) ;
#10845=DIRECTION ( 'NONE',  ( -0.4817536741017063306, 0.8763066800438685799, 0.000000000000000000 ) ) ;
#10847=ORIENTED_EDGE ( 'NONE', *, *, #11148, .F. ) ;
#10848=VECTOR ( 'NONE', #14791, 1000.000000000000000 ) ;
#10849=EDGE_LOOP ( 'NONE', ( #13213, #20083, #23061, #15725 ) ) ;
#10850=ORIENTED_EDGE ( 'NONE', *, *, #10953, .T. ) ;
#10851=ORIENTED_EDGE ( 'NONE', *, *, #9696, .T. ) ;
#10852=DIRECTION ( 'NONE',  ( 0.000000000000000000, 0.000000000000000000, 1.000000000000000000 ) ) ;
#10864=DIRECTION ( 'NONE',  ( -0.9921147013144785420, -0.1253332335642980688, 0.000000000000000000 ) ) ;
#10865=CARTESIAN_POINT ( 'NONE',  ( -30.24338421796775123, 7.248980000274508839, -6.500000000000000000 ) ) ;
#10869=FACE_OUTER_BOUND ( 'NONE', #3580, .T. ) ;
#10870=FACE_OUTER_BOUND ( 'NONE', #7763, .T. ) ;
#10881=AXIS2_PLACEMENT_3D ( 'NONE', #9770, #17746, #23890 ) ;
#10885=CARTESIAN_POINT ( 'NONE',  ( 23.96296185032708337, 19.82388608118420237, -6.500000000000000000 ) ) ;
#10886=CIRCLE ( 'NONE', #20934, 31.10000000000000142 ) ;
#10892=CARTESIAN_POINT ( 'NONE',  ( -30.85476721088022600, 3.897863563850190616, -6.500000000000000000 ) ) ;
#10897=CARTESIAN_POINT ( 'NONE',  ( -21.65113613650359525, -22.32573188046897172, -6.500000000000000000 ) ) ;
#10898=AXIS2_PLACEMENT_3D ( 'NONE', #20439, #2537, #18506 ) ;
#10899=ORIENTED_EDGE ( 'NONE', *, *, #23472, .F. ) ;
#10903=AXIS2_PLACEMENT_3D ( 'NONE', #5071, #4813, #16585 ) ;
#10905=AXIS2_PLACEMENT_3D ( 'NONE', #17260, #25228, #11481 ) ;
#10906=CARTESIAN_POINT ( 'NONE',  ( 0.000000000000000000, 0.000000000000000000, -6.500000000000000000 ) ) ;
#10909=ADVANCED_FACE ( 'NONE', ( #4409 ), #4022, .F. ) ;
#10915=DIRECTION ( 'NONE',  ( 0.000000000000000000, 0.000000000000000000, 1.000000000000000000 ) ) ;
#10921=EDGE_CURVE ( 'NONE', #22990, #21955, #10886, .T. ) ;
#10922=CIRCLE ( 'NONE', #22624, 0.4999999999999997780 ) ;
#10925=CIRCLE ( 'NONE', #15966, 0.5000000000000009992 ) ;
#10926=CIRCLE ( 'NONE', #23064, 31.10000000000000142 ) ;
#10928=FACE_OUTER_BOUND ( 'NONE', #5646, .T. ) ;
#10930=DIRECTION ( 'NONE',  ( 0.9685831611286337406, 0.2486898871648445808, 0.000000000000000000 ) ) ;
#10934=DIRECTION ( 'NONE',  ( -0.000000000000000000, -0.000000000000000000, 1.000000000000000000 ) ) ;
#10938=DIRECTION ( 'NONE',  ( 1.000000000000000000, 0.000000000000000000, 0.000000000000000000 ) ) ;
#10940=DIRECTION ( 'NONE',  ( 0.000000000000000000, 0.000000000000000000, 1.000000000000000000 ) ) ;
#10943=CARTESIAN_POINT ( 'NONE',  ( 21.65113613650343538, 22.32573188046912449, -2.750000000000000000 ) ) ;
#10944=ORIENTED_EDGE ( 'NONE', *, *, #4324, .F. ) ;
#10945=DIRECTION ( 'NONE',  ( 1.000000000000000000, 0.000000000000000000, 0.000000000000000000 ) ) ;
#10950=ORIENTED_EDGE ( 'NONE', *, *, #2339, .T. ) ;
#10951=VECTOR ( 'NONE', #11864, 1000.000000000000000 ) ;
#10953=EDGE_CURVE ( 'NONE', #20598, #2083, #18163, .T. ) ;
#10954=CIRCLE ( 'NONE', #1780, 0.5000000000000006661 ) ;
#10957=ORIENTED_EDGE ( 'NONE', *, *, #19375, .F. ) ;
#10958=ORIENTED_EDGE ( 'NONE', *, *, #13384, .F. ) ;
#10960=ADVANCED_FACE ( 'NONE', ( #242 ), #366, .T. ) ;
#10962=DIRECTION ( 'NONE',  ( -0.000000000000000000, -0.000000000000000000, 1.000000000000000000 ) ) ;
#10967=CIRCLE ( 'NONE', #22673, 0.4999999999999999445 ) ;
#10968=CARTESIAN_POINT ( 'NONE',  ( -29.09636799667067564, 10.98232076577254368, -2.750000000000000000 ) ) ;
#10975=DIRECTION ( 'NONE',  ( -6.938893903907225222E-15, -1.000000000000000000, 0.000000000000000000 ) ) ;
#10980=AXIS2_PLACEMENT_3D ( 'NONE', #12077, #12344, #2156 ) ;
#10982=ADVANCED_FACE ( 'NONE', ( #16186 ), #6242, .F. ) ;
#10986=DIRECTION ( 'NONE',  ( 1.000000000000000000, 0.000000000000000000, 0.000000000000000000 ) ) ;
#10987=ORIENTED_EDGE ( 'NONE', *, *, #23354, .F. ) ;
#10989=AXIS2_PLACEMENT_3D ( 'NONE', #11628, #23067, #25015 ) ;
#10992=ORIENTED_EDGE ( 'NONE', *, *, #10422, .F. ) ;
#10993=ORIENTED_EDGE ( 'NONE', *, *, #13854, .F. ) ;
#10995=EDGE_LOOP ( 'NONE', ( #11076, #11556, #14886, #16161 ) ) ;
#10998=EDGE_CURVE ( 'NONE', #13848, #16720, #14251, .T. ) ;
#11001=DIRECTION ( 'NONE',  ( 0.000000000000000000, 0.000000000000000000, 1.000000000000000000 ) ) ;
#11014=ORIENTED_EDGE ( 'NONE', *, *, #18566, .F. ) ;
#11018=ORIENTED_EDGE ( 'NONE', *, *, #11945, .F. ) ;
#11019=CYLINDRICAL_SURFACE ( 'NONE', #20474, 0.5000000000000004441 ) ;
#11020=ORIENTED_EDGE ( 'NONE', *, *, #8349, .F. ) ;
#11024=ORIENTED_EDGE ( 'NONE', *, *, #13478, .T. ) ;
#11025=CARTESIAN_POINT ( 'NONE',  ( 26.25859848311271705, 16.66421332384673804, 1.000000000000000000 ) ) ;
#11027=DIRECTION ( 'NONE',  ( -0.000000000000000000, -0.000000000000000000, 1.000000000000000000 ) ) ;
#11028=CARTESIAN_POINT ( 'NONE',  ( -29.09636799667091367, -10.98232076577190774, -6.500000000000000000 ) ) ;
#11029=CARTESIAN_POINT ( 'NONE',  ( -20.78941499438242246, -22.67092431280570963, 1.000000000000000000 ) ) ;
#11031=CYLINDRICAL_SURFACE ( 'NONE', #859, 31.10000000000000142 ) ;
#11035=DIRECTION ( 'NONE',  ( 0.000000000000000000, 0.000000000000000000, 1.000000000000000000 ) ) ;
#11036=ORIENTED_EDGE ( 'NONE', *, *, #10046, .T. ) ;
#11046=ADVANCED_FACE ( 'NONE', ( #16578 ), #20754, .F. ) ;
#11052=EDGE_CURVE ( 'NONE', #20454, #21926, #14675, .T. ) ;
#11061=DIRECTION ( 'NONE',  ( 0.000000000000000000, 0.000000000000000000, 1.000000000000000000 ) ) ;
#11063=CARTESIAN_POINT ( 'NONE',  ( 4.393401135980992578, 30.78811501957144969, 1.000000000000000000 ) ) ;
#11066=LINE ( 'NONE', #1401, #23854 ) ;
#11068=DIRECTION ( 'NONE',  ( 0.000000000000000000, 0.000000000000000000, 1.000000000000000000 ) ) ;
#11071=ORIENTED_EDGE ( 'NONE', *, *, #14865, .T. ) ;
#11076=ORIENTED_EDGE ( 'NONE', *, *, #20753, .F. ) ;
#11078=VERTEX_POINT ( 'NONE', #1012 ) ;
#11080=ORIENTED_EDGE ( 'NONE', *, *, #24826, .F. ) ;
#11087=CARTESIAN_POINT ( 'NONE',  ( 0.000000000000000000, 0.000000000000000000, -6.500000000000000000 ) ) ;
#11089=EDGE_CURVE ( 'NONE', #25532, #5321, #18840, .T. ) ;
#11090=CARTESIAN_POINT ( 'NONE',  ( 0.000000000000000000, 0.000000000000000000, 1.000000000000000000 ) ) ;
#11093=CARTESIAN_POINT ( 'NONE',  ( -30.78811501957148167, -4.393401135980793626, 1.000000000000000000 ) ) ;
#11094=DIRECTION ( 'NONE',  ( 1.000000000000000000, 0.000000000000000000, 0.000000000000000000 ) ) ;
#11095=AXIS2_PLACEMENT_3D ( 'NONE', #10628, #13097, #2530 ) ;
#11099=DIRECTION ( 'NONE',  ( 0.000000000000000000, 0.000000000000000000, 1.000000000000000000 ) ) ;
#11100=DIRECTION ( 'NONE',  ( 0.000000000000000000, 0.000000000000000000, 1.000000000000000000 ) ) ;
#11102=CARTESIAN_POINT ( 'NONE',  ( 0.000000000000000000, 0.000000000000000000, 1.000000000000000000 ) ) ;
#11106=ORIENTED_EDGE ( 'NONE', *, *, #15128, .F. ) ;
#11108=CARTESIAN_POINT ( 'NONE',  ( 25.16042852506090810, 18.28012134629586072, -6.500000000000000000 ) ) ;
#11110=ORIENTED_EDGE ( 'NONE', *, *, #23832, .T. ) ;
#11112=ORIENTED_EDGE ( 'NONE', *, *, #330, .T. ) ;
#11113=ORIENTED_EDGE ( 'NONE', *, *, #5301, .T. ) ;
#11114=FACE_OUTER_BOUND ( 'NONE', #17939, .T. ) ;
#11115=DIRECTION ( 'NONE',  ( 0.000000000000000000, 0.000000000000000000, 1.000000000000000000 ) ) ;
#11122=EDGE_CURVE ( 'NONE', #3398, #17170, #18406, .T. ) ;
#11128=DIRECTION ( 'NONE',  ( 0.000000000000000000, 0.000000000000000000, 1.000000000000000000 ) ) ;
#11130=DIRECTION ( 'NONE',  ( 0.000000000000000000, 0.000000000000000000, 1.000000000000000000 ) ) ;
#11131=CARTESIAN_POINT ( 'NONE',  ( -12.74173596767339767, 28.14012133169338270, 1.000000000000000000 ) ) ;
#11134=ORIENTED_EDGE ( 'NONE', *, *, #782, .F. ) ;
#11135=ORIENTED_EDGE ( 'NONE', *, *, #10714, .T. ) ;
#11139=ORIENTED_EDGE ( 'NONE', *, *, #16990, .F. ) ;
#11142=CARTESIAN_POINT ( 'NONE',  ( 22.32573188046904633, -21.65113613650351709, -6.500000000000000000 ) ) ;
#11144=CARTESIAN_POINT ( 'NONE',  ( -3.897863563850083146, -30.85476721088024021, -6.500000000000000000 ) ) ;
#11146=LINE ( 'NONE', #25161, #4570 ) ;
#11148=EDGE_CURVE ( 'NONE', #13117, #3186, #20069, .T. ) ;
#11151=EDGE_CURVE ( 'NONE', #15884, #1343, #23027, .T. ) ;
#11155=ORIENTED_EDGE ( 'NONE', *, *, #13459, .T. ) ;
#11157=DIRECTION ( 'NONE',  ( -0.000000000000000000, 0.000000000000000000, 1.000000000000000000 ) ) ;
#11158=ADVANCED_FACE ( 'NONE', ( #14874 ), #880, .F. ) ;
#11161=CARTESIAN_POINT ( 'NONE',  ( 4.393401135981119587, 30.78811501957143193, -2.750000000000000000 ) ) ;
#11165=VECTOR ( 'NONE', #15868, 1000.000000000000000 ) ;
#11166=CARTESIAN_POINT ( 'NONE',  ( -13.69242354489172797, -27.92360179968362743, -2.750000000000000000 ) ) ;
#11176=CARTESIAN_POINT ( 'NONE',  ( 0.000000000000000000, 0.000000000000000000, -6.500000000000000000 ) ) ;
#11185=CARTESIAN_POINT ( 'NONE',  ( -22.17092431280609333, -21.28941499438201745, -6.500000000000000000 ) ) ;
#11189=AXIS2_PLACEMENT_3D ( 'NONE', #16217, #19615, #23939 ) ;
#11191=DIRECTION ( 'NONE',  ( -0.9297764858882481276, 0.3681245526846864125, 0.000000000000000000 ) ) ;
#11194=CARTESIAN_POINT ( 'NONE',  ( 0.000000000000000000, 0.000000000000000000, -6.500000000000000000 ) ) ;
#11199=ORIENTED_EDGE ( 'NONE', *, *, #14074, .F. ) ;
#11200=EDGE_CURVE ( 'NONE', #17840, #14500, #21522, .T. ) ;
#11205=VECTOR ( 'NONE', #20749, 1000.000000000000000 ) ;
#11207=CIRCLE ( 'NONE', #19147, 0.4999999999999998890 ) ;
#11208=VECTOR ( 'NONE', #22876, 1000.000000000000000 ) ;
#11210=EDGE_CURVE ( 'NONE', #17608, #585, #17233, .T. ) ;
#11215=DIRECTION ( 'NONE',  ( 0.000000000000000000, 0.000000000000000000, 1.000000000000000000 ) ) ;
#11216=FACE_OUTER_BOUND ( 'NONE', #16165, .T. ) ;
#11217=DIRECTION ( 'NONE',  ( -0.000000000000000000, -0.000000000000000000, 1.000000000000000000 ) ) ;
#11221=DIRECTION ( 'NONE',  ( -0.000000000000000000, -0.000000000000000000, 1.000000000000000000 ) ) ;
#11223=AXIS2_PLACEMENT_3D ( 'NONE', #6082, #211, #15903 ) ;
#11228=LINE ( 'NONE', #13335, #2926 ) ;
#11230=ORIENTED_EDGE ( 'NONE', *, *, #6520, .T. ) ;
#11231=EDGE_CURVE ( 'NONE', #6673, #13859, #11066, .T. ) ;
#11233=ORIENTED_EDGE ( 'NONE', *, *, #2161, .F. ) ;
#11235=ORIENTED_EDGE ( 'NONE', *, *, #14804, .T. ) ;
#11240=DIRECTION ( 'NONE',  ( 0.000000000000000000, 0.000000000000000000, 1.000000000000000000 ) ) ;
#11247=CARTESIAN_POINT ( 'NONE',  ( -31.00322564728516639, -2.451530025008796798, -6.500000000000000000 ) ) ;
#11250=DIRECTION ( 'NONE',  ( 1.000000000000000000, 0.000000000000000000, 0.000000000000000000 ) ) ;
#11251=CYLINDRICAL_SURFACE ( 'NONE', #16209, 0.5000000000000004441 ) ;
#11256=AXIS2_PLACEMENT_3D ( 'NONE', #14719, #17550, #4779 ) ;
#11261=ORIENTED_EDGE ( 'NONE', *, *, #23187, .F. ) ;
#11262=CARTESIAN_POINT ( 'NONE',  ( 0.000000000000000000, 0.000000000000000000, 1.000000000000000000 ) ) ;
#11265=EDGE_CURVE ( 'NONE', #14631, #6939, #7989, .T. ) ;
#11266=ORIENTED_EDGE ( 'NONE', *, *, #6733, .F. ) ;
#11267=DIRECTION ( 'NONE',  ( 0.000000000000000000, 0.000000000000000000, 1.000000000000000000 ) ) ;
#11268=VECTOR ( 'NONE', #5053, 1000.000000000000000 ) ;
#11269=EDGE_CURVE ( 'NONE', #10289, #5651, #3603, .T. ) ;
#11270=EDGE_LOOP ( 'NONE', ( #18076, #1354, #11110, #20395 ) ) ;
#11276=DIRECTION ( 'NONE',  ( 1.000000000000000000, 0.000000000000000000, 0.000000000000000000 ) ) ;
#11277=DIRECTION ( 'NONE',  ( 1.000000000000000000, 0.000000000000000000, 0.000000000000000000 ) ) ;
#11280=CIRCLE ( 'NONE', #14635, 0.5000000000000006661 ) ;
#11281=CARTESIAN_POINT ( 'NONE',  ( -30.24338421796775123, 7.248980000274508839, -2.750000000000000000 ) ) ;
#11285=AXIS2_PLACEMENT_3D ( 'NONE', #7753, #15132, #5780 ) ;
#11287=FACE_OUTER_BOUND ( 'NONE', #6395, .T. ) ;
#11294=CIRCLE ( 'NONE', #23418, 31.10000000000000142 ) ;
#11298=ORIENTED_EDGE ( 'NONE', *, *, #12543, .F. ) ;
#11300=CIRCLE ( 'NONE', #15902, 0.4999999999999996114 ) ;
#11301=ADVANCED_FACE ( 'NONE', ( #3483 ), #1519, .T. ) ;
#11302=AXIS2_PLACEMENT_3D ( 'NONE', #7041, #4436, #10830 ) ;
#11303=CARTESIAN_POINT ( 'NONE',  ( -27.92360179968358125, 13.69242354489182922, -6.500000000000000000 ) ) ;
#11309=CIRCLE ( 'NONE', #12150, 0.5000000000000007772 ) ;
#11312=EDGE_CURVE ( 'NONE', #23396, #23209, #11315, .T. ) ;
#11313=AXIS2_PLACEMENT_3D ( 'NONE', #7899, #199, #14184 ) ;
#11315=CIRCLE ( 'NONE', #22631, 0.4999999999999998335 ) ;
#11317=DIRECTION ( 'NONE',  ( 1.000000000000000000, 0.000000000000000000, 0.000000000000000000 ) ) ;
#11319=CARTESIAN_POINT ( 'NONE',  ( -26.25859848311247902, 16.66421332384710752, 1.000000000000000000 ) ) ;
#11325=DIRECTION ( 'NONE',  ( 0.000000000000000000, 0.000000000000000000, 1.000000000000000000 ) ) ;
#11328=ORIENTED_EDGE ( 'NONE', *, *, #16240, .F. ) ;
#11335=CIRCLE ( 'NONE', #18467, 31.10000000000000142 ) ;
#11338=EDGE_LOOP ( 'NONE', ( #255, #9914, #7091, #14950 ) ) ;
#11339=ORIENTED_EDGE ( 'NONE', *, *, #15078, .T. ) ;
#11343=CIRCLE ( 'NONE', #14701, 0.5000000000000003331 ) ;
#11344=EDGE_CURVE ( 'NONE', #9390, #12699, #5576, .T. ) ;
#11346=AXIS2_PLACEMENT_3D ( 'NONE', #22415, #16666, #24775 ) ;
#11347=DIRECTION ( 'NONE',  ( 0.000000000000000000, 0.000000000000000000, 1.000000000000000000 ) ) ;
#11351=CARTESIAN_POINT ( 'NONE',  ( 0.000000000000000000, 0.000000000000000000, 1.000000000000000000 ) ) ;
#11353=DIRECTION ( 'NONE',  ( 0.000000000000000000, 0.000000000000000000, -1.000000000000000000 ) ) ;
#11355=FACE_OUTER_BOUND ( 'NONE', #3808, .T. ) ;
#11356=DIRECTION ( 'NONE',  ( 1.000000000000000000, 0.000000000000000000, 0.000000000000000000 ) ) ;
#11358=ORIENTED_EDGE ( 'NONE', *, *, #14332, .F. ) ;
#11359=CARTESIAN_POINT ( 'NONE',  ( 18.28012134629577190, -25.16042852506097205, -6.500000000000000000 ) ) ;
#11361=CIRCLE ( 'NONE', #17646, 31.10000000000000142 ) ;
#11364=DIRECTION ( 'NONE',  ( 0.000000000000000000, 0.000000000000000000, -1.000000000000000000 ) ) ;
#11365=ORIENTED_EDGE ( 'NONE', *, *, #3416, .F. ) ;
#11367=AXIS2_PLACEMENT_3D ( 'NONE', #16830, #6876, #22958 ) ;
#11369=DIRECTION ( 'NONE',  ( 1.000000000000000000, 0.000000000000000000, 0.000000000000000000 ) ) ;
#11370=ORIENTED_EDGE ( 'NONE', *, *, #23269, .F. ) ;
#11373=ORIENTED_EDGE ( 'NONE', *, *, #8853, .T. ) ;
#11374=VERTEX_POINT ( 'NONE', #15766 ) ;
#11375=VERTEX_POINT ( 'NONE', #2170 ) ;
#11376=DIRECTION ( 'NONE',  ( 0.000000000000000000, 0.000000000000000000, 1.000000000000000000 ) ) ;
#11377=FACE_OUTER_BOUND ( 'NONE', #10995, .T. ) ;
#11378=VECTOR ( 'NONE', #20246, 1000.000000000000000 ) ;
#11380=DIRECTION ( 'NONE',  ( -0.000000000000000000, -0.000000000000000000, 1.000000000000000000 ) ) ;
#11381=AXIS2_PLACEMENT_3D ( 'NONE', #12725, #20694, #16784 ) ;
#11386=ADVANCED_FACE ( 'NONE', ( #17857 ), #25705, .F. ) ;
#11392=CYLINDRICAL_SURFACE ( 'NONE', #19956, 0.5000000000000002220 ) ;
#11393=EDGE_CURVE ( 'NONE', #15245, #2906, #13010, .T. ) ;
#11394=CARTESIAN_POINT ( 'NONE',  ( 28.34936733434205536, 12.78762572734047254, -6.500000000000000000 ) ) ;
#11401=EDGE_LOOP ( 'NONE', ( #11936, #22007, #5257, #20889 ) ) ;
#11402=DIRECTION ( 'NONE',  ( 1.000000000000000000, 0.000000000000000000, 0.000000000000000000 ) ) ;
#11403=ORIENTED_EDGE ( 'NONE', *, *, #12397, .T. ) ;
#11410=CYLINDRICAL_SURFACE ( 'NONE', #25554, 31.10000000000000142 ) ;
#11412=ORIENTED_EDGE ( 'NONE', *, *, #9613, .F. ) ;
#11415=CARTESIAN_POINT ( 'NONE',  ( -30.35476721088030061, -3.897863563849544466, -6.500000000000000000 ) ) ;
#11419=CARTESIAN_POINT ( 'NONE',  ( 16.23990935651698564, -26.52310962334756184, -2.750000000000000000 ) ) ;
#11420=EDGE_CURVE ( 'NONE', #19518, #25247, #7785, .T. ) ;
#11424=DIRECTION ( 'NONE',  ( 1.000000000000000000, 0.000000000000000000, 0.000000000000000000 ) ) ;
#11427=VERTEX_POINT ( 'NONE', #23875 ) ;
#11432=DIRECTION ( 'NONE',  ( 0.000000000000000000, 0.000000000000000000, 1.000000000000000000 ) ) ;
#11435=ORIENTED_EDGE ( 'NONE', *, *, #1682, .F. ) ;
#11438=DIRECTION ( 'NONE',  ( 0.000000000000000000, 0.000000000000000000, 1.000000000000000000 ) ) ;
#11448=LINE ( 'NONE', #1393, #2908 ) ;
#11450=CARTESIAN_POINT ( 'NONE',  ( 0.000000000000000000, 0.000000000000000000, 1.000000000000000000 ) ) ;
#11452=CARTESIAN_POINT ( 'NONE',  ( -30.04913349766228592, -5.827558883615738594, -6.500000000000000000 ) ) ;
#11459=LINE ( 'NONE', #21526, #22154 ) ;
#11460=ORIENTED_EDGE ( 'NONE', *, *, #2120, .F. ) ;
#11471=ORIENTED_EDGE ( 'NONE', *, *, #17833, .F. ) ;
#11477=SURFACE_STYLE_FILL_AREA ( #5599 ) ;
#11478=EDGE_CURVE ( 'NONE', #4613, #4306, #12091, .T. ) ;
#11479=CARTESIAN_POINT ( 'NONE',  ( 29.57785765677924061, -9.610428525060996208, -6.500000000000000000 ) ) ;
#11481=DIRECTION ( 'NONE',  ( 1.000000000000000000, 0.000000000000000000, 0.000000000000000000 ) ) ;
#11483=DIRECTION ( 'NONE',  ( 0.000000000000000000, 0.000000000000000000, 1.000000000000000000 ) ) ;
#11484=DIRECTION ( 'NONE',  ( 0.000000000000000000, 0.000000000000000000, 1.000000000000000000 ) ) ;
#11485=DIRECTION ( 'NONE',  ( -0.2486898871648584586, -0.9685831611286301879, 0.000000000000000000 ) ) ;
#11491=DIRECTION ( 'NONE',  ( 0.000000000000000000, 0.000000000000000000, 1.000000000000000000 ) ) ;
#11492=LINE ( 'NONE', #7435, #5802 ) ;
#11493=LINE ( 'NONE', #13475, #3471 ) ;
#11494=ORIENTED_EDGE ( 'NONE', *, *, #2766, .T. ) ;
#11496=CARTESIAN_POINT ( 'NONE',  ( -3.897863563849436552, 30.85476721088031482, -6.500000000000000000 ) ) ;
#11498=ORIENTED_EDGE ( 'NONE', *, *, #422, .F. ) ;
#11499=EDGE_CURVE ( 'NONE', #23656, #12264, #17202, .T. ) ;
#11500=ORIENTED_EDGE ( 'NONE', *, *, #14414, .F. ) ;
#11502=ORIENTED_EDGE ( 'NONE', *, *, #20217, .F. ) ;
#11504=FACE_OUTER_BOUND ( 'NONE', #19112, .T. ) ;
#11512=CARTESIAN_POINT ( 'NONE',  ( 0.000000000000000000, 0.000000000000000000, -6.500000000000000000 ) ) ;
#11513=LINE ( 'NONE', #15707, #2186 ) ;
#11516=FACE_OUTER_BOUND ( 'NONE', #22679, .T. ) ;
#11517=CARTESIAN_POINT ( 'NONE',  ( -27.10000000000000142, 0.000000000000000000, 1.000000000000000000 ) ) ;
#11519=DIRECTION ( 'NONE',  ( 1.000000000000000000, 0.000000000000000000, 0.000000000000000000 ) ) ;
#11520=CARTESIAN_POINT ( 'NONE',  ( -25.45105997952931176, -17.87326343783925608, 1.000000000000000000 ) ) ;
#11525=DIRECTION ( 'NONE',  ( -0.000000000000000000, -0.000000000000000000, 1.000000000000000000 ) ) ;
#11527=ADVANCED_FACE ( 'NONE', ( #22418 ), #4638, .F. ) ;
#11530=ORIENTED_EDGE ( 'NONE', *, *, #170, .F. ) ;
#11533=FACE_OUTER_BOUND ( 'NONE', #25687, .T. ) ;
#11534=EDGE_LOOP ( 'NONE', ( #4384, #20967, #12429, #21801 ) ) ;
#11537=LINE ( 'NONE', #23577, #17272 ) ;
#11540=CARTESIAN_POINT ( 'NONE',  ( -1.453535542772826039, -31.06601413805601908, -6.500000000000000000 ) ) ;
#11547=ORIENTED_EDGE ( 'NONE', *, *, #19209, .T. ) ;
#11549=ORIENTED_EDGE ( 'NONE', *, *, #21165, .T. ) ;
#11551=ORIENTED_EDGE ( 'NONE', *, *, #5464, .T. ) ;
#11555=EDGE_CURVE ( 'NONE', #10376, #20210, #15514, .T. ) ;
#11556=ORIENTED_EDGE ( 'NONE', *, *, #16516, .F. ) ;
#11560=CYLINDRICAL_SURFACE ( 'NONE', #16432, 31.10000000000000142 ) ;
#11564=DIRECTION ( 'NONE',  ( -0.000000000000000000, -0.000000000000000000, 1.000000000000000000 ) ) ;
#11567=CARTESIAN_POINT ( 'NONE',  ( -25.16042852506104666, -18.28012134629567598, 1.000000000000000000 ) ) ;
#11568=DIRECTION ( 'NONE',  ( 1.000000000000000000, 0.000000000000000000, 0.000000000000000000 ) ) ;
#11573=DIRECTION ( 'NONE',  ( -0.000000000000000000, 0.000000000000000000, -1.000000000000000000 ) ) ;
#11578=ORIENTED_EDGE ( 'NONE', *, *, #11151, .F. ) ;
#11582=EDGE_LOOP ( 'NONE', ( #15337, #21617, #11370, #2461 ) ) ;
#11587=ORIENTED_EDGE ( 'NONE', *, *, #1479, .F. ) ;
#11592=EDGE_CURVE ( 'NONE', #21926, #20454, #2151, .T. ) ;
#11594=EDGE_CURVE ( 'NONE', #14918, #4583, #21688, .T. ) ;
#11595=AXIS2_PLACEMENT_3D ( 'NONE', #3042, #1076, #1196 ) ;
#11598=DIRECTION ( 'NONE',  ( 0.000000000000000000, 0.000000000000000000, 1.000000000000000000 ) ) ;
#11600=CIRCLE ( 'NONE', #25404, 0.4999999999999999445 ) ;
#11601=CARTESIAN_POINT ( 'NONE',  ( 29.99470236596032535, 8.217531866531109230, 1.000000000000000000 ) ) ;
#11602=CARTESIAN_POINT ( 'NONE',  ( -1.453535542772826039, -31.06601413805601908, 1.000000000000000000 ) ) ;
#11603=LINE ( 'NONE', #13971, #3284 ) ;
#11604=CARTESIAN_POINT ( 'NONE',  ( -22.67092431280609688, -21.28941499438201745, -6.500000000000000000 ) ) ;
#11605=EDGE_LOOP ( 'NONE', ( #22535, #22394, #3816, #19591 ) ) ;
#11615=CARTESIAN_POINT ( 'NONE',  ( -9.610428525060479288, 29.57785765677940404, 1.000000000000000000 ) ) ;
#11616=VERTEX_POINT ( 'NONE', #9668 ) ;
#11621=ORIENTED_EDGE ( 'NONE', *, *, #1898, .F. ) ;
#11623=CYLINDRICAL_SURFACE ( 'NONE', #1364, 31.10000000000000142 ) ;
#11624=LINE ( 'NONE', #15958, #1509 ) ;
#11625=CIRCLE ( 'NONE', #427, 0.5000000000000002220 ) ;
#11627=CIRCLE ( 'NONE', #19149, 0.4999999999999986122 ) ;
#11628=CARTESIAN_POINT ( 'NONE',  ( -25.16042852506064165, 18.28012134629622309, -6.500000000000000000 ) ) ;
#11634=DIRECTION ( 'NONE',  ( 0.000000000000000000, 0.000000000000000000, 1.000000000000000000 ) ) ;
#11638=CIRCLE ( 'NONE', #3702, 0.5000000000000003331 ) ;
#11639=CARTESIAN_POINT ( 'NONE',  ( -14.48253926456298579, 27.25313774936435962, 1.000000000000000000 ) ) ;
#11641=CARTESIAN_POINT ( 'NONE',  ( 26.52310962334744104, 16.23990935651718459, 1.000000000000000000 ) ) ;
#11644=DIRECTION ( 'NONE',  ( 1.000000000000000000, 0.000000000000000000, 0.000000000000000000 ) ) ;
#11648=VERTEX_POINT ( 'NONE', #15426 ) ;
#11649=DIRECTION ( 'NONE',  ( 1.000000000000000000, 0.000000000000000000, 0.000000000000000000 ) ) ;
#11650=ORIENTED_EDGE ( 'NONE', *, *, #2012, .F. ) ;
#11652=DIRECTION ( 'NONE',  ( 1.000000000000000000, 0.000000000000000000, 0.000000000000000000 ) ) ;
#11653=ORIENTED_EDGE ( 'NONE', *, *, #22431, .F. ) ;
#11661=DIRECTION ( 'NONE',  ( 0.000000000000000000, -0.000000000000000000, 1.000000000000000000 ) ) ;
#11662=AXIS2_PLACEMENT_3D ( 'NONE', #1876, #12315, #20023 ) ;
#11668=DIRECTION ( 'NONE',  ( 0.9822872507286911636, 0.1873813145857119722, 0.000000000000000000 ) ) ;
#11669=LINE ( 'NONE', #16958, #3768 ) ;
#11670=AXIS2_PLACEMENT_3D ( 'NONE', #12819, #20791, #22493 ) ;
#11680=AXIS2_PLACEMENT_3D ( 'NONE', #21289, #11347, #1421 ) ;
#11686=ORIENTED_EDGE ( 'NONE', *, *, #16598, .T. ) ;
#11688=CYLINDRICAL_SURFACE ( 'NONE', #1083, 0.5000000000000004441 ) ;
#11689=CIRCLE ( 'NONE', #433, 0.5000000000000003331 ) ;
#11693=DIRECTION ( 'NONE',  ( 0.000000000000000000, 0.000000000000000000, -1.000000000000000000 ) ) ;
#11695=CIRCLE ( 'NONE', #2111, 0.5000000000000006661 ) ;
#11697=CARTESIAN_POINT ( 'NONE',  ( 0.000000000000000000, 0.000000000000000000, -6.500000000000000000 ) ) ;
#11703=DIRECTION ( 'NONE',  ( 0.000000000000000000, 0.000000000000000000, 1.000000000000000000 ) ) ;
#11704=VECTOR ( 'NONE', #24131, 1000.000000000000000 ) ;
#11710=LINE ( 'NONE', #25706, #12248 ) ;
#11722=VECTOR ( 'NONE', #24448, 1000.000000000000000 ) ;
#11725=LINE ( 'NONE', #19824, #9215 ) ;
#11732=AXIS2_PLACEMENT_3D ( 'NONE', #19834, #15791, #24144 ) ;
#11737=FACE_OUTER_BOUND ( 'NONE', #16620, .T. ) ;
#11739=DIRECTION ( 'NONE',  ( 0.000000000000000000, 0.000000000000000000, 1.000000000000000000 ) ) ;
#11741=ADVANCED_FACE ( 'NONE', ( #22068 ), #20110, .T. ) ;
#11754=DIRECTION ( 'NONE',  ( 1.000000000000000000, 0.000000000000000000, 0.000000000000000000 ) ) ;
#11756=ORIENTED_EDGE ( 'NONE', *, *, #8063, .F. ) ;
#11757=ADVANCED_FACE ( 'NONE', ( #23916 ), #2333, .F. ) ;
#11758=CIRCLE ( 'NONE', #16796, 0.5000000000000001110 ) ;
#11759=EDGE_LOOP ( 'NONE', ( #2250, #9209, #5520, #20011 ) ) ;
#11760=ORIENTED_EDGE ( 'NONE', *, *, #20211, .F. ) ;
#11762=ORIENTED_EDGE ( 'NONE', *, *, #21233, .T. ) ;
#11763=DIRECTION ( 'NONE',  ( 0.000000000000000000, 0.000000000000000000, 1.000000000000000000 ) ) ;
#11767=CIRCLE ( 'NONE', #9273, 0.5000000000000001110 ) ;
#11770=CIRCLE ( 'NONE', #516, 0.4999999999999995004 ) ;
#11773=FACE_OUTER_BOUND ( 'NONE', #12490, .T. ) ;
#11774=CARTESIAN_POINT ( 'NONE',  ( 0.000000000000000000, 0.000000000000000000, -6.500000000000000000 ) ) ;
#11780=DIRECTION ( 'NONE',  ( 1.000000000000000000, 0.000000000000000000, 0.000000000000000000 ) ) ;
#11785=CARTESIAN_POINT ( 'NONE',  ( -28.72825533807115050, 11.91206721063083229, -6.500000000000000000 ) ) ;
#11788=VERTEX_POINT ( 'NONE', #12391 ) ;
#11789=CARTESIAN_POINT ( 'NONE',  ( 0.000000000000000000, 0.000000000000000000, 1.000000000000000000 ) ) ;
#11792=ORIENTED_EDGE ( 'NONE', *, *, #23192, .F. ) ;
#11793=DIRECTION ( 'NONE',  ( 0.000000000000000000, 0.000000000000000000, -1.000000000000000000 ) ) ;
#11799=EDGE_CURVE ( 'NONE', #1796, #16142, #19848, .T. ) ;
#11802=CARTESIAN_POINT ( 'NONE',  ( 30.78811501957144969, 4.393401135981008565, 1.000000000000000000 ) ) ;
#11803=DIRECTION ( 'NONE',  ( 1.000000000000000000, 0.000000000000000000, 0.000000000000000000 ) ) ;
#11804=DIRECTION ( 'NONE',  ( -0.9048270524660170233, 0.4257792915650782661, 0.000000000000000000 ) ) ;
#11812=AXIS2_PLACEMENT_3D ( 'NONE', #25267, #7348, #19373 ) ;
#11815=ORIENTED_EDGE ( 'NONE', *, *, #22938, .F. ) ;
#11816=ORIENTED_EDGE ( 'NONE', *, *, #22866, .F. ) ;
#11819=ORIENTED_EDGE ( 'NONE', *, *, #4563, .F. ) ;
#11821=CIRCLE ( 'NONE', #3888, 0.4999999999999997224 ) ;
#11826=CIRCLE ( 'NONE', #5557, 0.5000000000000005551 ) ;
#11828=ORIENTED_EDGE ( 'NONE', *, *, #21358, .F. ) ;
#11829=CARTESIAN_POINT ( 'NONE',  ( 30.91344420362545975, -3.401318489841207882, -6.500000000000000000 ) ) ;
#11830=CARTESIAN_POINT ( 'NONE',  ( -22.17092431280609333, -21.28941499438201745, -6.500000000000000000 ) ) ;
#11832=CYLINDRICAL_SURFACE ( 'NONE', #2568, 0.5000000000000004441 ) ;
#11835=CARTESIAN_POINT ( 'NONE',  ( 0.000000000000000000, 0.000000000000000000, -6.500000000000000000 ) ) ;
#11837=DIRECTION ( 'NONE',  ( -0.000000000000000000, -0.000000000000000000, 1.000000000000000000 ) ) ;
#11845=ORIENTED_EDGE ( 'NONE', *, *, #1835, .T. ) ;
#11849=ORIENTED_EDGE ( 'NONE', *, *, #23095, .T. ) ;
#11852=DIRECTION ( 'NONE',  ( 1.000000000000000000, 0.000000000000000000, 0.000000000000000000 ) ) ;
#11856=ORIENTED_EDGE ( 'NONE', *, *, #11210, .F. ) ;
#11862=DIRECTION ( 'NONE',  ( 0.000000000000000000, 0.000000000000000000, -1.000000000000000000 ) ) ;
#11864=DIRECTION ( 'NONE',  ( 0.000000000000000000, 0.000000000000000000, -1.000000000000000000 ) ) ;
#11866=DIRECTION ( 'NONE',  ( 1.000000000000000000, 0.000000000000000000, 0.000000000000000000 ) ) ;
#11869=FACE_OUTER_BOUND ( 'NONE', #4421, .T. ) ;
#11872=ORIENTED_EDGE ( 'NONE', *, *, #23066, .T. ) ;
#11878=CARTESIAN_POINT ( 'NONE',  ( 1.453535542772610212, 31.06601413805602263, -6.500000000000000000 ) ) ;
#11882=DIRECTION ( 'NONE',  ( 0.000000000000000000, 0.000000000000000000, 1.000000000000000000 ) ) ;
#11884=EDGE_LOOP ( 'NONE', ( #16111, #9345, #8065, #21506 ) ) ;
#11885=VERTEX_POINT ( 'NONE', #20634 ) ;
#11886=ORIENTED_EDGE ( 'NONE', *, *, #25449, .F. ) ;
#11888=DIRECTION ( 'NONE',  ( 0.000000000000000000, 0.000000000000000000, 1.000000000000000000 ) ) ;
#11889=DIRECTION ( 'NONE',  ( -0.4257792915650782661, -0.9048270524660170233, 0.000000000000000000 ) ) ;
#11890=EDGE_CURVE ( 'NONE', #10602, #789, #22191, .T. ) ;
#11892=EDGE_CURVE ( 'NONE', #24369, #2048, #901, .T. ) ;
#11897=DIRECTION ( 'NONE',  ( -0.4257792915650642218, 0.9048270524660235736, 0.000000000000000000 ) ) ;
#11898=CARTESIAN_POINT ( 'NONE',  ( 30.12293631110040693, -7.734255490827107948, -6.500000000000000000 ) ) ;
#11900=CARTESIAN_POINT ( 'NONE',  ( -25.45105997952899912, 17.87326343783971083, 1.000000000000000000 ) ) ;
#11905=CARTESIAN_POINT ( 'NONE',  ( 0.000000000000000000, 0.000000000000000000, 1.000000000000000000 ) ) ;
#11911=ORIENTED_EDGE ( 'NONE', *, *, #7363, .T. ) ;
#11912=EDGE_LOOP ( 'NONE', ( #989, #22466, #9771, #18345, #17864, #23821, #24690, #22183, #7479, #22217, #7968, #3528, #17654, #11412, #23176, #23180, #11760, #4762, #13508, #13482, #9833, #24685, #4333, #22531, #1834, #11587, #15809, #16134, #2524, #22533, #17777, #2778, #2976, #19255, #22397, #8486, #10051, #8940, #23301, #14345, #22671, #8007, #20572, #2115, #9224, #15362, #25589, #9706, #15988, #4059, #18591, #20803, #1735, #8130, #16750, #19090, #4128, #18376, #15780, #13438, #24554, #727, #4503, #9825, #16506, #3672, #6347, #22114, #1737, #17101, #20013, #25597, #2694, #5425, #17549, #2873, #17441, #1370, #13516, #18461, #11845, #16225, #20101, #1860, #19378, #5236, #14231, #2632, #20541, #5555, #1202, #12828, #20271, #23273, #6545, #12303, #25080, #4906, #19938, #14440, #7294, #10592, #17812, #1379, #17745, #19316, #9597, #8599, #15429, #616, #13817, #3645, #9849, #5838, #18586, #22367, #21560, #18501, #19515, #4389, #3388, #8311, #3976, #6640, #16760, #19404, #10082, #21942, #17137, #19976, #24338, #7966, #3850, #12337, #7823, #8000, #2000, #25408, #22368, #16409, #3709, #25479, #549, #22306, #11358, #793, #23922, #4971, #22468, #10266, #795, #9145, #6259, #13914, #10851, #9983, #11036, #22177, #23154, #14237, #12992, #6813, #3526, #14616, #19136, #16945, #19839, #16502, #7326, #14040, #8671, #14553, #18346, #18876, #18110, #2398, #3396, #3078, #6258, #25629, #6250, #18872, #22863, #8666, #3055, #11266, #8312, #11199, #19311, #24824, #21697, #1832, #5415, #824, #7237, #2073, #6601, #14179, #19111, #5420, #4352, #2005, #2598, #12590, #1802, #15621, #10299, #4226, #3916, #18050, #14375, #23852, #25245, #13449, #10176, #3435, #12982, #14145, #2371, #20397, #21451, #15087, #1267, #12846, #8192, #6907, #13505, #17716, #19057, #4876, #18878, #19212, #6870, #13714, #6568, #20324, #15488, #18588, #5545, #13267, #24789, #21988, #9355, #2725, #6293, #11653, #3113, #10598, #23363 ) ) ;
#11913=DIRECTION ( 'NONE',  ( 0.000000000000000000, 0.000000000000000000, 1.000000000000000000 ) ) ;
#11918=VERTEX_POINT ( 'NONE', #18668 ) ;
#11921=EDGE_CURVE ( 'NONE', #11918, #14948, #20890, .T. ) ;
#11923=CARTESIAN_POINT ( 'NONE',  ( 0.000000000000000000, 0.000000000000000000, -6.500000000000000000 ) ) ;
#11925=FACE_OUTER_BOUND ( 'NONE', #18230, .T. ) ;
#11926=CARTESIAN_POINT ( 'NONE',  ( 14.98253926456319007, -27.25313774936425304, -6.500000000000000000 ) ) ;
#11930=CARTESIAN_POINT ( 'NONE',  ( 30.91344420362545975, -3.401318489841207882, 1.000000000000000000 ) ) ;
#11931=DIRECTION ( 'NONE',  ( 0.6845471059286901694, -0.7289686274214101092, 0.000000000000000000 ) ) ;
#11932=AXIS2_PLACEMENT_3D ( 'NONE', #9539, #7971, #11889 ) ;
#11933=ORIENTED_EDGE ( 'NONE', *, *, #19445, .T. ) ;
#11934=VERTEX_POINT ( 'NONE', #24544 ) ;
#11936=ORIENTED_EDGE ( 'NONE', *, *, #15233, .T. ) ;
#11940=CARTESIAN_POINT ( 'NONE',  ( -17.87326343783962201, -25.45105997952905597, -6.500000000000000000 ) ) ;
#11942=CARTESIAN_POINT ( 'NONE',  ( -16.66421332384701515, -26.25859848311253941, 1.000000000000000000 ) ) ;
#11945=EDGE_CURVE ( 'NONE', #20109, #5929, #15950, .T. ) ;
#11951=EDGE_CURVE ( 'NONE', #22201, #18149, #4661, .T. ) ;
#11953=CARTESIAN_POINT ( 'NONE',  ( 28.91604871112457076, -11.44867358849361416, -6.500000000000000000 ) ) ;
#11954=EDGE_CURVE ( 'NONE', #16234, #962, #8010, .T. ) ;
#11963=ORIENTED_EDGE ( 'NONE', *, *, #9500, .T. ) ;
#11969=DIRECTION ( 'NONE',  ( 0.9921147013144777649, -0.1253332335643050077, 0.000000000000000000 ) ) ;
#11970=CARTESIAN_POINT ( 'NONE',  ( 19.82388608118429119, 23.96296185032701587, -6.500000000000000000 ) ) ;
#11972=ORIENTED_EDGE ( 'NONE', *, *, #19132, .T. ) ;
#11973=ORIENTED_EDGE ( 'NONE', *, *, #4394, .T. ) ;
#11978=LINE ( 'NONE', #9776, #10837 ) ;
#11982=CARTESIAN_POINT ( 'NONE',  ( 14.54246377227358877, 27.49048467073853175, 1.000000000000000000 ) ) ;
#11984=DIRECTION ( 'NONE',  ( 0.000000000000000000, 0.000000000000000000, -1.000000000000000000 ) ) ;
#11988=CARTESIAN_POINT ( 'NONE',  ( -18.28012134629613783, -25.16042852506070560, -6.500000000000000000 ) ) ;
#11997=CARTESIAN_POINT ( 'NONE',  ( -23.64116323484209659, 20.20656826142307239, -6.500000000000000000 ) ) ;
#11998=DIRECTION ( 'NONE',  ( 0.2486898871648653975, 0.9685831611286285225, 0.000000000000000000 ) ) ;
#12002=ORIENTED_EDGE ( 'NONE', *, *, #7581, .T. ) ;
#12003=DIRECTION ( 'NONE',  ( 1.000000000000000000, 0.000000000000000000, 0.000000000000000000 ) ) ;
#12004=CARTESIAN_POINT ( 'NONE',  ( 0.000000000000000000, 0.000000000000000000, 0.000000000000000000 ) ) ;
#12005=VECTOR ( 'NONE', #14091, 1000.000000000000000 ) ;
#12007=EDGE_CURVE ( 'NONE', #2048, #14460, #10925, .T. ) ;
#12009=DIRECTION ( 'NONE',  ( 0.000000000000000000, 0.000000000000000000, 1.000000000000000000 ) ) ;
#12012=ADVANCED_FACE ( 'NONE', ( #25326 ), #23234, .F. ) ;
#12014=DIRECTION ( 'NONE',  ( 0.000000000000000000, 0.000000000000000000, 1.000000000000000000 ) ) ;
#12017=CYLINDRICAL_SURFACE ( 'NONE', #11189, 0.4999999999999970024 ) ;
#12022=DIRECTION ( 'NONE',  ( -0.000000000000000000, -0.000000000000000000, 1.000000000000000000 ) ) ;
#12023=CIRCLE ( 'NONE', #22049, 31.10000000000000142 ) ;
#12026=ORIENTED_EDGE ( 'NONE', *, *, #15336, .F. ) ;
#12028=LINE ( 'NONE', #2245, #7509 ) ;
#12029=DIRECTION ( 'NONE',  ( -0.5358267949790012086, -0.8443279255020122998, 0.000000000000000000 ) ) ;
#12030=EDGE_LOOP ( 'NONE', ( #18562, #7225, #18882, #16010 ) ) ;
#12031=ORIENTED_EDGE ( 'NONE', *, *, #14100, .T. ) ;
#12033=CIRCLE ( 'NONE', #18297, 0.5000000000000001110 ) ;
#12034=ORIENTED_EDGE ( 'NONE', *, *, #25399, .F. ) ;
#12037=DIRECTION ( 'NONE',  ( 0.000000000000000000, 0.000000000000000000, 1.000000000000000000 ) ) ;
#12043=DIRECTION ( 'NONE',  ( -0.000000000000000000, -0.000000000000000000, 1.000000000000000000 ) ) ;
#12044=AXIS2_PLACEMENT_3D ( 'NONE', #19925, #81, #17731 ) ;
#12047=DIRECTION ( 'NONE',  ( 0.1873813145857330109, 0.9822872507286871668, 0.000000000000000000 ) ) ;
#12058=ORIENTED_EDGE ( 'NONE', *, *, #18638, .T. ) ;
#12061=CIRCLE ( 'NONE', #2888, 0.5000000000000001110 ) ;
#12062=ORIENTED_EDGE ( 'NONE', *, *, #21128, .F. ) ;
#12065=CIRCLE ( 'NONE', #17861, 0.5000000000000004441 ) ;
#12066=DIRECTION ( 'NONE',  ( 0.000000000000000000, 0.000000000000000000, 1.000000000000000000 ) ) ;
#12068=ORIENTED_EDGE ( 'NONE', *, *, #8779, .T. ) ;
#12070=CIRCLE ( 'NONE', #7060, 0.5000000000000003331 ) ;
#12071=EDGE_CURVE ( 'NONE', #17619, #8646, #20973, .T. ) ;
#12072=CARTESIAN_POINT ( 'NONE',  ( 8.217531866531214035, 29.99470236596028982, -6.500000000000000000 ) ) ;
#12073=CIRCLE ( 'NONE', #13744, 31.10000000000000142 ) ;
#12075=DIRECTION ( 'NONE',  ( 0.000000000000000000, 0.000000000000000000, 1.000000000000000000 ) ) ;
#12077=CARTESIAN_POINT ( 'NONE',  ( -11.44867358849309547, 28.91604871112477326, -6.500000000000000000 ) ) ;
#12082=CIRCLE ( 'NONE', #12932, 31.10000000000000142 ) ;
#12083=AXIS2_PLACEMENT_3D ( 'NONE', #14917, #21181, #9414 ) ;
#12085=AXIS2_PLACEMENT_3D ( 'NONE', #19506, #25670, #11277 ) ;
#12089=DIRECTION ( 'NONE',  ( 1.000000000000000000, 0.000000000000000000, 0.000000000000000000 ) ) ;
#12090=DIRECTION ( 'NONE',  ( 1.000000000000000000, 0.000000000000000000, 0.000000000000000000 ) ) ;
#12091=LINE ( 'NONE', #20066, #2570 ) ;
#12093=LINE ( 'NONE', #24002, #6637 ) ;
#12096=AXIS2_PLACEMENT_3D ( 'NONE', #25269, #19244, #11402 ) ;
#12101=VERTEX_POINT ( 'NONE', #19794 ) ;
#12103=VECTOR ( 'NONE', #17797, 1000.000000000000000 ) ;
#12104=LINE ( 'NONE', #4125, #878 ) ;
#12107=ORIENTED_EDGE ( 'NONE', *, *, #6708, .T. ) ;
#12112=EDGE_CURVE ( 'NONE', #6766, #25247, #7594, .T. ) ;
#12117=DIRECTION ( 'NONE',  ( 1.000000000000000000, 0.000000000000000000, 0.000000000000000000 ) ) ;
#12121=DIRECTION ( 'NONE',  ( 0.000000000000000000, 0.000000000000000000, 1.000000000000000000 ) ) ;
#12122=DIRECTION ( 'NONE',  ( 1.000000000000000000, 0.000000000000000000, 0.000000000000000000 ) ) ;
#12129=DIRECTION ( 'NONE',  ( 0.000000000000000000, 0.000000000000000000, 1.000000000000000000 ) ) ;
#12132=EDGE_LOOP ( 'NONE', ( #16328, #9740, #7195, #21382 ) ) ;
#12138=AXIS2_PLACEMENT_3D ( 'NONE', #24889, #23181, #14827 ) ;
#12143=ORIENTED_EDGE ( 'NONE', *, *, #16545, .F. ) ;
#12144=DIRECTION ( 'NONE',  ( -0.7289686274214168815, -0.6845471059286831750, 0.000000000000000000 ) ) ;
#12145=AXIS2_PLACEMENT_3D ( 'NONE', #15555, #23524, #5608 ) ;
#12147=CIRCLE ( 'NONE', #15075, 0.5000000000000001110 ) ;
#12150=AXIS2_PLACEMENT_3D ( 'NONE', #268, #22230, #5887 ) ;
#12155=CARTESIAN_POINT ( 'NONE',  ( -1.952785157361201618, 31.03863125411927371, -6.500000000000000000 ) ) ;
#12156=CIRCLE ( 'NONE', #2983, 31.10000000000000142 ) ;
#12161=AXIS2_PLACEMENT_3D ( 'NONE', #7019, #15005, #22986 ) ;
#12166=ORIENTED_EDGE ( 'NONE', *, *, #24563, .T. ) ;
#12169=VERTEX_POINT ( 'NONE', #15316 ) ;
#12173=VERTEX_POINT ( 'NONE', #5505 ) ;
#12174=ORIENTED_EDGE ( 'NONE', *, *, #5637, .F. ) ;
#12175=ORIENTED_EDGE ( 'NONE', *, *, #6227, .T. ) ;
#12184=VECTOR ( 'NONE', #21201, 1000.000000000000000 ) ;
#12190=LINE ( 'NONE', #8265, #6306 ) ;
#12191=FACE_OUTER_BOUND ( 'NONE', #11270, .T. ) ;
#12196=DIRECTION ( 'NONE',  ( 0.000000000000000000, 0.000000000000000000, 1.000000000000000000 ) ) ;
#12199=AXIS2_PLACEMENT_3D ( 'NONE', #19092, #23275, #7585 ) ;
#12201=EDGE_LOOP ( 'NONE', ( #24577, #25717, #23879, #15210 ) ) ;
#12206=CARTESIAN_POINT ( 'NONE',  ( -30.54913349766215802, 5.827558883616378083, -6.500000000000000000 ) ) ;
#12210=VECTOR ( 'NONE', #24421, 1000.000000000000000 ) ;
#12211=EDGE_CURVE ( 'NONE', #8412, #24490, #19364, .T. ) ;
#12216=CARTESIAN_POINT ( 'NONE',  ( 0.000000000000000000, 0.000000000000000000, -6.500000000000000000 ) ) ;
#12217=AXIS2_PLACEMENT_3D ( 'NONE', #23373, #17371, #13188 ) ;
#12219=DIRECTION ( 'NONE',  ( 1.000000000000000000, 0.000000000000000000, 0.000000000000000000 ) ) ;
#12224=DIRECTION ( 'NONE',  ( 1.000000000000000000, 0.000000000000000000, 0.000000000000000000 ) ) ;
#12225=AXIS2_PLACEMENT_3D ( 'NONE', #14954, #9196, #4884 ) ;
#12227=DIRECTION ( 'NONE',  ( -0.000000000000000000, -0.000000000000000000, 1.000000000000000000 ) ) ;
#12232=ORIENTED_EDGE ( 'NONE', *, *, #1567, .F. ) ;
#12234=CARTESIAN_POINT ( 'NONE',  ( -9.110428525060477511, 29.57785765677940404, -6.500000000000000000 ) ) ;
#12237=VERTEX_POINT ( 'NONE', #13613 ) ;
#12241=ORIENTED_EDGE ( 'NONE', *, *, #21784, .F. ) ;
#12242=ORIENTED_EDGE ( 'NONE', *, *, #2578, .T. ) ;
#12246=EDGE_CURVE ( 'NONE', #16230, #24819, #11513, .T. ) ;
#12248=VECTOR ( 'NONE', #19687, 1000.000000000000000 ) ;
#12250=AXIS2_PLACEMENT_3D ( 'NONE', #6366, #4659, #16567 ) ;
#12253=DIRECTION ( 'NONE',  ( 0.000000000000000000, 0.000000000000000000, 1.000000000000000000 ) ) ;
#12254=CARTESIAN_POINT ( 'NONE',  ( 3.401318489841097747, 30.91344420362547396, 1.000000000000000000 ) ) ;
#12255=CARTESIAN_POINT ( 'NONE',  ( 30.24338421796779386, -7.248980000274303670, -2.750000000000000000 ) ) ;
#12260=ORIENTED_EDGE ( 'NONE', *, *, #17375, .T. ) ;
#12263=FACE_OUTER_BOUND ( 'NONE', #5769, .T. ) ;
#12264=VERTEX_POINT ( 'NONE', #5633 ) ;
#12272=FACE_OUTER_BOUND ( 'NONE', #5620, .T. ) ;
#12274=AXIS2_PLACEMENT_3D ( 'NONE', #9479, #17457, #15368 ) ;
#12275=VERTEX_POINT ( 'NONE', #1577 ) ;
#12279=CYLINDRICAL_SURFACE ( 'NONE', #3024, 31.10000000000000142 ) ;
#12282=CARTESIAN_POINT ( 'NONE',  ( 4.393401135980900207, -30.78811501957146390, 1.000000000000000000 ) ) ;
#12283=ADVANCED_FACE ( 'NONE', ( #15583 ), #21579, .F. ) ;
#12285=DIRECTION ( 'NONE',  ( 1.387778780781445044E-14, 1.000000000000000000, 0.000000000000000000 ) ) ;
#12288=EDGE_CURVE ( 'NONE', #13585, #14795, #15129, .T. ) ;
#12292=CARTESIAN_POINT ( 'NONE',  ( -0.4999838450258491940, -31.09598070739550124, 1.000000000000000000 ) ) ;
#12295=DIRECTION ( 'NONE',  ( 0.000000000000000000, 0.000000000000000000, -1.000000000000000000 ) ) ;
#12303=ORIENTED_EDGE ( 'NONE', *, *, #11945, .T. ) ;
#12304=ORIENTED_EDGE ( 'NONE', *, *, #9853, .T. ) ;
#12305=FACE_OUTER_BOUND ( 'NONE', #23058, .T. ) ;
#12306=ORIENTED_EDGE ( 'NONE', *, *, #24265, .F. ) ;
#12308=VERTEX_POINT ( 'NONE', #3795 ) ;
#12311=VERTEX_POINT ( 'NONE', #20131 ) ;
#12315=DIRECTION ( 'NONE',  ( 0.000000000000000000, 0.000000000000000000, 1.000000000000000000 ) ) ;
#12317=DIRECTION ( 'NONE',  ( 1.000000000000000000, 0.000000000000000000, 0.000000000000000000 ) ) ;
#12319=DIRECTION ( 'NONE',  ( 0.000000000000000000, 0.000000000000000000, 1.000000000000000000 ) ) ;
#12322=CARTESIAN_POINT ( 'NONE',  ( -5.335677986745010593, -30.63887302793242284, -6.500000000000000000 ) ) ;
#12325=EDGE_CURVE ( 'NONE', #16191, #10388, #24305, .T. ) ;
#12326=CARTESIAN_POINT ( 'NONE',  ( 0.000000000000000000, 0.000000000000000000, 1.000000000000000000 ) ) ;
#12327=CARTESIAN_POINT ( 'NONE',  ( 7.734255490827002255, 30.12293631110042469, -6.500000000000000000 ) ) ;
#12328=ADVANCED_FACE ( 'NONE', ( #19753 ), #13872, .F. ) ;
#12332=ORIENTED_EDGE ( 'NONE', *, *, #22807, .T. ) ;
#12333=CYLINDRICAL_SURFACE ( 'NONE', #1609, 0.5000000000000004441 ) ;
#12334=EDGE_LOOP ( 'NONE', ( #24043, #2724, #3557, #21115 ) ) ;
#12337=ORIENTED_EDGE ( 'NONE', *, *, #25360, .F. ) ;
#12338=CIRCLE ( 'NONE', #12754, 31.10000000000000142 ) ;
#12339=DIRECTION ( 'NONE',  ( 1.000000000000000000, 0.000000000000000000, 0.000000000000000000 ) ) ;
#12340=VERTEX_POINT ( 'NONE', #18064 ) ;
#12341=AXIS2_PLACEMENT_3D ( 'NONE', #24473, #18469, #10603 ) ;
#12344=DIRECTION ( 'NONE',  ( 0.000000000000000000, 0.000000000000000000, 1.000000000000000000 ) ) ;
#12345=CARTESIAN_POINT ( 'NONE',  ( 7.248980000273979485, -30.24338421796786847, -6.500000000000000000 ) ) ;
#12346=DIRECTION ( 'NONE',  ( 0.000000000000000000, 0.000000000000000000, 1.000000000000000000 ) ) ;
#12348=CYLINDRICAL_SURFACE ( 'NONE', #22694, 0.5000000000000004441 ) ;
#12349=AXIS2_PLACEMENT_3D ( 'NONE', #9223, #11438, #7645 ) ;
#12353=ADVANCED_FACE ( 'NONE', ( #24324 ), #3929, .F. ) ;
#12357=CARTESIAN_POINT ( 'NONE',  ( -30.60000000000000142, 3.257552089140643357E-13, 1.000000000000000000 ) ) ;
#12366=EDGE_CURVE ( 'NONE', #4853, #89, #5501, .T. ) ;
#12369=ORIENTED_EDGE ( 'NONE', *, *, #8373, .F. ) ;
#12370=ORIENTED_EDGE ( 'NONE', *, *, #4735, .T. ) ;
#12373=DIRECTION ( 'NONE',  ( 1.000000000000000000, 0.000000000000000000, 0.000000000000000000 ) ) ;
#12375=DIRECTION ( 'NONE',  ( 0.8090169943749532244, 0.5877852522924652545, 0.000000000000000000 ) ) ;
#12377=CARTESIAN_POINT ( 'NONE',  ( 12.78762572734057024, 28.34936733434201273, 1.000000000000000000 ) ) ;
#12378=DIRECTION ( 'NONE',  ( -0.4817536741017198754, -0.8763066800438610304, 0.000000000000000000 ) ) ;
#12379=DIRECTION ( 'NONE',  ( 1.000000000000000000, 0.000000000000000000, 0.000000000000000000 ) ) ;
#12383=CARTESIAN_POINT ( 'NONE',  ( -29.07785765677917311, 9.610428525061202265, 1.000000000000000000 ) ) ;
#12390=ORIENTED_EDGE ( 'NONE', *, *, #3063, .F. ) ;
#12391=CARTESIAN_POINT ( 'NONE',  ( -22.32573188046936252, -21.65113613650319380, 1.000000000000000000 ) ) ;
#12397=EDGE_CURVE ( 'NONE', #1315, #7103, #19291, .T. ) ;
#12402=ADVANCED_FACE ( 'NONE', ( #14394 ), #22231, .T. ) ;
#12409=CARTESIAN_POINT ( 'NONE',  ( -17.78012134629558716, 25.16042852506110705, 1.000000000000000000 ) ) ;
#12411=CARTESIAN_POINT ( 'NONE',  ( -10.08469938919458286, 29.41953157733104263, 1.000000000000000000 ) ) ;
#12417=DIRECTION ( 'NONE',  ( 1.000000000000000000, 0.000000000000000000, 0.000000000000000000 ) ) ;
#12420=CARTESIAN_POINT ( 'NONE',  ( -5.327558883615603591, 30.54913349766230724, -6.500000000000000000 ) ) ;
#12421=CYLINDRICAL_SURFACE ( 'NONE', #19584, 31.10000000000000142 ) ;
#12424=EDGE_CURVE ( 'NONE', #15870, #6150, #146, .T. ) ;
#12425=ORIENTED_EDGE ( 'NONE', *, *, #642, .F. ) ;
#12429=ORIENTED_EDGE ( 'NONE', *, *, #9891, .T. ) ;
#12440=DIRECTION ( 'NONE',  ( 1.000000000000000000, 0.000000000000000000, 0.000000000000000000 ) ) ;
#12441=CIRCLE ( 'NONE', #25810, 0.5000000000000007772 ) ;
#12448=CIRCLE ( 'NONE', #3676, 31.10000000000000142 ) ;
#12453=DIRECTION ( 'NONE',  ( 0.000000000000000000, 0.000000000000000000, 1.000000000000000000 ) ) ;
#12456=ORIENTED_EDGE ( 'NONE', *, *, #4246, .T. ) ;
#12458=CARTESIAN_POINT ( 'NONE',  ( -12.74173596767398742, -28.14012133169310559, 1.000000000000000000 ) ) ;
#12459=ORIENTED_EDGE ( 'NONE', *, *, #7442, .F. ) ;
#12461=AXIS2_PLACEMENT_3D ( 'NONE', #18028, #23905, #2442 ) ;
#12467=CARTESIAN_POINT ( 'NONE',  ( -14.48253926456298579, 27.25313774936435962, -6.500000000000000000 ) ) ;
#12471=AXIS2_PLACEMENT_3D ( 'NONE', #16707, #4809, #12784 ) ;
#12472=CIRCLE ( 'NONE', #12858, 31.10000000000000142 ) ;
#12476=AXIS2_PLACEMENT_3D ( 'NONE', #5291, #1380, #22954 ) ;
#12479=AXIS2_PLACEMENT_3D ( 'NONE', #3908, #7821, #16073 ) ;
#12482=EDGE_CURVE ( 'NONE', #18610, #19636, #11770, .T. ) ;
#12485=VERTEX_POINT ( 'NONE', #20518 ) ;
#12490=EDGE_LOOP ( 'NONE', ( #25, #24209, #6665, #17244 ) ) ;
#12491=VERTEX_POINT ( 'NONE', #4950 ) ;
#12494=LINE ( 'NONE', #2314, #8037 ) ;
#12495=EDGE_CURVE ( 'NONE', #20454, #3228, #2613, .T. ) ;
#12498=EDGE_CURVE ( 'NONE', #23985, #3679, #20550, .T. ) ;
#12499=AXIS2_PLACEMENT_3D ( 'NONE', #2538, #22157, #14327 ) ;
#12506=DIRECTION ( 'NONE',  ( 0.000000000000000000, 0.000000000000000000, 1.000000000000000000 ) ) ;
#12508=CARTESIAN_POINT ( 'NONE',  ( 29.72853858738285737, 9.133673601486366422, -6.500000000000000000 ) ) ;
#12512=CARTESIAN_POINT ( 'NONE',  ( 18.68225429291714690, -24.86329371854781201, -2.750000000000000000 ) ) ;
#12516=CIRCLE ( 'NONE', #3742, 0.5000000000000017764 ) ;
#12517=DIRECTION ( 'NONE',  ( 1.000000000000000000, 0.000000000000000000, 0.000000000000000000 ) ) ;
#12524=VERTEX_POINT ( 'NONE', #24561 ) ;
#12526=CIRCLE ( 'NONE', #13379, 0.5000000000000003331 ) ;
#12532=DIRECTION ( 'NONE',  ( 0.000000000000000000, -0.000000000000000000, 1.000000000000000000 ) ) ;
#12533=CARTESIAN_POINT ( 'NONE',  ( 25.45105997952925136, 17.87326343783933780, -6.500000000000000000 ) ) ;
#12534=CIRCLE ( 'NONE', #15883, 0.5000000000000001110 ) ;
#12537=CIRCLE ( 'NONE', #17980, 31.10000000000000142 ) ;
#12540=ADVANCED_FACE ( 'NONE', ( #22620 ), #18683, .T. ) ;
#12543=EDGE_CURVE ( 'NONE', #9673, #6572, #771, .T. ) ;
#12547=DIRECTION ( 'NONE',  ( 0.000000000000000000, 0.000000000000000000, 1.000000000000000000 ) ) ;
#12550=LINE ( 'NONE', #14272, #25700 ) ;
#12551=CARTESIAN_POINT ( 'NONE',  ( -12.74173596767339767, 28.14012133169338270, -6.500000000000000000 ) ) ;
#12552=DIRECTION ( 'NONE',  ( -0.8090169943749417891, 0.5877852522924807976, 0.000000000000000000 ) ) ;
#12557=ORIENTED_EDGE ( 'NONE', *, *, #10251, .F. ) ;
#12558=VECTOR ( 'NONE', #915, 1000.000000000000000 ) ;
#12559=AXIS2_PLACEMENT_3D ( 'NONE', #4464, #20407, #12317 ) ;
#12560=ORIENTED_EDGE ( 'NONE', *, *, #24953, .T. ) ;
#12562=ORIENTED_EDGE ( 'NONE', *, *, #7392, .F. ) ;
#12567=AXIS2_PLACEMENT_3D ( 'NONE', #24056, #17914, #11897 ) ;
#12577=EDGE_CURVE ( 'NONE', #17170, #12491, #2600, .T. ) ;
#12581=CARTESIAN_POINT ( 'NONE',  ( -13.24173596767339767, 28.14012133169338270, 1.000000000000000000 ) ) ;
#12583=DIRECTION ( 'NONE',  ( 0.000000000000000000, 0.000000000000000000, 1.000000000000000000 ) ) ;
#12586=AXIS2_PLACEMENT_3D ( 'NONE', #16572, #2577, #6615 ) ;
#12588=CARTESIAN_POINT ( 'NONE',  ( -6.317933499822993682, 30.45149776762736593, -2.750000000000000000 ) ) ;
#12589=EDGE_LOOP ( 'NONE', ( #5738, #9034, #4329, #17073 ) ) ;
#12590=ORIENTED_EDGE ( 'NONE', *, *, #7980, .F. ) ;
#12596=DIRECTION ( 'NONE',  ( 0.000000000000000000, 0.000000000000000000, 1.000000000000000000 ) ) ;
#12597=ORIENTED_EDGE ( 'NONE', *, *, #24350, .F. ) ;
#12603=DIRECTION ( 'NONE',  ( -0.5877852522924652545, 0.8090169943749532244, 0.000000000000000000 ) ) ;
#12605=CARTESIAN_POINT ( 'NONE',  ( -1.952785157361865753, -31.03863125411923463, -6.500000000000000000 ) ) ;
#12608=CIRCLE ( 'NONE', #6756, 31.10000000000000142 ) ;
#12614=AXIS2_PLACEMENT_3D ( 'NONE', #15025, #13069, #16991 ) ;
#12616=AXIS2_PLACEMENT_3D ( 'NONE', #21171, #11099, #16743 ) ;
#12620=CIRCLE ( 'NONE', #11367, 0.5000000000000005551 ) ;
#12622=LINE ( 'NONE', #20595, #22107 ) ;
#12627=ORIENTED_EDGE ( 'NONE', *, *, #18886, .T. ) ;
#12630=DIRECTION ( 'NONE',  ( 1.000000000000000000, 0.000000000000000000, 0.000000000000000000 ) ) ;
#12634=AXIS2_PLACEMENT_3D ( 'NONE', #9420, #15572, #21452 ) ;
#12635=DIRECTION ( 'NONE',  ( 1.000000000000000000, 0.000000000000000000, 0.000000000000000000 ) ) ;
#12645=CARTESIAN_POINT ( 'NONE',  ( -7.734255490826573265, 30.12293631110053838, -6.500000000000000000 ) ) ;
#12647=AXIS2_PLACEMENT_3D ( 'NONE', #13063, #23128, #20901 ) ;
#12649=CYLINDRICAL_SURFACE ( 'NONE', #7991, 31.10000000000000142 ) ;
#12654=CARTESIAN_POINT ( 'NONE',  ( 25.16042852506077665, -18.28012134629603835, -6.500000000000000000 ) ) ;
#12656=AXIS2_PLACEMENT_3D ( 'NONE', #7957, #19466, #24036 ) ;
#12669=DIRECTION ( 'NONE',  ( 0.000000000000000000, 0.000000000000000000, 1.000000000000000000 ) ) ;
#12670=AXIS2_PLACEMENT_3D ( 'NONE', #16420, #22412, #18508 ) ;
#12671=ORIENTED_EDGE ( 'NONE', *, *, #24526, .T. ) ;
#12673=VERTEX_POINT ( 'NONE', #1674 ) ;
#12675=ORIENTED_EDGE ( 'NONE', *, *, #23124, .F. ) ;
#12681=ADVANCED_FACE ( 'NONE', ( #15407 ), #15282, .F. ) ;
#12684=DIRECTION ( 'NONE',  ( 0.000000000000000000, 0.000000000000000000, 1.000000000000000000 ) ) ;
#12688=DIRECTION ( 'NONE',  ( -0.9510565162951518658, 0.3090169943749528914, 0.000000000000000000 ) ) ;
#12692=CARTESIAN_POINT ( 'NONE',  ( -25.75859848311247902, 16.66421332384710752, 1.000000000000000000 ) ) ;
#12693=CIRCLE ( 'NONE', #9749, 31.10000000000000142 ) ;
#12699=VERTEX_POINT ( 'NONE', #13696 ) ;
#12702=VERTEX_POINT ( 'NONE', #15545 ) ;
#12704=EDGE_CURVE ( 'NONE', #14144, #22219, #20127, .T. ) ;
#12707=ADVANCED_FACE ( 'NONE', ( #7557 ), #3507, .F. ) ;
#12719=CARTESIAN_POINT ( 'NONE',  ( -30.85476721088022600, 3.897863563850190616, -6.500000000000000000 ) ) ;
#12721=CARTESIAN_POINT ( 'NONE',  ( 0.000000000000000000, 0.000000000000000000, -6.500000000000000000 ) ) ;
#12722=DIRECTION ( 'NONE',  ( -0.5358267949789882190, 0.8443279255020205154, 0.000000000000000000 ) ) ;
#12725=CARTESIAN_POINT ( 'NONE',  ( -25.16042852506064165, 18.28012134629622309, 1.000000000000000000 ) ) ;
#12729=EDGE_LOOP ( 'NONE', ( #16531, #14501, #8941, #22859 ) ) ;
#12733=EDGE_CURVE ( 'NONE', #20576, #24829, #14313, .T. ) ;
#12737=VERTEX_POINT ( 'NONE', #25092 ) ;
#12738=CARTESIAN_POINT ( 'NONE',  ( -31.06601413805604039, -1.453535542772269595, -6.500000000000000000 ) ) ;
#12740=EDGE_CURVE ( 'NONE', #17935, #12275, #5123, .T. ) ;
#12741=CARTESIAN_POINT ( 'NONE',  ( -28.34936733434187062, 12.78762572734086866, 1.000000000000000000 ) ) ;
#12748=FACE_OUTER_BOUND ( 'NONE', #23661, .T. ) ;
#12749=ORIENTED_EDGE ( 'NONE', *, *, #4067, .T. ) ;
#12751=CARTESIAN_POINT ( 'NONE',  ( -23.96296185032722548, -19.82388608118403539, 1.000000000000000000 ) ) ;
#12754=AXIS2_PLACEMENT_3D ( 'NONE', #24715, #10196, #276 ) ;
#12759=ORIENTED_EDGE ( 'NONE', *, *, #2922, .T. ) ;
#12762=DIRECTION ( 'NONE',  ( 0.000000000000000000, 0.000000000000000000, 1.000000000000000000 ) ) ;
#12769=CIRCLE ( 'NONE', #678, 0.5000000000000009992 ) ;
#12770=CARTESIAN_POINT ( 'NONE',  ( 0.000000000000000000, 0.000000000000000000, -6.500000000000000000 ) ) ;
#12775=VECTOR ( 'NONE', #18286, 1000.000000000000000 ) ;
#12776=CARTESIAN_POINT ( 'NONE',  ( -16.66421332384701515, -26.25859848311253941, -6.500000000000000000 ) ) ;
#12778=CARTESIAN_POINT ( 'NONE',  ( -15.41874213889376044, 27.00874656207322388, -2.750000000000000000 ) ) ;
#12781=CARTESIAN_POINT ( 'NONE',  ( -23.64116323484252291, -20.20656826142258211, -2.750000000000000000 ) ) ;
#12782=DIRECTION ( 'NONE',  ( 0.000000000000000000, 0.000000000000000000, 1.000000000000000000 ) ) ;
#12784=DIRECTION ( 'NONE',  ( 1.000000000000000000, 0.000000000000000000, 0.000000000000000000 ) ) ;
#12787=AXIS2_PLACEMENT_3D ( 'NONE', #7587, #10053, #1841 ) ;
#12792=ORIENTED_EDGE ( 'NONE', *, *, #5762, .F. ) ;
#12798=( LENGTH_UNIT ( ) NAMED_UNIT ( * ) SI_UNIT ( .MILLI., .METRE. ) );
#12805=CARTESIAN_POINT ( 'NONE',  ( 30.78811501957143548, -4.393401135981102712, 1.000000000000000000 ) ) ;
#12809=CARTESIAN_POINT ( 'NONE',  ( -4.393401135980685268, 30.78811501957149588, 1.000000000000000000 ) ) ;
#12815=CARTESIAN_POINT ( 'NONE',  ( 20.92219106202050583, 23.01025686871638598, -6.500000000000000000 ) ) ;
#12816=DIRECTION ( 'NONE',  ( 0.000000000000000000, 0.000000000000000000, 1.000000000000000000 ) ) ;
#12818=VERTEX_POINT ( 'NONE', #3894 ) ;
#12819=CARTESIAN_POINT ( 'NONE',  ( -30.54913349766228592, -5.827558883615738594, -6.500000000000000000 ) ) ;
#12820=CARTESIAN_POINT ( 'NONE',  ( 16.66421332384664566, -26.25859848311276679, -6.500000000000000000 ) ) ;
#12822=EDGE_LOOP ( 'NONE', ( #12824, #12869, #6538, #25630 ) ) ;
#12824=ORIENTED_EDGE ( 'NONE', *, *, #2700, .F. ) ;
#12828=ORIENTED_EDGE ( 'NONE', *, *, #1570, .F. ) ;
#12831=EDGE_CURVE ( 'NONE', #25296, #12101, #16176, .T. ) ;
#12838=CARTESIAN_POINT ( 'NONE',  ( -26.25859848311282363, -16.66421332384654974, 1.000000000000000000 ) ) ;
#12839=DIRECTION ( 'NONE',  ( 0.8090169943749532244, 0.5877852522924652545, 0.000000000000000000 ) ) ;
#12840=EDGE_CURVE ( 'NONE', #19322, #3259, #13055, .T. ) ;
#12841=CARTESIAN_POINT ( 'NONE',  ( -12.78762572734076919, -28.34936733434192035, 1.000000000000000000 ) ) ;
#12844=CARTESIAN_POINT ( 'NONE',  ( 31.03863125411925239, 1.952785157361540236, 1.000000000000000000 ) ) ;
#12845=CARTESIAN_POINT ( 'NONE',  ( -29.62293631110050995, -7.734255490826679846, -6.500000000000000000 ) ) ;
#12846=ORIENTED_EDGE ( 'NONE', *, *, #6052, .F. ) ;
#12853=ORIENTED_EDGE ( 'NONE', *, *, #24055, .T. ) ;
#12855=VERTEX_POINT ( 'NONE', #19953 ) ;
#12858=AXIS2_PLACEMENT_3D ( 'NONE', #13007, #3311, #7250 ) ;
#12864=EDGE_CURVE ( 'NONE', #19636, #18810, #16313, .T. ) ;
#12866=EDGE_CURVE ( 'NONE', #7097, #13890, #419, .T. ) ;
#12868=CARTESIAN_POINT ( 'NONE',  ( 29.41953157733091118, -10.08469938919497721, 1.000000000000000000 ) ) ;
#12869=ORIENTED_EDGE ( 'NONE', *, *, #19981, .T. ) ;
#12870=CARTESIAN_POINT ( 'NONE',  ( -23.01025686871616216, 20.92219106202074741, 1.000000000000000000 ) ) ;
#12874=AXIS2_PLACEMENT_3D ( 'NONE', #13234, #19371, #18993 ) ;
#12875=DIRECTION ( 'NONE',  ( -0.000000000000000000, -0.000000000000000000, 1.000000000000000000 ) ) ;
#12882=CARTESIAN_POINT ( 'NONE',  ( 0.000000000000000000, 0.000000000000000000, -6.500000000000000000 ) ) ;
#12883=VECTOR ( 'NONE', #24117, 1000.000000000000000 ) ;
#12886=DIRECTION ( 'NONE',  ( 0.000000000000000000, 0.000000000000000000, 1.000000000000000000 ) ) ;
#12888=CARTESIAN_POINT ( 'NONE',  ( -19.82388608118395013, 23.96296185032730364, -6.500000000000000000 ) ) ;
#12891=DIRECTION ( 'NONE',  ( 0.000000000000000000, 0.000000000000000000, 1.000000000000000000 ) ) ;
#12893=EDGE_CURVE ( 'NONE', #23600, #21660, #23365, .T. ) ;
#12899=ADVANCED_FACE ( 'NONE', ( #22053 ), #10156, .F. ) ;
#12900=CARTESIAN_POINT ( 'NONE',  ( 19.82388608118411710, -23.96296185032715798, -6.500000000000000000 ) ) ;
#12902=AXIS2_PLACEMENT_3D ( 'NONE', #24962, #3379, #25477 ) ;
#12906=LINE ( 'NONE', #8716, #23483 ) ;
#12911=DIRECTION ( 'NONE',  ( -0.5358267949789882190, 0.8443279255020205154, 0.000000000000000000 ) ) ;
#12912=ORIENTED_EDGE ( 'NONE', *, *, #13425, .T. ) ;
#12916=FACE_OUTER_BOUND ( 'NONE', #11534, .T. ) ;
#12918=DIRECTION ( 'NONE',  ( 0.000000000000000000, 0.000000000000000000, -1.000000000000000000 ) ) ;
#12919=EDGE_CURVE ( 'NONE', #4816, #24761, #14221, .T. ) ;
#12920=AXIS2_PLACEMENT_3D ( 'NONE', #17093, #18663, #21024 ) ;
#12921=VERTEX_POINT ( 'NONE', #12377 ) ;
#12923=ORIENTED_EDGE ( 'NONE', *, *, #2367, .F. ) ;
#12928=AXIS2_PLACEMENT_3D ( 'NONE', #9142, #25104, #7193 ) ;
#12931=CARTESIAN_POINT ( 'NONE',  ( -30.10000000000000142, 3.686186865433532535E-15, -6.500000000000000000 ) ) ;
#12932=AXIS2_PLACEMENT_3D ( 'NONE', #25196, #3338, #3596 ) ;
#12934=CARTESIAN_POINT ( 'NONE',  ( -27.92360179968386547, -13.69242354489123770, -2.750000000000000000 ) ) ;
#12935=CIRCLE ( 'NONE', #821, 31.10000000000000142 ) ;
#12940=DIRECTION ( 'NONE',  ( 0.000000000000000000, 0.000000000000000000, 1.000000000000000000 ) ) ;
#12941=CYLINDRICAL_SURFACE ( 'NONE', #16374, 0.5000000000000004441 ) ;
#12944=AXIS2_PLACEMENT_3D ( 'NONE', #18267, #22319, #12375 ) ;
#12945=ADVANCED_FACE ( 'NONE', ( #16696 ), #20874, .F. ) ;
#12947=AXIS2_PLACEMENT_3D ( 'NONE', #16291, #1375, #15237 ) ;
#12948=CARTESIAN_POINT ( 'NONE',  ( 0.000000000000000000, 0.000000000000000000, -6.500000000000000000 ) ) ;
#12951=CARTESIAN_POINT ( 'NONE',  ( 30.78811501957141772, -4.393401135981229721, -6.500000000000000000 ) ) ;
#12952=DIRECTION ( 'NONE',  ( 0.000000000000000000, 0.000000000000000000, 1.000000000000000000 ) ) ;
#12955=VECTOR ( 'NONE', #17774, 1000.000000000000000 ) ;
#12956=ORIENTED_EDGE ( 'NONE', *, *, #3225, .F. ) ;
#12958=ORIENTED_EDGE ( 'NONE', *, *, #24655, .T. ) ;
#12959=DIRECTION ( 'NONE',  ( -0.000000000000000000, 0.000000000000000000, -1.000000000000000000 ) ) ;
#12962=FACE_OUTER_BOUND ( 'NONE', #11401, .T. ) ;
#12963=CARTESIAN_POINT ( 'NONE',  ( 0.000000000000000000, 0.000000000000000000, -6.500000000000000000 ) ) ;
#12964=AXIS2_PLACEMENT_3D ( 'NONE', #13357, #23670, #15706 ) ;
#12971=DIRECTION ( 'NONE',  ( 0.1253332335643120576, 0.9921147013144768767, 0.000000000000000000 ) ) ;
#12976=CIRCLE ( 'NONE', #8380, 0.5000000000000004441 ) ;
#12978=AXIS2_PLACEMENT_3D ( 'NONE', #13176, #21145, #3217 ) ;
#12979=CARTESIAN_POINT ( 'NONE',  ( -20.20656826142300133, -23.64116323484216053, -6.500000000000000000 ) ) ;
#12982=ORIENTED_EDGE ( 'NONE', *, *, #14439, .T. ) ;
#12984=ORIENTED_EDGE ( 'NONE', *, *, #23445, .T. ) ;
#12989=ORIENTED_EDGE ( 'NONE', *, *, #4988, .F. ) ;
#12992=ORIENTED_EDGE ( 'NONE', *, *, #24826, .T. ) ;
#12993=DIRECTION ( 'NONE',  ( 1.000000000000000000, 0.000000000000000000, 0.000000000000000000 ) ) ;
#12996=DIRECTION ( 'NONE',  ( 0.000000000000000000, 0.000000000000000000, 1.000000000000000000 ) ) ;
#12998=DIRECTION ( 'NONE',  ( 0.000000000000000000, 0.000000000000000000, 1.000000000000000000 ) ) ;
#12999=AXIS2_PLACEMENT_3D ( 'NONE', #1822, #18278, #2326 ) ;
#13003=AXIS2_PLACEMENT_3D ( 'NONE', #1007, #22444, #12378 ) ;
#13004=CYLINDRICAL_SURFACE ( 'NONE', #22571, 0.5000000000000004441 ) ;
#13007=CARTESIAN_POINT ( 'NONE',  ( 0.000000000000000000, 0.000000000000000000, -6.500000000000000000 ) ) ;
#13010=CIRCLE ( 'NONE', #18445, 0.5000000000000005551 ) ;
#13013=EDGE_CURVE ( 'NONE', #19667, #5148, #22112, .T. ) ;
#13018=DIRECTION ( 'NONE',  ( 0.000000000000000000, 0.000000000000000000, 1.000000000000000000 ) ) ;
#13020=ORIENTED_EDGE ( 'NONE', *, *, #308, .F. ) ;
#13021=DIRECTION ( 'NONE',  ( 0.000000000000000000, -0.000000000000000000, -1.000000000000000000 ) ) ;
#13023=DIRECTION ( 'NONE',  ( -0.000000000000000000, 0.000000000000000000, -1.000000000000000000 ) ) ;
#13025=ADVANCED_FACE ( 'NONE', ( #2702 ), #18921, .F. ) ;
#13029=EDGE_CURVE ( 'NONE', #13257, #9189, #14188, .T. ) ;
#13030=CIRCLE ( 'NONE', #13446, 0.4999999999999999445 ) ;
#13035=CARTESIAN_POINT ( 'NONE',  ( 25.98730014090442353, 17.08421000182768523, -6.500000000000000000 ) ) ;
#13036=CARTESIAN_POINT ( 'NONE',  ( -8.217531866531430751, -29.99470236596023653, -6.500000000000000000 ) ) ;
#13037=CIRCLE ( 'NONE', #10519, 0.4999999999999997224 ) ;
#13050=DIRECTION ( 'NONE',  ( 0.000000000000000000, 0.000000000000000000, 1.000000000000000000 ) ) ;
#13053=CYLINDRICAL_SURFACE ( 'NONE', #20444, 0.5000000000000004441 ) ;
#13055=CIRCLE ( 'NONE', #5003, 0.4999999999999998335 ) ;
#13058=ORIENTED_EDGE ( 'NONE', *, *, #23271, .T. ) ;
#13059=EDGE_CURVE ( 'NONE', #25447, #15051, #24805, .T. ) ;
#13061=VERTEX_POINT ( 'NONE', #10663 ) ;
#13063=CARTESIAN_POINT ( 'NONE',  ( 0.000000000000000000, 0.000000000000000000, -6.500000000000000000 ) ) ;
#13067=AXIS2_PLACEMENT_3D ( 'NONE', #3919, #4039, #12003 ) ;
#13069=DIRECTION ( 'NONE',  ( 0.000000000000000000, 0.000000000000000000, 1.000000000000000000 ) ) ;
#13071=AXIS2_PLACEMENT_3D ( 'NONE', #7732, #9820, #7852 ) ;
#13073=CYLINDRICAL_SURFACE ( 'NONE', #6326, 0.5000000000000004441 ) ;
#13076=DIRECTION ( 'NONE',  ( 0.2486898871648653975, 0.9685831611286285225, 0.000000000000000000 ) ) ;
#13079=CARTESIAN_POINT ( 'NONE',  ( 0.000000000000000000, 0.000000000000000000, 1.000000000000000000 ) ) ;
#13084=DIRECTION ( 'NONE',  ( -0.000000000000000000, -0.000000000000000000, 1.000000000000000000 ) ) ;
#13086=ORIENTED_EDGE ( 'NONE', *, *, #9041, .T. ) ;
#13090=AXIS2_PLACEMENT_3D ( 'NONE', #22285, #20709, #24623 ) ;
#13094=ORIENTED_EDGE ( 'NONE', *, *, #19921, .F. ) ;
#13095=EDGE_CURVE ( 'NONE', #18169, #10049, #20443, .T. ) ;
#13097=DIRECTION ( 'NONE',  ( -0.000000000000000000, -0.000000000000000000, 1.000000000000000000 ) ) ;
#13099=EDGE_CURVE ( 'NONE', #10033, #1701, #12082, .T. ) ;
#13103=DIRECTION ( 'NONE',  ( -1.000000000000000000, 0.000000000000000000, 0.000000000000000000 ) ) ;
#13104=CIRCLE ( 'NONE', #16450, 0.5000000000000001110 ) ;
#13106=EDGE_CURVE ( 'NONE', #10774, #5737, #1659, .T. ) ;
#13110=CARTESIAN_POINT ( 'NONE',  ( -23.64116323484210369, 20.20656826142307949, -2.750000000000000000 ) ) ;
#13111=FACE_OUTER_BOUND ( 'NONE', #20114, .T. ) ;
#13115=LINE ( 'NONE', #25265, #17464 ) ;
#13116=LINE ( 'NONE', #5515, #17246 ) ;
#13117=VERTEX_POINT ( 'NONE', #21514 ) ;
#13125=CARTESIAN_POINT ( 'NONE',  ( 0.000000000000000000, 0.000000000000000000, -6.500000000000000000 ) ) ;
#13133=LINE ( 'NONE', #18507, #17111 ) ;
#13139=EDGE_CURVE ( 'NONE', #3323, #3258, #11448, .T. ) ;
#13144=EDGE_CURVE ( 'NONE', #4479, #15851, #20864, .T. ) ;
#13145=ORIENTED_EDGE ( 'NONE', *, *, #11420, .F. ) ;
#13147=DIRECTION ( 'NONE',  ( -0.3681245526846659843, 0.9297764858882561212, 0.000000000000000000 ) ) ;
#13151=ORIENTED_EDGE ( 'NONE', *, *, #13347, .F. ) ;
#13152=ORIENTED_EDGE ( 'NONE', *, *, #23271, .F. ) ;
#13153=DIRECTION ( 'NONE',  ( 0.000000000000000000, 0.000000000000000000, 1.000000000000000000 ) ) ;
#13156=EDGE_CURVE ( 'NONE', #11375, #13603, #25049, .T. ) ;
#13161=EDGE_CURVE ( 'NONE', #13717, #5974, #19419, .T. ) ;
#13162=DIRECTION ( 'NONE',  ( 1.000000000000000000, 0.000000000000000000, 0.000000000000000000 ) ) ;
#13164=EDGE_CURVE ( 'NONE', #20076, #22016, #18364, .T. ) ;
#13176=CARTESIAN_POINT ( 'NONE',  ( 0.000000000000000000, 0.000000000000000000, -6.500000000000000000 ) ) ;
#13181=DIRECTION ( 'NONE',  ( -0.06279051952930156388, 0.9980267284282724471, 0.000000000000000000 ) ) ;
#13182=ORIENTED_EDGE ( 'NONE', *, *, #14434, .F. ) ;
#13186=ORIENTED_EDGE ( 'NONE', *, *, #9319, .T. ) ;
#13187=VERTEX_POINT ( 'NONE', #15135 ) ;
#13188=DIRECTION ( 'NONE',  ( 1.000000000000000000, 0.000000000000000000, 0.000000000000000000 ) ) ;
#13194=LINE ( 'NONE', #19454, #25502 ) ;
#13198=LINE ( 'NONE', #3242, #7035 ) ;
#13199=FACE_OUTER_BOUND ( 'NONE', #11605, .T. ) ;
#13200=EDGE_CURVE ( 'NONE', #17442, #8421, #16280, .T. ) ;
#13205=DIRECTION ( 'NONE',  ( 0.000000000000000000, 0.000000000000000000, -1.000000000000000000 ) ) ;
#13210=CARTESIAN_POINT ( 'NONE',  ( 0.000000000000000000, 0.000000000000000000, 1.000000000000000000 ) ) ;
#13212=EDGE_CURVE ( 'NONE', #10117, #674, #2498, .T. ) ;
#13213=ORIENTED_EDGE ( 'NONE', *, *, #2505, .F. ) ;
#13215=VERTEX_POINT ( 'NONE', #7393 ) ;
#13216=VERTEX_POINT ( 'NONE', #13036 ) ;
#13217=ORIENTED_EDGE ( 'NONE', *, *, #17469, .T. ) ;
#13218=CARTESIAN_POINT ( 'NONE',  ( 17.87326343783925253, -25.45105997952931176, -6.500000000000000000 ) ) ;
#13223=DIRECTION ( 'NONE',  ( 1.000000000000000000, 0.000000000000000000, 0.000000000000000000 ) ) ;
#13228=DIRECTION ( 'NONE',  ( 0.000000000000000000, 0.000000000000000000, 1.000000000000000000 ) ) ;
#13229=CARTESIAN_POINT ( 'NONE',  ( 0.000000000000000000, 0.000000000000000000, -6.500000000000000000 ) ) ;
#13230=FACE_OUTER_BOUND ( 'NONE', #2121, .T. ) ;
#13232=FACE_OUTER_BOUND ( 'NONE', #14247, .T. ) ;
#13234=CARTESIAN_POINT ( 'NONE',  ( -28.14012133169306296, 13.24173596767408867, -6.500000000000000000 ) ) ;
#13238=CARTESIAN_POINT ( 'NONE',  ( 0.000000000000000000, 31.10000000000000142, -6.500000000000000000 ) ) ;
#13243=DIRECTION ( 'NONE',  ( -0.000000000000000000, 0.000000000000000000, 1.000000000000000000 ) ) ;
#13245=CARTESIAN_POINT ( 'NONE',  ( -24.86329371854755266, 18.68225429291749151, 1.000000000000000000 ) ) ;
#13249=CARTESIAN_POINT ( 'NONE',  ( 7.248980000274197977, 30.24338421796781518, 1.000000000000000000 ) ) ;
#13250=FACE_OUTER_BOUND ( 'NONE', #6990, .T. ) ;
#13253=CARTESIAN_POINT ( 'NONE',  ( 7.734255490826784651, -30.12293631110048153, -6.500000000000000000 ) ) ;
#13257=VERTEX_POINT ( 'NONE', #3986 ) ;
#13258=ORIENTED_EDGE ( 'NONE', *, *, #15387, .F. ) ;
#13261=EDGE_LOOP ( 'NONE', ( #8004, #4263, #3527, #964 ) ) ;
#13262=LINE ( 'NONE', #3318, #3721 ) ;
#13263=EDGE_CURVE ( 'NONE', #6150, #14821, #3308, .T. ) ;
#13266=ORIENTED_EDGE ( 'NONE', *, *, #22155, .F. ) ;
#13267=ORIENTED_EDGE ( 'NONE', *, *, #13425, .F. ) ;
#13270=CIRCLE ( 'NONE', #14575, 31.10000000000000142 ) ;
#13272=CARTESIAN_POINT ( 'NONE',  ( 27.49048467073848911, -14.54246377227368647, -2.750000000000000000 ) ) ;
#13273=ORIENTED_EDGE ( 'NONE', *, *, #1206, .T. ) ;
#13284=AXIS2_PLACEMENT_3D ( 'NONE', #442, #18609, #16132 ) ;
#13289=CARTESIAN_POINT ( 'NONE',  ( 24.27856662945507438, 19.43607991388980238, -2.750000000000000000 ) ) ;
#13291=DIRECTION ( 'NONE',  ( 0.000000000000000000, 0.000000000000000000, 1.000000000000000000 ) ) ;
#13292=ADVANCED_FACE ( 'NONE', ( #15760 ), #21637, .F. ) ;
#13296=ORIENTED_EDGE ( 'NONE', *, *, #19247, .F. ) ;
#13301=VERTEX_POINT ( 'NONE', #23725 ) ;
#13303=EDGE_CURVE ( 'NONE', #10526, #13848, #16520, .T. ) ;
#13306=VERTEX_POINT ( 'NONE', #4599 ) ;
#13308=EDGE_CURVE ( 'NONE', #15503, #3397, #20885, .T. ) ;
#13311=CIRCLE ( 'NONE', #16653, 0.4999999999999998335 ) ;
#13312=CIRCLE ( 'NONE', #2027, 0.5000000000000013323 ) ;
#13316=VECTOR ( 'NONE', #23561, 1000.000000000000000 ) ;
#13317=CARTESIAN_POINT ( 'NONE',  ( -30.24338421796790044, -7.248980000273874680, -2.750000000000000000 ) ) ;
#13318=DIRECTION ( 'NONE',  ( 0.000000000000000000, 0.000000000000000000, 1.000000000000000000 ) ) ;
#13321=CARTESIAN_POINT ( 'NONE',  ( 29.99470236596029693, -8.217531866531192719, 1.000000000000000000 ) ) ;
#13323=CARTESIAN_POINT ( 'NONE',  ( -7.234255490827218082, -30.12293631110037140, -6.500000000000000000 ) ) ;
#13324=CYLINDRICAL_SURFACE ( 'NONE', #25150, 31.10000000000000142 ) ;
#13329=VECTOR ( 'NONE', #22494, 1000.000000000000000 ) ;
#13332=CIRCLE ( 'NONE', #23293, 0.4999999999999997224 ) ;
#13333=ORIENTED_EDGE ( 'NONE', *, *, #5886, .F. ) ;
#13335=CARTESIAN_POINT ( 'NONE',  ( -14.54246377227378062, -27.49048467073843227, -2.750000000000000000 ) ) ;
#13336=CARTESIAN_POINT ( 'NONE',  ( -27.25313774936430633, -14.98253926456308172, 1.000000000000000000 ) ) ;
#13337=EDGE_LOOP ( 'NONE', ( #15043, #12068, #22427, #7441 ) ) ;
#13338=AXIS2_PLACEMENT_3D ( 'NONE', #16590, #14626, #2721 ) ;
#13339=VERTEX_POINT ( 'NONE', #8654 ) ;
#13341=ORIENTED_EDGE ( 'NONE', *, *, #13161, .F. ) ;
#13342=ORIENTED_EDGE ( 'NONE', *, *, #308, .T. ) ;
#13345=CYLINDRICAL_SURFACE ( 'NONE', #25568, 31.10000000000000142 ) ;
#13347=EDGE_CURVE ( 'NONE', #23094, #3781, #2090, .T. ) ;
#13349=AXIS2_PLACEMENT_3D ( 'NONE', #14359, #10023, #18023 ) ;
#13350=ADVANCED_FACE ( 'NONE', ( #9045 ), #7217, .F. ) ;
#13353=CARTESIAN_POINT ( 'NONE',  ( 0.000000000000000000, 0.000000000000000000, 0.000000000000000000 ) ) ;
#13356=CIRCLE ( 'NONE', #1230, 31.10000000000000142 ) ;
#13357=CARTESIAN_POINT ( 'NONE',  ( -31.03863125411927371, -1.952785157361310198, 1.000000000000000000 ) ) ;
#13359=CIRCLE ( 'NONE', #20871, 31.10000000000000142 ) ;
#13362=CYLINDRICAL_SURFACE ( 'NONE', #15792, 0.5000000000000004441 ) ;
#13368=CARTESIAN_POINT ( 'NONE',  ( 15.41874213889403578, 27.00874656207305691, 1.000000000000000000 ) ) ;
#13370=LINE ( 'NONE', #13507, #21288 ) ;
#13372=AXIS2_PLACEMENT_3D ( 'NONE', #12581, #20561, #2650 ) ;
#13375=ORIENTED_EDGE ( 'NONE', *, *, #5804, .F. ) ;
#13379=AXIS2_PLACEMENT_3D ( 'NONE', #10155, #16175, #24140 ) ;
#13384=EDGE_CURVE ( 'NONE', #5285, #2848, #14812, .T. ) ;
#13385=CARTESIAN_POINT ( 'NONE',  ( -19.32388608118446527, -23.96296185032687376, 1.000000000000000000 ) ) ;
#13388=AXIS2_PLACEMENT_3D ( 'NONE', #16997, #7045, #12688 ) ;
#13395=DIRECTION ( 'NONE',  ( 1.000000000000000000, 0.000000000000000000, 0.000000000000000000 ) ) ;
#13406=CARTESIAN_POINT ( 'NONE',  ( -27.25313774936397948, 14.98253926456367502, -6.500000000000000000 ) ) ;
#13407=CIRCLE ( 'NONE', #6304, 0.5000000000000003331 ) ;
#13408=VECTOR ( 'NONE', #432, 1000.000000000000000 ) ;
#13410=ORIENTED_EDGE ( 'NONE', *, *, #4828, .F. ) ;
#13411=AXIS2_PLACEMENT_3D ( 'NONE', #24011, #20463, #484 ) ;
#13416=AXIS2_PLACEMENT_3D ( 'NONE', #20095, #13834, #18025 ) ;
#13421=EDGE_CURVE ( 'NONE', #20933, #25179, #7111, .T. ) ;
#13424=AXIS2_PLACEMENT_3D ( 'NONE', #14479, #24417, #22722 ) ;
#13425=EDGE_CURVE ( 'NONE', #12921, #20210, #16706, .T. ) ;
#13426=FACE_OUTER_BOUND ( 'NONE', #8276, .T. ) ;
#13438=ORIENTED_EDGE ( 'NONE', *, *, #16426, .T. ) ;
#13439=DIRECTION ( 'NONE',  ( 0.000000000000000000, -0.000000000000000000, 1.000000000000000000 ) ) ;
#13443=ORIENTED_EDGE ( 'NONE', *, *, #14964, .F. ) ;
#13446=AXIS2_PLACEMENT_3D ( 'NONE', #17615, #25593, #5970 ) ;
#13447=ORIENTED_EDGE ( 'NONE', *, *, #4563, .T. ) ;
#13449=ORIENTED_EDGE ( 'NONE', *, *, #5684, .F. ) ;
#13452=VECTOR ( 'NONE', #2031, 1000.000000000000000 ) ;
#13454=CIRCLE ( 'NONE', #15110, 0.4999999999999998335 ) ;
#13459=EDGE_CURVE ( 'NONE', #4812, #14631, #1262, .T. ) ;
#13460=CARTESIAN_POINT ( 'NONE',  ( 28.72825533807129261, -11.91206721063050189, 1.000000000000000000 ) ) ;
#13461=AXIS2_PLACEMENT_3D ( 'NONE', #1568, #5492, #25115 ) ;
#13475=CARTESIAN_POINT ( 'NONE',  ( 30.78811501957144969, 4.393401135981008565, -2.750000000000000000 ) ) ;
#13478=EDGE_CURVE ( 'NONE', #24860, #22793, #20033, .T. ) ;
#13479=CARTESIAN_POINT ( 'NONE',  ( 7.248980000274102942, -30.24338421796783649, 1.000000000000000000 ) ) ;
#13480=CARTESIAN_POINT ( 'NONE',  ( 0.000000000000000000, 0.000000000000000000, -6.500000000000000000 ) ) ;
#13482=ORIENTED_EDGE ( 'NONE', *, *, #17345, .F. ) ;
#13484=ORIENTED_EDGE ( 'NONE', *, *, #6435, .F. ) ;
#13486=DIRECTION ( 'NONE',  ( 0.000000000000000000, 0.000000000000000000, 1.000000000000000000 ) ) ;
#13488=CIRCLE ( 'NONE', #2198, 31.10000000000000142 ) ;
#13489=ADVANCED_FACE ( 'NONE', ( #22907 ), #4993, .F. ) ;
#13490=DIRECTION ( 'NONE',  ( 0.000000000000000000, 0.000000000000000000, 1.000000000000000000 ) ) ;
#13497=CARTESIAN_POINT ( 'NONE',  ( 30.63887302793247969, 5.335677986744675749, -2.750000000000000000 ) ) ;
#13498=DIRECTION ( 'NONE',  ( 0.000000000000000000, 0.000000000000000000, 1.000000000000000000 ) ) ;
#13499=EDGE_CURVE ( 'NONE', #7472, #24402, #438, .T. ) ;
#13502=CARTESIAN_POINT ( 'NONE',  ( -29.57785765677936851, -9.610428525060582317, 1.000000000000000000 ) ) ;
#13505=ORIENTED_EDGE ( 'NONE', *, *, #23557, .T. ) ;
#13506=EDGE_CURVE ( 'NONE', #11885, #12101, #25066, .T. ) ;
#13507=CARTESIAN_POINT ( 'NONE',  ( 27.00874656207294322, -15.41874213889423828, -2.750000000000000000 ) ) ;
#13508=ORIENTED_EDGE ( 'NONE', *, *, #6598, .F. ) ;
#13509=ADVANCED_FACE ( 'NONE', ( #690 ), #16635, .F. ) ;
#13510=ORIENTED_EDGE ( 'NONE', *, *, #14907, .F. ) ;
#13515=DIRECTION ( 'NONE',  ( -0.000000000000000000, 0.000000000000000000, 1.000000000000000000 ) ) ;
#13516=ORIENTED_EDGE ( 'NONE', *, *, #14403, .F. ) ;
#13520=DIRECTION ( 'NONE',  ( 0.000000000000000000, 0.000000000000000000, 1.000000000000000000 ) ) ;
#13529=EDGE_CURVE ( 'NONE', #19798, #13339, #8774, .T. ) ;
#13532=ADVANCED_FACE ( 'NONE', ( #7725 ), #5750, .F. ) ;
#13534=VERTEX_POINT ( 'NONE', #15451 ) ;
#13535=CARTESIAN_POINT ( 'NONE',  ( -7.734255490826573265, 30.12293631110053838, 1.000000000000000000 ) ) ;
#13541=CARTESIAN_POINT ( 'NONE',  ( -22.67092431280563503, 21.28941499438250062, -6.500000000000000000 ) ) ;
#13544=LINE ( 'NONE', #23336, #2192 ) ;
#13551=CYLINDRICAL_SURFACE ( 'NONE', #8408, 0.5000000000000004441 ) ;
#13555=EDGE_CURVE ( 'NONE', #20939, #1141, #4604, .T. ) ;
#13568=DIRECTION ( 'NONE',  ( 1.000000000000000000, 0.000000000000000000, 0.000000000000000000 ) ) ;
#13572=ORIENTED_EDGE ( 'NONE', *, *, #19626, .F. ) ;
#13582=DIRECTION ( 'NONE',  ( -0.4817536741017198754, -0.8763066800438610304, 0.000000000000000000 ) ) ;
#13585=VERTEX_POINT ( 'NONE', #3798 ) ;
#13595=DIRECTION ( 'NONE',  ( 0.000000000000000000, -0.000000000000000000, 1.000000000000000000 ) ) ;
#13596=CYLINDRICAL_SURFACE ( 'NONE', #2910, 31.10000000000000142 ) ;
#13598=ORIENTED_EDGE ( 'NONE', *, *, #5684, .T. ) ;
#13601=ORIENTED_EDGE ( 'NONE', *, *, #15136, .T. ) ;
#13603=VERTEX_POINT ( 'NONE', #11639 ) ;
#13606=LINE ( 'NONE', #21572, #2667 ) ;
#13607=EDGE_CURVE ( 'NONE', #8280, #1701, #25763, .T. ) ;
#13608=AXIS2_PLACEMENT_3D ( 'NONE', #21188, #11240, #23277 ) ;
#13612=DIRECTION ( 'NONE',  ( 0.000000000000000000, 0.000000000000000000, 1.000000000000000000 ) ) ;
#13613=CARTESIAN_POINT ( 'NONE',  ( 23.01025686871630782, -20.92219106202058754, -6.500000000000000000 ) ) ;
#13617=LINE ( 'NONE', #13497, #22476 ) ;
#13623=LINE ( 'NONE', #7607, #18086 ) ;
#13625=CYLINDRICAL_SURFACE ( 'NONE', #5424, 0.5000000000000004441 ) ;
#13628=CARTESIAN_POINT ( 'NONE',  ( -19.32388608118446527, -23.96296185032687376, -6.500000000000000000 ) ) ;
#13631=ORIENTED_EDGE ( 'NONE', *, *, #15566, .F. ) ;
#13632=CARTESIAN_POINT ( 'NONE',  ( -4.393401135980685268, 30.78811501957149588, -6.500000000000000000 ) ) ;
#13634=ORIENTED_EDGE ( 'NONE', *, *, #2638, .T. ) ;
#13638=CARTESIAN_POINT ( 'NONE',  ( 31.06601413805602618, 1.453535542772499856, -6.500000000000000000 ) ) ;
#13639=CARTESIAN_POINT ( 'NONE',  ( -30.54913349766215802, 5.827558883616378083, 1.000000000000000000 ) ) ;
#13641=EDGE_CURVE ( 'NONE', #25152, #24761, #2930, .T. ) ;
#13645=DIRECTION ( 'NONE',  ( 0.000000000000000000, 0.000000000000000000, 1.000000000000000000 ) ) ;
#13647=VERTEX_POINT ( 'NONE', #23802 ) ;
#13650=ORIENTED_EDGE ( 'NONE', *, *, #5915, .T. ) ;
#13653=CARTESIAN_POINT ( 'NONE',  ( 1.453535542772391942, -31.06601413805603329, -6.500000000000000000 ) ) ;
#13655=ORIENTED_EDGE ( 'NONE', *, *, #13421, .T. ) ;
#13656=CARTESIAN_POINT ( 'NONE',  ( 31.09598070739550479, 0.4999838450258676792, -2.750000000000000000 ) ) ;
#13657=ORIENTED_EDGE ( 'NONE', *, *, #1724, .T. ) ;
#13659=CARTESIAN_POINT ( 'NONE',  ( -24.66042852506064165, 18.28012134629622309, 1.000000000000000000 ) ) ;
#13664=EDGE_CURVE ( 'NONE', #5148, #15562, #11280, .T. ) ;
#13667=EDGE_CURVE ( 'NONE', #5989, #6393, #12537, .T. ) ;
#13668=CARTESIAN_POINT ( 'NONE',  ( -20.78941499438192508, 22.67092431280617859, -6.500000000000000000 ) ) ;
#13676=CARTESIAN_POINT ( 'NONE',  ( 4.393401135980900207, -30.78811501957146390, -2.750000000000000000 ) ) ;
#13681=ORIENTED_EDGE ( 'NONE', *, *, #782, .T. ) ;
#13685=DIRECTION ( 'NONE',  ( 0.000000000000000000, 0.000000000000000000, 1.000000000000000000 ) ) ;
#13686=VERTEX_POINT ( 'NONE', #23554 ) ;
#13687=ORIENTED_EDGE ( 'NONE', *, *, #6708, .F. ) ;
#13688=DIRECTION ( 'NONE',  ( 0.000000000000000000, 0.000000000000000000, 1.000000000000000000 ) ) ;
#13693=AXIS2_PLACEMENT_3D ( 'NONE', #9050, #23292, #22914 ) ;
#13696=CARTESIAN_POINT ( 'NONE',  ( 30.91344420362548107, 3.401318489840985837, -6.500000000000000000 ) ) ;
#13697=CARTESIAN_POINT ( 'NONE',  ( -29.09636799667091367, -10.98232076577190774, -2.750000000000000000 ) ) ;
#13698=CARTESIAN_POINT ( 'NONE',  ( 30.45149776762727356, -6.317933499823421784, 1.000000000000000000 ) ) ;
#13699=FACE_OUTER_BOUND ( 'NONE', #16137, .T. ) ;
#13701=CARTESIAN_POINT ( 'NONE',  ( -16.23990935651690748, 26.52310962334761157, 1.000000000000000000 ) ) ;
#13703=VERTEX_POINT ( 'NONE', #6142 ) ;
#13708=DIRECTION ( 'NONE',  ( 0.000000000000000000, 0.000000000000000000, 1.000000000000000000 ) ) ;
#13714=ORIENTED_EDGE ( 'NONE', *, *, #7238, .F. ) ;
#13717=VERTEX_POINT ( 'NONE', #12292 ) ;
#13718=ORIENTED_EDGE ( 'NONE', *, *, #23187, .T. ) ;
#13719=CARTESIAN_POINT ( 'NONE',  ( 0.000000000000000000, 0.000000000000000000, -6.500000000000000000 ) ) ;
#13722=VECTOR ( 'NONE', #17264, 1000.000000000000000 ) ;
#13724=DIRECTION ( 'NONE',  ( 0.000000000000000000, 0.000000000000000000, 1.000000000000000000 ) ) ;
#13731=ADVANCED_FACE ( 'NONE', ( #14002 ), #2098, .F. ) ;
#13733=AXIS2_PLACEMENT_3D ( 'NONE', #16041, #14067, #4501 ) ;
#13734=DIRECTION ( 'NONE',  ( 0.000000000000000000, 0.000000000000000000, 1.000000000000000000 ) ) ;
#13737=CARTESIAN_POINT ( 'NONE',  ( 0.000000000000000000, 0.000000000000000000, 1.000000000000000000 ) ) ;
#13739=DIRECTION ( 'NONE',  ( 0.000000000000000000, 0.000000000000000000, 1.000000000000000000 ) ) ;
#13742=VECTOR ( 'NONE', #17068, 1000.000000000000000 ) ;
#13743=DIRECTION ( 'NONE',  ( 1.000000000000000000, 0.000000000000000000, -0.000000000000000000 ) ) ;
#13744=AXIS2_PLACEMENT_3D ( 'NONE', #19205, #21307, #9285 ) ;
#13747=ORIENTED_EDGE ( 'NONE', *, *, #18103, .T. ) ;
#13749=ORIENTED_EDGE ( 'NONE', *, *, #5336, .F. ) ;
#13753=ORIENTED_EDGE ( 'NONE', *, *, #5206, .T. ) ;
#13755=AXIS2_PLACEMENT_3D ( 'NONE', #15687, #11882, #1831 ) ;
#13756=ORIENTED_EDGE ( 'NONE', *, *, #7074, .T. ) ;
#13759=CIRCLE ( 'NONE', #20429, 0.5000000000000005551 ) ;
#13761=CYLINDRICAL_SURFACE ( 'NONE', #7982, 0.5000000000000004441 ) ;
#13765=ADVANCED_FACE ( 'NONE', ( #6021 ), #14126, .T. ) ;
#13768=AXIS2_PLACEMENT_3D ( 'NONE', #6539, #16371, #24336 ) ;
#13770=AXIS2_PLACEMENT_3D ( 'NONE', #8203, #6232, #4140 ) ;
#13772=EDGE_CURVE ( 'NONE', #4937, #8646, #15974, .T. ) ;
#13773=CARTESIAN_POINT ( 'NONE',  ( -6.317933499823659815, -30.45149776762723093, -2.750000000000000000 ) ) ;
#13775=AXIS2_PLACEMENT_3D ( 'NONE', #14759, #16715, #22858 ) ;
#13780=ORIENTED_EDGE ( 'NONE', *, *, #6590, .F. ) ;
#13782=CIRCLE ( 'NONE', #21243, 31.10000000000000142 ) ;
#13784=CARTESIAN_POINT ( 'NONE',  ( 0.000000000000000000, 0.000000000000000000, -6.500000000000000000 ) ) ;
#13785=EDGE_CURVE ( 'NONE', #11788, #19594, #39, .T. ) ;
#13786=ORIENTED_EDGE ( 'NONE', *, *, #25003, .T. ) ;
#13787=VERTEX_POINT ( 'NONE', #11900 ) ;
#13788=DIRECTION ( 'NONE',  ( 0.6845471059286972748, 0.7289686274214034478, 0.000000000000000000 ) ) ;
#13790=ORIENTED_EDGE ( 'NONE', *, *, #19445, .F. ) ;
#13792=DIRECTION ( 'NONE',  ( 0.000000000000000000, 0.000000000000000000, 1.000000000000000000 ) ) ;
#13795=CIRCLE ( 'NONE', #17569, 0.5000000000000003331 ) ;
#13798=CIRCLE ( 'NONE', #6699, 31.10000000000000142 ) ;
#13799=CARTESIAN_POINT ( 'NONE',  ( 18.28012134629595309, 25.16042852506084770, 1.000000000000000000 ) ) ;
#13801=CARTESIAN_POINT ( 'NONE',  ( -24.66042852506104310, -18.28012134629567598, -6.500000000000000000 ) ) ;
#13804=EDGE_CURVE ( 'NONE', #13187, #14350, #2948, .T. ) ;
#13805=DIRECTION ( 'NONE',  ( 0.000000000000000000, 0.000000000000000000, 1.000000000000000000 ) ) ;
#13807=AXIS2_PLACEMENT_3D ( 'NONE', #22354, #8120, #19994 ) ;
#13809=AXIS2_PLACEMENT_3D ( 'NONE', #9581, #25544, #1993 ) ;
#13811=CARTESIAN_POINT ( 'NONE',  ( -12.78762572734076919, -28.34936733434192035, -6.500000000000000000 ) ) ;
#13815=EDGE_CURVE ( 'NONE', #10117, #3578, #16729, .T. ) ;
#13817=ORIENTED_EDGE ( 'NONE', *, *, #4215, .T. ) ;
#13819=AXIS2_PLACEMENT_3D ( 'NONE', #15970, #18063, #7841 ) ;
#13820=ADVANCED_FACE ( 'NONE', ( #19868 ), #16095, .F. ) ;
#13829=AXIS2_PLACEMENT_3D ( 'NONE', #18792, #12782, #2832 ) ;
#13834=DIRECTION ( 'NONE',  ( 0.000000000000000000, 0.000000000000000000, 1.000000000000000000 ) ) ;
#13835=DIRECTION ( 'NONE',  ( 0.000000000000000000, 0.000000000000000000, 1.000000000000000000 ) ) ;
#13840=EDGE_LOOP ( 'NONE', ( #13857, #12956, #4161, #21695 ) ) ;
#13844=CARTESIAN_POINT ( 'NONE',  ( -11.44867358849309547, 28.91604871112477326, -6.500000000000000000 ) ) ;
#13845=AXIS2_PLACEMENT_3D ( 'NONE', #5775, #12043, #11803 ) ;
#13846=EDGE_CURVE ( 'NONE', #2002, #5285, #23830, .T. ) ;
#13848=VERTEX_POINT ( 'NONE', #12411 ) ;
#13850=CARTESIAN_POINT ( 'NONE',  ( 31.03863125411924173, -1.952785157361756951, -6.500000000000000000 ) ) ;
#13853=VECTOR ( 'NONE', #15299, 1000.000000000000000 ) ;
#13854=EDGE_CURVE ( 'NONE', #10597, #2759, #11300, .T. ) ;
#13857=ORIENTED_EDGE ( 'NONE', *, *, #14297, .F. ) ;
#13859=VERTEX_POINT ( 'NONE', #24186 ) ;
#13861=AXIS2_PLACEMENT_3D ( 'NONE', #7658, #7908, #15895 ) ;
#13862=FACE_BOUND ( 'NONE', #3187, .T. ) ;
#13865=AXIS2_PLACEMENT_3D ( 'NONE', #3824, #19641, #15611 ) ;
#13868=AXIS2_PLACEMENT_3D ( 'NONE', #18186, #20256, #10308 ) ;
#13870=CIRCLE ( 'NONE', #24322, 31.10000000000000142 ) ;
#13871=DIRECTION ( 'NONE',  ( 0.000000000000000000, -0.000000000000000000, 1.000000000000000000 ) ) ;
#13872=CYLINDRICAL_SURFACE ( 'NONE', #5931, 0.5000000000000004441 ) ;
#13874=AXIS2_PLACEMENT_3D ( 'NONE', #25308, #13792, #7649 ) ;
#13875=CARTESIAN_POINT ( 'NONE',  ( -7.734255490826573265, 30.12293631110053838, -6.500000000000000000 ) ) ;
#13879=AXIS2_PLACEMENT_3D ( 'NONE', #24412, #6607, #12373 ) ;
#13881=CARTESIAN_POINT ( 'NONE',  ( -7.734255490827218971, -30.12293631110037140, 1.000000000000000000 ) ) ;
#13887=ORIENTED_EDGE ( 'NONE', *, *, #13106, .F. ) ;
#13888=EDGE_CURVE ( 'NONE', #19523, #25423, #6275, .T. ) ;
#13889=AXIS2_PLACEMENT_3D ( 'NONE', #20398, #14798, #24346 ) ;
#13890=VERTEX_POINT ( 'NONE', #18305 ) ;
#13891=DIRECTION ( 'NONE',  ( 0.000000000000000000, 0.000000000000000000, 1.000000000000000000 ) ) ;
#13898=ORIENTED_EDGE ( 'NONE', *, *, #9394, .F. ) ;
#13905=DIRECTION ( 'NONE',  ( 0.000000000000000000, 0.000000000000000000, 1.000000000000000000 ) ) ;
#13907=DIRECTION ( 'NONE',  ( 1.000000000000000000, 0.000000000000000000, 0.000000000000000000 ) ) ;
#13914=ORIENTED_EDGE ( 'NONE', *, *, #25003, .F. ) ;
#13917=ORIENTED_EDGE ( 'NONE', *, *, #2012, .T. ) ;
#13918=LINE ( 'NONE', #3701, #21900 ) ;
#13922=DIRECTION ( 'NONE',  ( 0.000000000000000000, 0.000000000000000000, 1.000000000000000000 ) ) ;
#13923=ORIENTED_EDGE ( 'NONE', *, *, #20430, .F. ) ;
#13926=ADVANCED_FACE ( 'NONE', ( #18688 ), #3002, .F. ) ;
#13928=ORIENTED_EDGE ( 'NONE', *, *, #20315, .F. ) ;
#13932=EDGE_CURVE ( 'NONE', #15879, #25564, #2740, .T. ) ;
#13933=DIRECTION ( 'NONE',  ( 0.5877852522924730261, -0.8090169943749474513, 0.000000000000000000 ) ) ;
#13938=CARTESIAN_POINT ( 'NONE',  ( -24.27856662945480792, 19.43607991389014344, 1.000000000000000000 ) ) ;
#13939=CIRCLE ( 'NONE', #21873, 0.5000000000000002220 ) ;
#13944=CYLINDRICAL_SURFACE ( 'NONE', #11223, 0.5000000000000004441 ) ;
#13945=CARTESIAN_POINT ( 'NONE',  ( -14.54246377227378062, -27.49048467073843227, 1.000000000000000000 ) ) ;
#13951=EDGE_LOOP ( 'NONE', ( #15186, #2688, #18664, #6815 ) ) ;
#13955=FACE_OUTER_BOUND ( 'NONE', #25248, .T. ) ;
#13956=ORIENTED_EDGE ( 'NONE', *, *, #22471, .F. ) ;
#13957=ORIENTED_EDGE ( 'NONE', *, *, #23689, .F. ) ;
#13959=EDGE_CURVE ( 'NONE', #13534, #24264, #18816, .T. ) ;
#13963=CARTESIAN_POINT ( 'NONE',  ( -18.68225429291750928, -24.86329371854754200, -6.500000000000000000 ) ) ;
#13965=DIRECTION ( 'NONE',  ( 0.000000000000000000, 0.000000000000000000, 1.000000000000000000 ) ) ;
#13967=FACE_OUTER_BOUND ( 'NONE', #23784, .T. ) ;
#13970=CYLINDRICAL_SURFACE ( 'NONE', #9959, 0.5000000000000004441 ) ;
#13971=CARTESIAN_POINT ( 'NONE',  ( -9.133673601486680838, -29.72853858738275434, -2.750000000000000000 ) ) ;
#13973=ORIENTED_EDGE ( 'NONE', *, *, #21773, .T. ) ;
#13974=DIRECTION ( 'NONE',  ( 1.000000000000000000, 0.000000000000000000, 0.000000000000000000 ) ) ;
#13981=DIRECTION ( 'NONE',  ( -0.000000000000000000, -0.000000000000000000, 1.000000000000000000 ) ) ;
#13985=EDGE_LOOP ( 'NONE', ( #16685, #15105, #14016, #20542 ) ) ;
#13986=ORIENTED_EDGE ( 'NONE', *, *, #4067, .F. ) ;
#13987=ORIENTED_EDGE ( 'NONE', *, *, #17014, .F. ) ;
#13989=CYLINDRICAL_SURFACE ( 'NONE', #13067, 31.10000000000000142 ) ;
#13996=EDGE_CURVE ( 'NONE', #9053, #12491, #10024, .T. ) ;
#14002=FACE_OUTER_BOUND ( 'NONE', #4331, .T. ) ;
#14006=EDGE_CURVE ( 'NONE', #18011, #19944, #6290, .T. ) ;
#14008=DIRECTION ( 'NONE',  ( 0.000000000000000000, 0.000000000000000000, 1.000000000000000000 ) ) ;
#14009=EDGE_CURVE ( 'NONE', #674, #14282, #16314, .T. ) ;
#14013=ORIENTED_EDGE ( 'NONE', *, *, #8635, .F. ) ;
#14014=DIRECTION ( 'NONE',  ( 0.000000000000000000, 0.000000000000000000, 1.000000000000000000 ) ) ;
#14016=ORIENTED_EDGE ( 'NONE', *, *, #22549, .F. ) ;
#14019=EDGE_CURVE ( 'NONE', #24045, #7204, #14222, .T. ) ;
#14021=ORIENTED_EDGE ( 'NONE', *, *, #3069, .F. ) ;
#14024=ORIENTED_EDGE ( 'NONE', *, *, #3740, .F. ) ;
#14026=CARTESIAN_POINT ( 'NONE',  ( 30.12293631110045311, 7.734255490826897450, -6.500000000000000000 ) ) ;
#14028=DIRECTION ( 'NONE',  ( 1.000000000000000000, 0.000000000000000000, 0.000000000000000000 ) ) ;
#14030=AXIS2_PLACEMENT_3D ( 'NONE', #680, #24864, #2760 ) ;
#14033=EDGE_CURVE ( 'NONE', #14041, #23505, #9624, .T. ) ;
#14038=DIRECTION ( 'NONE',  ( -0.000000000000000000, 0.000000000000000000, 1.000000000000000000 ) ) ;
#14039=VECTOR ( 'NONE', #8110, 1000.000000000000000 ) ;
#14040=ORIENTED_EDGE ( 'NONE', *, *, #17162, .F. ) ;
#14041=VERTEX_POINT ( 'NONE', #11602 ) ;
#14043=EDGE_CURVE ( 'NONE', #12524, #16720, #12976, .T. ) ;
#14044=EDGE_LOOP ( 'NONE', ( #2397, #20537, #5282, #20793 ) ) ;
#14045=DIRECTION ( 'NONE',  ( 0.000000000000000000, 0.000000000000000000, 1.000000000000000000 ) ) ;
#14048=CARTESIAN_POINT ( 'NONE',  ( 0.000000000000000000, 0.000000000000000000, -6.500000000000000000 ) ) ;
#14049=ORIENTED_EDGE ( 'NONE', *, *, #19996, .T. ) ;
#14051=ORIENTED_EDGE ( 'NONE', *, *, #18537, .T. ) ;
#14052=CARTESIAN_POINT ( 'NONE',  ( 0.000000000000000000, 0.000000000000000000, -6.500000000000000000 ) ) ;
#14054=CARTESIAN_POINT ( 'NONE',  ( 0.000000000000000000, 0.000000000000000000, -6.500000000000000000 ) ) ;
#14062=CARTESIAN_POINT ( 'NONE',  ( -22.67092431280609688, -21.28941499438201745, 1.000000000000000000 ) ) ;
#14067=DIRECTION ( 'NONE',  ( -0.000000000000000000, -0.000000000000000000, 1.000000000000000000 ) ) ;
#14074=EDGE_CURVE ( 'NONE', #20492, #3679, #3785, .T. ) ;
#14078=ORIENTED_EDGE ( 'NONE', *, *, #10670, .F. ) ;
#14079=ORIENTED_EDGE ( 'NONE', *, *, #19516, .F. ) ;
#14082=DIRECTION ( 'NONE',  ( 0.000000000000000000, 0.000000000000000000, 1.000000000000000000 ) ) ;
#14084=FACE_OUTER_BOUND ( 'NONE', #24830, .T. ) ;
#14088=DIRECTION ( 'NONE',  ( -0.000000000000000000, 0.000000000000000000, -1.000000000000000000 ) ) ;
#14091=DIRECTION ( 'NONE',  ( -0.000000000000000000, -0.000000000000000000, 1.000000000000000000 ) ) ;
#14093=DIRECTION ( 'NONE',  ( 0.000000000000000000, 0.000000000000000000, 1.000000000000000000 ) ) ;
#14095=ORIENTED_EDGE ( 'NONE', *, *, #14893, .F. ) ;
#14099=DIRECTION ( 'NONE',  ( 1.000000000000000000, 0.000000000000000000, 0.000000000000000000 ) ) ;
#14100=EDGE_CURVE ( 'NONE', #10597, #9053, #23642, .T. ) ;
#14101=CARTESIAN_POINT ( 'NONE',  ( 11.44867358849351113, 28.91604871112461339, 1.000000000000000000 ) ) ;
#14106=DIRECTION ( 'NONE',  ( -0.06279051952931542779, -0.9980267284282714479, 0.000000000000000000 ) ) ;
#14110=ORIENTED_EDGE ( 'NONE', *, *, #25853, .T. ) ;
#14111=ORIENTED_EDGE ( 'NONE', *, *, #22417, .T. ) ;
#14112=ADVANCED_FACE ( 'NONE', ( #11355 ), #1548, .T. ) ;
#14113=ORIENTED_EDGE ( 'NONE', *, *, #9832, .F. ) ;
#14114=DIRECTION ( 'NONE',  ( 0.000000000000000000, -0.000000000000000000, -1.000000000000000000 ) ) ;
#14126=CYLINDRICAL_SURFACE ( 'NONE', #6712, 31.10000000000000142 ) ;
#14128=DIRECTION ( 'NONE',  ( -0.6845471059286901694, -0.7289686274214101092, 0.000000000000000000 ) ) ;
#14131=DIRECTION ( 'NONE',  ( 0.000000000000000000, 0.000000000000000000, 1.000000000000000000 ) ) ;
#14135=DIRECTION ( 'NONE',  ( -0.000000000000000000, -0.000000000000000000, 1.000000000000000000 ) ) ;
#14140=ORIENTED_EDGE ( 'NONE', *, *, #15011, .T. ) ;
#14144=VERTEX_POINT ( 'NONE', #17761 ) ;
#14145=ORIENTED_EDGE ( 'NONE', *, *, #24655, .F. ) ;
#14155=CYLINDRICAL_SURFACE ( 'NONE', #12559, 31.10000000000000142 ) ;
#14156=CIRCLE ( 'NONE', #2877, 31.10000000000000142 ) ;
#14158=AXIS2_PLACEMENT_3D ( 'NONE', #23013, #14093, #20099 ) ;
#14163=FACE_OUTER_BOUND ( 'NONE', #23960, .T. ) ;
#14165=EDGE_LOOP ( 'NONE', ( #4760, #20, #13601, #8824 ) ) ;
#14175=VECTOR ( 'NONE', #2674, 1000.000000000000000 ) ;
#14176=ADVANCED_FACE ( 'NONE', ( #11869 ), #13970, .F. ) ;
#14177=FACE_OUTER_BOUND ( 'NONE', #4481, .T. ) ;
#14178=CIRCLE ( 'NONE', #24602, 0.4999999999999983902 ) ;
#14179=ORIENTED_EDGE ( 'NONE', *, *, #15758, .F. ) ;
#14183=AXIS2_PLACEMENT_3D ( 'NONE', #13238, #11525, #17422 ) ;
#14184=DIRECTION ( 'NONE',  ( -0.9980267284282718920, -0.06279051952930848890, 0.000000000000000000 ) ) ;
#14188=CIRCLE ( 'NONE', #4151, 0.4999999999999999445 ) ;
#14189=CIRCLE ( 'NONE', #5811, 31.10000000000000142 ) ;
#14190=AXIS2_PLACEMENT_3D ( 'NONE', #7807, #15927, #24022 ) ;
#14192=AXIS2_PLACEMENT_3D ( 'NONE', #16648, #24099, #8281 ) ;
#14193=DIRECTION ( 'NONE',  ( 0.000000000000000000, 0.000000000000000000, 1.000000000000000000 ) ) ;
#14194=CARTESIAN_POINT ( 'NONE',  ( -11.44867358849309547, 28.91604871112477326, -6.500000000000000000 ) ) ;
#14199=AXIS2_PLACEMENT_3D ( 'NONE', #11496, #17277, #25242 ) ;
#14210=ORIENTED_EDGE ( 'NONE', *, *, #13772, .F. ) ;
#14211=ORIENTED_EDGE ( 'NONE', *, *, #20030, .F. ) ;
#14214=FACE_OUTER_BOUND ( 'NONE', #2798, .T. ) ;
#14219=AXIS2_PLACEMENT_3D ( 'NONE', #9794, #19971, #15563 ) ;
#14221=LINE ( 'NONE', #20342, #15438 ) ;
#14222=CIRCLE ( 'NONE', #19644, 0.4999999999999996669 ) ;
#14224=CARTESIAN_POINT ( 'NONE',  ( -28.34936733434213707, -12.78762572734027181, -6.500000000000000000 ) ) ;
#14225=DIRECTION ( 'NONE',  ( 1.000000000000000000, 0.000000000000000000, 0.000000000000000000 ) ) ;
#14230=CIRCLE ( 'NONE', #2953, 0.5000000000000007772 ) ;
#14231=ORIENTED_EDGE ( 'NONE', *, *, #1844, .T. ) ;
#14232=DIRECTION ( 'NONE',  ( 0.000000000000000000, 0.000000000000000000, 1.000000000000000000 ) ) ;
#14237=ORIENTED_EDGE ( 'NONE', *, *, #6750, .F. ) ;
#14238=CARTESIAN_POINT ( 'NONE',  ( -23.96296185032722548, -19.82388608118403539, 1.000000000000000000 ) ) ;
#14239=CARTESIAN_POINT ( 'NONE',  ( 30.54913349766223973, 5.827558883615938434, -6.500000000000000000 ) ) ;
#14246=CIRCLE ( 'NONE', #17580, 31.10000000000000142 ) ;
#14247=EDGE_LOOP ( 'NONE', ( #8106, #24980, #5116, #13186 ) ) ;
#14250=DIRECTION ( 'NONE',  ( -0.9048270524660229075, -0.4257792915650654986, 0.000000000000000000 ) ) ;
#14251=CIRCLE ( 'NONE', #5462, 31.10000000000000142 ) ;
#14254=EDGE_CURVE ( 'NONE', #5166, #1446, #25414, .T. ) ;
#14255=CARTESIAN_POINT ( 'NONE',  ( -28.91604871112473418, -11.44867358849319849, -6.500000000000000000 ) ) ;
#14256=CIRCLE ( 'NONE', #22180, 31.10000000000000142 ) ;
#14263=AXIS2_PLACEMENT_3D ( 'NONE', #15756, #23720, #19918 ) ;
#14266=CARTESIAN_POINT ( 'NONE',  ( -31.09598070739550124, 0.4999838450263022760, -2.750000000000000000 ) ) ;
#14268=EDGE_CURVE ( 'NONE', #3560, #9004, #3276, .T. ) ;
#14269=DIRECTION ( 'NONE',  ( 1.000000000000000000, 0.000000000000000000, 0.000000000000000000 ) ) ;
#14271=AXIS2_PLACEMENT_3D ( 'NONE', #17601, #17470, #1647 ) ;
#14272=CARTESIAN_POINT ( 'NONE',  ( 27.92360179968367362, -13.69242354489163027, -2.750000000000000000 ) ) ;
#14273=VECTOR ( 'NONE', #24749, 1000.000000000000000 ) ;
#14275=DIRECTION ( 'NONE',  ( 0.000000000000000000, 0.000000000000000000, 1.000000000000000000 ) ) ;
#14276=DIRECTION ( 'NONE',  ( 0.000000000000000000, -0.000000000000000000, 1.000000000000000000 ) ) ;
#14279=FACE_OUTER_BOUND ( 'NONE', #6700, .T. ) ;
#14282=VERTEX_POINT ( 'NONE', #500 ) ;
#14286=ORIENTED_EDGE ( 'NONE', *, *, #19626, .T. ) ;
#14289=AXIS2_PLACEMENT_3D ( 'NONE', #22717, #12891, #19986 ) ;
#14290=ORIENTED_EDGE ( 'NONE', *, *, #24055, .F. ) ;
#14291=CYLINDRICAL_SURFACE ( 'NONE', #8166, 0.5000000000000004441 ) ;
#14293=AXIS2_PLACEMENT_3D ( 'NONE', #396, #2232, #6018 ) ;
#14295=CARTESIAN_POINT ( 'NONE',  ( -20.20656826142290541, -23.64116323484223869, 1.000000000000000000 ) ) ;
#14297=EDGE_CURVE ( 'NONE', #18150, #22371, #21938, .T. ) ;
#14302=ADVANCED_FACE ( 'NONE', ( #19958 ), #14870, .F. ) ;
#14303=CARTESIAN_POINT ( 'NONE',  ( -29.72853858738291422, -9.133673601486165694, -6.500000000000000000 ) ) ;
#14309=CIRCLE ( 'NONE', #17635, 0.5000000000000001110 ) ;
#14311=ORIENTED_EDGE ( 'NONE', *, *, #4172, .T. ) ;
#14313=CIRCLE ( 'NONE', #1779, 31.10000000000000142 ) ;
#14316=CARTESIAN_POINT ( 'NONE',  ( 17.08421000182766747, 25.98730014090443063, 1.000000000000000000 ) ) ;
#14324=FACE_OUTER_BOUND ( 'NONE', #13951, .T. ) ;
#14327=DIRECTION ( 'NONE',  ( 1.000000000000000000, 0.000000000000000000, 0.000000000000000000 ) ) ;
#14329=CIRCLE ( 'NONE', #11381, 0.5000000000000004441 ) ;
#14330=EDGE_CURVE ( 'NONE', #6385, #21955, #13312, .T. ) ;
#14332=EDGE_CURVE ( 'NONE', #4508, #2838, #11638, .T. ) ;
#14336=EDGE_CURVE ( 'NONE', #5148, #6810, #14995, .T. ) ;
#14338=LINE ( 'NONE', #23877, #6223 ) ;
#14339=DIRECTION ( 'NONE',  ( 0.000000000000000000, 0.000000000000000000, 1.000000000000000000 ) ) ;
#14344=ORIENTED_EDGE ( 'NONE', *, *, #20315, .T. ) ;
#14345=ORIENTED_EDGE ( 'NONE', *, *, #11954, .F. ) ;
#14347=CARTESIAN_POINT ( 'NONE',  ( 0.000000000000000000, 0.000000000000000000, -6.500000000000000000 ) ) ;
#14349=VERTEX_POINT ( 'NONE', #12508 ) ;
#14350=VERTEX_POINT ( 'NONE', #5061 ) ;
#14353=DIRECTION ( 'NONE',  ( -1.000000000000000000, 0.000000000000000000, 0.000000000000000000 ) ) ;
#14356=CIRCLE ( 'NONE', #15610, 0.5000000000000019984 ) ;
#14359=CARTESIAN_POINT ( 'NONE',  ( 0.000000000000000000, 0.000000000000000000, -6.500000000000000000 ) ) ;
#14360=EDGE_CURVE ( 'NONE', #17588, #7360, #24533, .T. ) ;
#14367=CARTESIAN_POINT ( 'NONE',  ( -19.43607991388963896, 24.27856662945520583, 1.000000000000000000 ) ) ;
#14371=VERTEX_POINT ( 'NONE', #11063 ) ;
#14375=ORIENTED_EDGE ( 'NONE', *, *, #23354, .T. ) ;
#14380=ORIENTED_EDGE ( 'NONE', *, *, #4312, .F. ) ;
#14385=ORIENTED_EDGE ( 'NONE', *, *, #12577, .F. ) ;
#14386=( NAMED_UNIT ( * ) PLANE_ANGLE_UNIT ( ) SI_UNIT ( $, .RADIAN. ) );
#14393=CARTESIAN_POINT ( 'NONE',  ( -27.00874656207317059, -15.41874213889385459, -2.750000000000000000 ) ) ;
#14394=FACE_OUTER_BOUND ( 'NONE', #10849, .T. ) ;
#14397=DIRECTION ( 'NONE',  ( 0.000000000000000000, 0.000000000000000000, 1.000000000000000000 ) ) ;
#14401=CYLINDRICAL_SURFACE ( 'NONE', #21670, 31.10000000000000142 ) ;
#14402=CARTESIAN_POINT ( 'NONE',  ( -25.98730014090418194, 17.08421000182805471, -6.500000000000000000 ) ) ;
#14403=EDGE_CURVE ( 'NONE', #19826, #19523, #1189, .T. ) ;
#14404=VERTEX_POINT ( 'NONE', #4918 ) ;
#14407=VERTEX_POINT ( 'NONE', #19041 ) ;
#14408=ORIENTED_EDGE ( 'NONE', *, *, #11265, .T. ) ;
#14410=EDGE_LOOP ( 'NONE', ( #19704, #6153, #19054, #7801 ) ) ;
#14413=CARTESIAN_POINT ( 'NONE',  ( 0.000000000000000000, 0.000000000000000000, -6.500000000000000000 ) ) ;
#14414=EDGE_CURVE ( 'NONE', #17868, #6671, #9144, .T. ) ;
#14420=CARTESIAN_POINT ( 'NONE',  ( -23.96296185032681336, 19.82388608118453632, 1.000000000000000000 ) ) ;
#14425=CARTESIAN_POINT ( 'NONE',  ( -29.62293631110050995, -7.734255490826679846, -6.500000000000000000 ) ) ;
#14428=CARTESIAN_POINT ( 'NONE',  ( -24.27856662945521649, -19.43607991388963185, -6.500000000000000000 ) ) ;
#14431=ORIENTED_EDGE ( 'NONE', *, *, #3960, .F. ) ;
#14434=EDGE_CURVE ( 'NONE', #22312, #11375, #20482, .T. ) ;
#14437=ORIENTED_EDGE ( 'NONE', *, *, #6426, .T. ) ;
#14439=EDGE_CURVE ( 'NONE', #3560, #21567, #19141, .T. ) ;
#14440=ORIENTED_EDGE ( 'NONE', *, *, #13263, .F. ) ;
#14442=DIRECTION ( 'NONE',  ( -0.8443279255020122998, 0.5358267949790012086, 0.000000000000000000 ) ) ;
#14443=ORIENTED_EDGE ( 'NONE', *, *, #4253, .T. ) ;
#14452=AXIS2_PLACEMENT_3D ( 'NONE', #14558, #5239, #15436 ) ;
#14459=CARTESIAN_POINT ( 'NONE',  ( 23.01025686871630782, -20.92219106202058754, 1.000000000000000000 ) ) ;
#14460=VERTEX_POINT ( 'NONE', #25317 ) ;
#14466=FACE_OUTER_BOUND ( 'NONE', #17066, .T. ) ;
#14475=DIRECTION ( 'NONE',  ( -0.000000000000000000, -0.000000000000000000, 1.000000000000000000 ) ) ;
#14477=DIRECTION ( 'NONE',  ( 0.000000000000000000, 0.000000000000000000, -1.000000000000000000 ) ) ;
#14478=CARTESIAN_POINT ( 'NONE',  ( -20.92219106202016476, 23.01025686871669507, -6.500000000000000000 ) ) ;
#14479=CARTESIAN_POINT ( 'NONE',  ( 0.000000000000000000, 0.000000000000000000, -6.500000000000000000 ) ) ;
#14480=CARTESIAN_POINT ( 'NONE',  ( 0.000000000000000000, 0.000000000000000000, 1.000000000000000000 ) ) ;
#14490=ORIENTED_EDGE ( 'NONE', *, *, #3230, .T. ) ;
#14492=DIRECTION ( 'NONE',  ( 1.000000000000000000, 0.000000000000000000, 0.000000000000000000 ) ) ;
#14495=ORIENTED_EDGE ( 'NONE', *, *, #8949, .F. ) ;
#14497=ORIENTED_EDGE ( 'NONE', *, *, #18566, .T. ) ;
#14500=VERTEX_POINT ( 'NONE', #3343 ) ;
#14501=ORIENTED_EDGE ( 'NONE', *, *, #13959, .F. ) ;
#14506=DIRECTION ( 'NONE',  ( 0.000000000000000000, 0.000000000000000000, 1.000000000000000000 ) ) ;
#14508=EDGE_CURVE ( 'NONE', #9980, #16142, #19977, .T. ) ;
#14512=CARTESIAN_POINT ( 'NONE',  ( 0.000000000000000000, 0.000000000000000000, -6.500000000000000000 ) ) ;
#14513=FACE_OUTER_BOUND ( 'NONE', #24095, .T. ) ;
#14514=CARTESIAN_POINT ( 'NONE',  ( -27.00874656207317059, -15.41874213889385459, -6.500000000000000000 ) ) ;
#14518=DIRECTION ( 'NONE',  ( 0.000000000000000000, 0.000000000000000000, 1.000000000000000000 ) ) ;
#14523=VERTEX_POINT ( 'NONE', #11452 ) ;
#14530=EDGE_LOOP ( 'NONE', ( #1134, #22918, #2183, #23563 ) ) ;
#14538=DIRECTION ( 'NONE',  ( -0.000000000000000000, -0.000000000000000000, 1.000000000000000000 ) ) ;
#14541=CARTESIAN_POINT ( 'NONE',  ( -28.14012133169333651, -13.24173596767349359, 1.000000000000000000 ) ) ;
#14551=EDGE_LOOP ( 'NONE', ( #14078, #14385, #16081, #15469 ) ) ;
#14552=CARTESIAN_POINT ( 'NONE',  ( -21.28941499438242246, -22.67092431280570963, -6.500000000000000000 ) ) ;
#14553=ORIENTED_EDGE ( 'NONE', *, *, #13804, .F. ) ;
#14558=CARTESIAN_POINT ( 'NONE',  ( -30.85476721088030061, -3.897863563849544466, -6.500000000000000000 ) ) ;
#14563=DIRECTION ( 'NONE',  ( 1.000000000000000000, 0.000000000000000000, 0.000000000000000000 ) ) ;
#14566=CARTESIAN_POINT ( 'NONE',  ( 21.65113613650343538, 22.32573188046912449, -6.500000000000000000 ) ) ;
#14571=EDGE_CURVE ( 'NONE', #20492, #24486, #14988, .T. ) ;
#14574=CIRCLE ( 'NONE', #3295, 0.5000000000000011102 ) ;
#14575=AXIS2_PLACEMENT_3D ( 'NONE', #16318, #19835, #4017 ) ;
#14577=EDGE_CURVE ( 'NONE', #23624, #17423, #23326, .T. ) ;
#14581=CARTESIAN_POINT ( 'NONE',  ( 0.000000000000000000, 0.000000000000000000, 1.000000000000000000 ) ) ;
#14582=VERTEX_POINT ( 'NONE', #23870 ) ;
#14588=DIRECTION ( 'NONE',  ( 1.000000000000000000, 0.000000000000000000, 0.000000000000000000 ) ) ;
#14595=CIRCLE ( 'NONE', #10829, 0.4999999999999999445 ) ;
#14596=CARTESIAN_POINT ( 'NONE',  ( -30.54913349766215802, 5.827558883616378083, -6.500000000000000000 ) ) ;
#14599=CIRCLE ( 'NONE', #24621, 0.4999999999999998890 ) ;
#14602=ADVANCED_FACE ( 'NONE', ( #5955 ), #19808, .F. ) ;
#14604=DIRECTION ( 'NONE',  ( -0.000000000000000000, -0.000000000000000000, 1.000000000000000000 ) ) ;
#14606=AXIS2_PLACEMENT_3D ( 'NONE', #1344, #17171, #23565 ) ;
#14607=DIRECTION ( 'NONE',  ( 0.000000000000000000, 0.000000000000000000, 1.000000000000000000 ) ) ;
#14610=EDGE_CURVE ( 'NONE', #21069, #20277, #21237, .T. ) ;
#14614=EDGE_CURVE ( 'NONE', #23568, #10460, #15399, .T. ) ;
#14615=DIRECTION ( 'NONE',  ( 0.3090169943749591086, 0.9510565162951497564, 0.000000000000000000 ) ) ;
#14616=ORIENTED_EDGE ( 'NONE', *, *, #3265, .F. ) ;
#14618=CARTESIAN_POINT ( 'NONE',  ( -30.35476721088030061, -3.897863563849544466, -6.500000000000000000 ) ) ;
#14619=DIRECTION ( 'NONE',  ( 1.000000000000000000, 0.000000000000000000, 0.000000000000000000 ) ) ;
#14620=ORIENTED_EDGE ( 'NONE', *, *, #8296, .T. ) ;
#14621=DIRECTION ( 'NONE',  ( 0.7289686274214236539, 0.6845471059286760696, 0.000000000000000000 ) ) ;
#14624=CARTESIAN_POINT ( 'NONE',  ( 0.000000000000000000, 0.000000000000000000, -6.500000000000000000 ) ) ;
#14626=DIRECTION ( 'NONE',  ( -0.000000000000000000, -0.000000000000000000, 1.000000000000000000 ) ) ;
#14628=EDGE_LOOP ( 'NONE', ( #19885, #13923, #21209, #25391 ) ) ;
#14631=VERTEX_POINT ( 'NONE', #17854 ) ;
#14632=DIRECTION ( 'NONE',  ( 0.000000000000000000, 0.000000000000000000, 1.000000000000000000 ) ) ;
#14635=AXIS2_PLACEMENT_3D ( 'NONE', #13875, #3931, #1580 ) ;
#14643=DIRECTION ( 'NONE',  ( 0.8763066800438685799, 0.4817536741017063306, 0.000000000000000000 ) ) ;
#14645=DIRECTION ( 'NONE',  ( 0.000000000000000000, 0.000000000000000000, 1.000000000000000000 ) ) ;
#14649=LINE ( 'NONE', #2744, #5657 ) ;
#14652=CIRCLE ( 'NONE', #6282, 0.4999999999999996669 ) ;
#14657=LINE ( 'NONE', #18699, #9141 ) ;
#14658=ORIENTED_EDGE ( 'NONE', *, *, #21368, .F. ) ;
#14659=AXIS2_PLACEMENT_3D ( 'NONE', #272, #8240, #4438 ) ;
#14667=VERTEX_POINT ( 'NONE', #13801 ) ;
#14668=CYLINDRICAL_SURFACE ( 'NONE', #2749, 31.10000000000000142 ) ;
#14670=AXIS2_PLACEMENT_3D ( 'NONE', #18238, #320, #4368 ) ;
#14672=DIRECTION ( 'NONE',  ( -0.9921147013144768767, 0.1253332335643120576, 0.000000000000000000 ) ) ;
#14674=CARTESIAN_POINT ( 'NONE',  ( 0.000000000000000000, 0.000000000000000000, 1.000000000000000000 ) ) ;
#14675=CIRCLE ( 'NONE', #1722, 30.10000000000000142 ) ;
#14680=DIRECTION ( 'NONE',  ( 0.000000000000000000, -0.000000000000000000, 1.000000000000000000 ) ) ;
#14685=CIRCLE ( 'NONE', #6739, 31.10000000000000142 ) ;
#14691=EDGE_LOOP ( 'NONE', ( #16497, #9498, #6065, #8840 ) ) ;
#14693=EDGE_CURVE ( 'NONE', #24465, #1590, #9121, .T. ) ;
#14694=VECTOR ( 'NONE', #18618, 1000.000000000000000 ) ;
#14696=CARTESIAN_POINT ( 'NONE',  ( -31.03863125411922752, 1.952785157361987878, 1.000000000000000000 ) ) ;
#14699=ORIENTED_EDGE ( 'NONE', *, *, #330, .F. ) ;
#14701=AXIS2_PLACEMENT_3D ( 'NONE', #21083, #17029, #20958 ) ;
#14702=EDGE_CURVE ( 'NONE', #21799, #8280, #2872, .T. ) ;
#14713=AXIS2_PLACEMENT_3D ( 'NONE', #20784, #12940, #10975 ) ;
#14719=CARTESIAN_POINT ( 'NONE',  ( 0.000000000000000000, 0.000000000000000000, 1.000000000000000000 ) ) ;
#14723=VERTEX_POINT ( 'NONE', #9751 ) ;
#14725=DIRECTION ( 'NONE',  ( -0.000000000000000000, -0.000000000000000000, 1.000000000000000000 ) ) ;
#14727=ORIENTED_EDGE ( 'NONE', *, *, #2689, .T. ) ;
#14728=ORIENTED_EDGE ( 'NONE', *, *, #1001, .T. ) ;
#14729=LINE ( 'NONE', #22430, #8303 ) ;
#14730=VECTOR ( 'NONE', #15694, 1000.000000000000000 ) ;
#14740=DIRECTION ( 'NONE',  ( 0.000000000000000000, 0.000000000000000000, 1.000000000000000000 ) ) ;
#14742=AXIS2_PLACEMENT_3D ( 'NONE', #8194, #13688, #2049 ) ;
#14755=ORIENTED_EDGE ( 'NONE', *, *, #11478, .F. ) ;
#14756=DIRECTION ( 'NONE',  ( 0.000000000000000000, 0.000000000000000000, 1.000000000000000000 ) ) ;
#14759=CARTESIAN_POINT ( 'NONE',  ( 18.28012134629595309, 25.16042852506084770, -6.500000000000000000 ) ) ;
#14760=ORIENTED_EDGE ( 'NONE', *, *, #19392, .T. ) ;
#14763=AXIS2_PLACEMENT_3D ( 'NONE', #3563, #23308, #21359 ) ;
#14764=EDGE_LOOP ( 'NONE', ( #10626, #11551, #7322, #20233 ) ) ;
#14766=VERTEX_POINT ( 'NONE', #12809 ) ;
#14767=ORIENTED_EDGE ( 'NONE', *, *, #5790, .T. ) ;
#14771=DIRECTION ( 'NONE',  ( 1.000000000000000000, 0.000000000000000000, 0.000000000000000000 ) ) ;
#14778=LINE ( 'NONE', #18953, #25093 ) ;
#14782=DIRECTION ( 'NONE',  ( 0.000000000000000000, 0.000000000000000000, 1.000000000000000000 ) ) ;
#14785=DIRECTION ( 'NONE',  ( 0.9297764858882561212, 0.3681245526846659843, 0.000000000000000000 ) ) ;
#14786=CARTESIAN_POINT ( 'NONE',  ( -14.98253926456356666, -27.25313774936403988, 1.000000000000000000 ) ) ;
#14787=AXIS2_PLACEMENT_3D ( 'NONE', #8586, #24279, #22836 ) ;
#14788=DIRECTION ( 'NONE',  ( 0.000000000000000000, 0.000000000000000000, 1.000000000000000000 ) ) ;
#14789=CARTESIAN_POINT ( 'NONE',  ( -30.91344420362543843, 3.401318489841417048, 1.000000000000000000 ) ) ;
#14790=ORIENTED_EDGE ( 'NONE', *, *, #14614, .F. ) ;
#14791=DIRECTION ( 'NONE',  ( 0.000000000000000000, 0.000000000000000000, -1.000000000000000000 ) ) ;
#14793=EDGE_LOOP ( 'NONE', ( #1476, #16621, #7584, #13058 ) ) ;
#14794=ORIENTED_EDGE ( 'NONE', *, *, #5886, .T. ) ;
#14795=VERTEX_POINT ( 'NONE', #21814 ) ;
#14796=VERTEX_POINT ( 'NONE', #11601 ) ;
#14797=ORIENTED_EDGE ( 'NONE', *, *, #11052, .T. ) ;
#14798=DIRECTION ( 'NONE',  ( 0.000000000000000000, 0.000000000000000000, 1.000000000000000000 ) ) ;
#14801=EDGE_CURVE ( 'NONE', #16708, #24402, #5794, .T. ) ;
#14804=EDGE_CURVE ( 'NONE', #10376, #8478, #8299, .T. ) ;
#14812=LINE ( 'NONE', #13110, #17959 ) ;
#14814=DIRECTION ( 'NONE',  ( 0.9921147013144794302, 0.1253332335642911299, 0.000000000000000000 ) ) ;
#14815=CARTESIAN_POINT ( 'NONE',  ( 30.10000000000000142, 0.000000000000000000, -6.500000000000000000 ) ) ;
#14820=CARTESIAN_POINT ( 'NONE',  ( 0.000000000000000000, 0.000000000000000000, 1.000000000000000000 ) ) ;
#14821=VERTEX_POINT ( 'NONE', #1547 ) ;
#14826=ORIENTED_EDGE ( 'NONE', *, *, #13263, .T. ) ;
#14827=DIRECTION ( 'NONE',  ( 0.6845471059286972748, 0.7289686274214034478, 0.000000000000000000 ) ) ;
#14832=CARTESIAN_POINT ( 'NONE',  ( -29.57785765677936851, -9.610428525060582317, 1.000000000000000000 ) ) ;
#14835=EDGE_CURVE ( 'NONE', #8766, #15596, #9509, .T. ) ;
#14839=DIRECTION ( 'NONE',  ( 0.000000000000000000, 0.000000000000000000, 1.000000000000000000 ) ) ;
#14841=ADVANCED_FACE ( 'NONE', ( #13699 ), #25230, .T. ) ;
#14843=CYLINDRICAL_SURFACE ( 'NONE', #9978, 0.5000000000000004441 ) ;
#14849=AXIS2_PLACEMENT_3D ( 'NONE', #20548, #4590, #22648 ) ;
#14853=VERTEX_POINT ( 'NONE', #13321 ) ;
#14854=EDGE_LOOP ( 'NONE', ( #20245, #6848, #5144, #21214 ) ) ;
#14860=DIRECTION ( 'NONE',  ( 0.000000000000000000, 0.000000000000000000, 1.000000000000000000 ) ) ;
#14861=CIRCLE ( 'NONE', #13608, 27.10000000000000142 ) ;
#14862=CARTESIAN_POINT ( 'NONE',  ( -17.87326343783916727, 25.45105997952937926, 1.000000000000000000 ) ) ;
#14865=EDGE_CURVE ( 'NONE', #8603, #16823, #21297, .T. ) ;
#14868=FACE_OUTER_BOUND ( 'NONE', #25071, .T. ) ;
#14869=CARTESIAN_POINT ( 'NONE',  ( 0.000000000000000000, 0.000000000000000000, 1.000000000000000000 ) ) ;
#14870=CYLINDRICAL_SURFACE ( 'NONE', #20404, 0.4999999999999970024 ) ;
#14874=FACE_OUTER_BOUND ( 'NONE', #2113, .T. ) ;
#14876=LINE ( 'NONE', #16851, #1211 ) ;
#14879=ORIENTED_EDGE ( 'NONE', *, *, #6019, .F. ) ;
#14883=DIRECTION ( 'NONE',  ( 0.000000000000000000, -0.000000000000000000, 1.000000000000000000 ) ) ;
#14885=DIRECTION ( 'NONE',  ( 1.000000000000000000, 0.000000000000000000, 0.000000000000000000 ) ) ;
#14886=ORIENTED_EDGE ( 'NONE', *, *, #21031, .F. ) ;
#14890=CARTESIAN_POINT ( 'NONE',  ( 0.000000000000000000, 0.000000000000000000, -6.500000000000000000 ) ) ;
#14893=EDGE_CURVE ( 'NONE', #8412, #2690, #13270, .T. ) ;
#14898=ADVANCED_FACE ( 'NONE', ( #18027 ), #14843, .F. ) ;
#14901=UNCERTAINTY_MEASURE_WITH_UNIT (LENGTH_MEASURE( 1.000000000000000082E-05 ), #12798, 'distance_accuracy_value', 'NONE');
#14902=PRODUCT_DEFINITION_CONTEXT ( 'detailed design', #21973, 'design' ) ;
#14904=CARTESIAN_POINT ( 'NONE',  ( 29.57785765677924061, -9.610428525060996208, -6.500000000000000000 ) ) ;
#14905=LINE ( 'NONE', #13323, #22499 ) ;
#14907=EDGE_CURVE ( 'NONE', #18639, #18972, #10763, .T. ) ;
#14911=CARTESIAN_POINT ( 'NONE',  ( -28.34936733434187062, 12.78762572734087044, -2.750000000000000000 ) ) ;
#14912=CARTESIAN_POINT ( 'NONE',  ( -29.99470236596024364, 8.217531866531397000, 1.000000000000000000 ) ) ;
#14913=CARTESIAN_POINT ( 'NONE',  ( -19.32388608118446527, -23.96296185032687376, -6.500000000000000000 ) ) ;
#14914=VERTEX_POINT ( 'NONE', #8330 ) ;
#14916=DIRECTION ( 'NONE',  ( 0.7289686274214236539, 0.6845471059286760696, 0.000000000000000000 ) ) ;
#14917=CARTESIAN_POINT ( 'NONE',  ( 14.98253926456319007, -27.25313774936425304, 1.000000000000000000 ) ) ;
#14918=VERTEX_POINT ( 'NONE', #8822 ) ;
#14919=ORIENTED_EDGE ( 'NONE', *, *, #14964, .T. ) ;
#14920=EDGE_LOOP ( 'NONE', ( #552, #20720, #11135, #10202 ) ) ;
#14921=EDGE_LOOP ( 'NONE', ( #11762, #7099, #17900, #22435 ) ) ;
#14922=EDGE_LOOP ( 'NONE', ( #7638, #14797 ) ) ;
#14924=ORIENTED_EDGE ( 'NONE', *, *, #21869, .T. ) ;
#14926=FACE_OUTER_BOUND ( 'NONE', #7443, .T. ) ;
#14934=CARTESIAN_POINT ( 'NONE',  ( -16.66421332384646448, 26.25859848311288403, -6.500000000000000000 ) ) ;
#14938=CARTESIAN_POINT ( 'NONE',  ( -7.248980000273768098, 30.24338421796792176, -6.500000000000000000 ) ) ;
#14941=ADVANCED_FACE ( 'NONE', ( #12748 ), #18158, .F. ) ;
#14942=VERTEX_POINT ( 'NONE', #20718 ) ;
#14947=CARTESIAN_POINT ( 'NONE',  ( -21.28941499438192864, 22.67092431280617859, -6.500000000000000000 ) ) ;
#14948=VERTEX_POINT ( 'NONE', #10160 ) ;
#14949=DIRECTION ( 'NONE',  ( 1.000000000000000000, 0.000000000000000000, 0.000000000000000000 ) ) ;
#14950=ORIENTED_EDGE ( 'NONE', *, *, #23227, .T. ) ;
#14951=DIRECTION ( 'NONE',  ( 1.000000000000000000, 0.000000000000000000, 0.000000000000000000 ) ) ;
#14954=CARTESIAN_POINT ( 'NONE',  ( -18.28012134629558716, 25.16042852506110705, 1.000000000000000000 ) ) ;
#14955=CIRCLE ( 'NONE', #13693, 31.10000000000000142 ) ;
#14964=EDGE_CURVE ( 'NONE', #4477, #3258, #22512, .T. ) ;
#14968=EDGE_CURVE ( 'NONE', #25152, #25550, #1936, .T. ) ;
#14969=AXIS2_PLACEMENT_3D ( 'NONE', #13844, #23771, #25484 ) ;
#14970=CARTESIAN_POINT ( 'NONE',  ( 29.57785765677931167, 9.610428525060783045, -6.500000000000000000 ) ) ;
#14974=EDGE_LOOP ( 'NONE', ( #23182, #19736, #6971, #12175 ) ) ;
#14976=CARTESIAN_POINT ( 'NONE',  ( 30.78811501957141772, -4.393401135981229721, -2.750000000000000000 ) ) ;
#14978=DIRECTION ( 'NONE',  ( 0.000000000000000000, 0.000000000000000000, -1.000000000000000000 ) ) ;
#14980=VERTEX_POINT ( 'NONE', #359 ) ;
#14984=LINE ( 'NONE', #17346, #8950 ) ;
#14988=CIRCLE ( 'NONE', #23728, 31.10000000000000142 ) ;
#14991=CIRCLE ( 'NONE', #15402, 0.4999999999999992784 ) ;
#14992=CYLINDRICAL_SURFACE ( 'NONE', #5493, 0.5000000000000004441 ) ;
#14994=CIRCLE ( 'NONE', #5395, 31.10000000000000142 ) ;
#14995=LINE ( 'NONE', #8986, #17902 ) ;
#15005=DIRECTION ( 'NONE',  ( 0.000000000000000000, 0.000000000000000000, 1.000000000000000000 ) ) ;
#15008=DIRECTION ( 'NONE',  ( -0.000000000000000000, 0.000000000000000000, 1.000000000000000000 ) ) ;
#15009=ORIENTED_EDGE ( 'NONE', *, *, #2436, .T. ) ;
#15011=EDGE_CURVE ( 'NONE', #17619, #13585, #12065, .T. ) ;
#15015=ORIENTED_EDGE ( 'NONE', *, *, #10791, .T. ) ;
#15022=AXIS2_PLACEMENT_3D ( 'NONE', #4448, #6666, #22765 ) ;
#15025=CARTESIAN_POINT ( 'NONE',  ( 0.000000000000000000, 0.000000000000000000, -6.500000000000000000 ) ) ;
#15029=CIRCLE ( 'NONE', #395, 0.4999999999999997224 ) ;
#15032=CARTESIAN_POINT ( 'NONE',  ( -30.12293631110035363, 7.734255490827311341, -6.500000000000000000 ) ) ;
#15033=DIRECTION ( 'NONE',  ( -0.000000000000000000, -0.000000000000000000, 1.000000000000000000 ) ) ;
#15034=CARTESIAN_POINT ( 'NONE',  ( -29.57785765677936851, -9.610428525060582317, -6.500000000000000000 ) ) ;
#15039=CARTESIAN_POINT ( 'NONE',  ( 0.000000000000000000, 0.000000000000000000, -6.500000000000000000 ) ) ;
#15040=AXIS2_PLACEMENT_3D ( 'NONE', #15597, #1982, #11652 ) ;
#15043=ORIENTED_EDGE ( 'NONE', *, *, #13095, .F. ) ;
#15045=DIRECTION ( 'NONE',  ( -0.000000000000000000, 0.000000000000000000, -1.000000000000000000 ) ) ;
#15050=ORIENTED_EDGE ( 'NONE', *, *, #3988, .F. ) ;
#15051=VERTEX_POINT ( 'NONE', #17440 ) ;
#15052=EDGE_LOOP ( 'NONE', ( #1663, #19661, #13182, #3814 ) ) ;
#15055=DIRECTION ( 'NONE',  ( -0.000000000000000000, 0.000000000000000000, 1.000000000000000000 ) ) ;
#15057=AXIS2_PLACEMENT_3D ( 'NONE', #14239, #22599, #14619 ) ;
#15061=AXIS2_PLACEMENT_3D ( 'NONE', #5186, #1251, #13162 ) ;
#15070=DIRECTION ( 'NONE',  ( 0.000000000000000000, 0.000000000000000000, 1.000000000000000000 ) ) ;
#15072=CARTESIAN_POINT ( 'NONE',  ( 0.000000000000000000, 0.000000000000000000, -6.500000000000000000 ) ) ;
#15073=LINE ( 'NONE', #14815, #23424 ) ;
#15075=AXIS2_PLACEMENT_3D ( 'NONE', #7628, #13905, #11668 ) ;
#15076=DIRECTION ( 'NONE',  ( 0.06279051952930848890, -0.9980267284282718920, 0.000000000000000000 ) ) ;
#15078=EDGE_CURVE ( 'NONE', #3783, #14500, #12472, .T. ) ;
#15079=ORIENTED_EDGE ( 'NONE', *, *, #18724, .T. ) ;
#15081=CARTESIAN_POINT ( 'NONE',  ( -1.952785157361865753, -31.03863125411923463, -6.500000000000000000 ) ) ;
#15082=EDGE_LOOP ( 'NONE', ( #372, #12912, #8608, #13375 ) ) ;
#15086=EDGE_CURVE ( 'NONE', #24580, #9729, #24595, .T. ) ;
#15087=ORIENTED_EDGE ( 'NONE', *, *, #5330, .F. ) ;
#15089=ADVANCED_FACE ( 'NONE', ( #11287 ), #24905, .T. ) ;
#15092=VECTOR ( 'NONE', #9405, 1000.000000000000000 ) ;
#15093=AXIS2_PLACEMENT_3D ( 'NONE', #8791, #693, #3040 ) ;
#15094=CYLINDRICAL_SURFACE ( 'NONE', #7165, 0.5000000000000004441 ) ;
#15095=DIRECTION ( 'NONE',  ( -0.000000000000000000, -0.000000000000000000, -1.000000000000000000 ) ) ;
#15097=ADVANCED_FACE ( 'NONE', ( #9074 ), #21371, .F. ) ;
#15098=AXIS2_PLACEMENT_3D ( 'NONE', #11176, #23222, #1254 ) ;
#15100=FACE_OUTER_BOUND ( 'NONE', #16894, .T. ) ;
#15104=AXIS2_PLACEMENT_3D ( 'NONE', #2673, #6333, #6714 ) ;
#15105=ORIENTED_EDGE ( 'NONE', *, *, #14577, .F. ) ;
#15106=VERTEX_POINT ( 'NONE', #12868 ) ;
#15110=AXIS2_PLACEMENT_3D ( 'NONE', #7359, #21215, #9711 ) ;
#15114=CARTESIAN_POINT ( 'NONE',  ( -25.98730014090454432, -17.08421000182750760, -6.500000000000000000 ) ) ;
#15118=DIRECTION ( 'NONE',  ( 1.000000000000000000, 0.000000000000000000, 0.000000000000000000 ) ) ;
#15119=AXIS2_PLACEMENT_3D ( 'NONE', #11359, #3765, #1432 ) ;
#15120=CYLINDRICAL_SURFACE ( 'NONE', #17172, 31.10000000000000142 ) ;
#15121=VERTEX_POINT ( 'NONE', #17326 ) ;
#15128=EDGE_CURVE ( 'NONE', #4507, #3917, #8735, .T. ) ;
#15129=CIRCLE ( 'NONE', #3007, 0.5000000000000004441 ) ;
#15130=EDGE_CURVE ( 'NONE', #18321, #20266, #20796, .T. ) ;
#15131=AXIS2_PLACEMENT_3D ( 'NONE', #11604, #23766, #25478 ) ;
#15132=DIRECTION ( 'NONE',  ( -0.000000000000000000, -0.000000000000000000, 1.000000000000000000 ) ) ;
#15135=CARTESIAN_POINT ( 'NONE',  ( 17.08421000182759997, -25.98730014090448392, 1.000000000000000000 ) ) ;
#15136=EDGE_CURVE ( 'NONE', #7090, #14766, #19014, .T. ) ;
#15144=DIRECTION ( 'NONE',  ( 0.5358267949790093132, 0.8443279255020070817, 0.000000000000000000 ) ) ;
#15155=CIRCLE ( 'NONE', #24737, 31.10000000000000142 ) ;
#15159=VERTEX_POINT ( 'NONE', #10897 ) ;
#15164=AXIS2_PLACEMENT_3D ( 'NONE', #22612, #6908, #24832 ) ;
#15167=DIRECTION ( 'NONE',  ( 1.000000000000000000, 0.000000000000000000, 0.000000000000000000 ) ) ;
#15177=CARTESIAN_POINT ( 'NONE',  ( -1.452785157361201396, 31.03863125411927371, -6.500000000000000000 ) ) ;
#15178=EDGE_CURVE ( 'NONE', #21381, #14795, #15828, .T. ) ;
#15181=ORIENTED_EDGE ( 'NONE', *, *, #11148, .T. ) ;
#15183=CARTESIAN_POINT ( 'NONE',  ( 0.000000000000000000, 0.000000000000000000, -6.500000000000000000 ) ) ;
#15186=ORIENTED_EDGE ( 'NONE', *, *, #10791, .F. ) ;
#15187=ORIENTED_EDGE ( 'NONE', *, *, #18629, .F. ) ;
#15191=DIRECTION ( 'NONE',  ( 0.000000000000000000, 0.000000000000000000, 1.000000000000000000 ) ) ;
#15201=DIRECTION ( 'NONE',  ( 0.000000000000000000, 0.000000000000000000, 1.000000000000000000 ) ) ;
#15203=DIRECTION ( 'NONE',  ( 0.1253332335642980688, -0.9921147013144785420, 0.000000000000000000 ) ) ;
#15208=ORIENTED_EDGE ( 'NONE', *, *, #20352, .T. ) ;
#15210=ORIENTED_EDGE ( 'NONE', *, *, #20211, .T. ) ;
#15211=EDGE_CURVE ( 'NONE', #10594, #20500, #4549, .T. ) ;
#15212=VERTEX_POINT ( 'NONE', #3695 ) ;
#15218=ORIENTED_EDGE ( 'NONE', *, *, #25505, .F. ) ;
#15221=DIRECTION ( 'NONE',  ( -0.000000000000000000, -0.000000000000000000, 1.000000000000000000 ) ) ;
#15222=CARTESIAN_POINT ( 'NONE',  ( 28.34936733434196299, -12.78762572734067149, 1.000000000000000000 ) ) ;
#15225=FACE_OUTER_BOUND ( 'NONE', #6127, .T. ) ;
#15226=PRODUCT_DEFINITION_FORMATION_WITH_SPECIFIED_SOURCE ( 'ANY', '', #8177, .NOT_KNOWN. ) ;
#15228=ADVANCED_FACE ( 'NONE', ( #21882 ), #19786, .F. ) ;
#15231=ORIENTED_EDGE ( 'NONE', *, *, #12704, .T. ) ;
#15233=EDGE_CURVE ( 'NONE', #19968, #13187, #20037, .T. ) ;
#15237=DIRECTION ( 'NONE',  ( 1.000000000000000000, 0.000000000000000000, 0.000000000000000000 ) ) ;
#15241=ORIENTED_EDGE ( 'NONE', *, *, #11269, .F. ) ;
#15242=ORIENTED_EDGE ( 'NONE', *, *, #907, .T. ) ;
#15243=CARTESIAN_POINT ( 'NONE',  ( 27.00874656207304980, 15.41874213889405176, -2.750000000000000000 ) ) ;
#15245=VERTEX_POINT ( 'NONE', #17962 ) ;
#15248=DIRECTION ( 'NONE',  ( 0.000000000000000000, 0.000000000000000000, 1.000000000000000000 ) ) ;
#15256=VECTOR ( 'NONE', #24430, 1000.000000000000000 ) ;
#15265=EDGE_LOOP ( 'NONE', ( #16009, #791, #5998, #9291 ) ) ;
#15269=EDGE_CURVE ( 'NONE', #11648, #21178, #6055, .T. ) ;
#15274=EDGE_CURVE ( 'NONE', #11788, #21799, #4133, .T. ) ;
#15277=ORIENTED_EDGE ( 'NONE', *, *, #24207, .F. ) ;
#15282=CYLINDRICAL_SURFACE ( 'NONE', #6361, 0.5000000000000004441 ) ;
#15283=LINE ( 'NONE', #5337, #21346 ) ;
#15284=CARTESIAN_POINT ( 'NONE',  ( 6.317933499823219279, -30.45149776762731975, -2.750000000000000000 ) ) ;
#15285=CIRCLE ( 'NONE', #4831, 0.5000000000000011102 ) ;
#15288=CARTESIAN_POINT ( 'NONE',  ( -25.16042852506064165, 18.28012134629622309, -6.500000000000000000 ) ) ;
#15292=DIRECTION ( 'NONE',  ( -0.4817536741017063306, 0.8763066800438685799, 0.000000000000000000 ) ) ;
#15293=CARTESIAN_POINT ( 'NONE',  ( -23.96296185032681336, 19.82388608118453632, -6.500000000000000000 ) ) ;
#15298=ORIENTED_EDGE ( 'NONE', *, *, #15604, .F. ) ;
#15299=DIRECTION ( 'NONE',  ( -0.000000000000000000, 0.000000000000000000, 1.000000000000000000 ) ) ;
#15301=FACE_OUTER_BOUND ( 'NONE', #448, .T. ) ;
#15302=EDGE_LOOP ( 'NONE', ( #20176, #10229, #20855, #5792 ) ) ;
#15305=ORIENTED_EDGE ( 'NONE', *, *, #4493, .T. ) ;
#15306=ORIENTED_EDGE ( 'NONE', *, *, #8109, .F. ) ;
#15308=FACE_OUTER_BOUND ( 'NONE', #722, .T. ) ;
#15315=FACE_OUTER_BOUND ( 'NONE', #11582, .T. ) ;
#15316=CARTESIAN_POINT ( 'NONE',  ( -11.91206721063010754, 28.72825533807145959, -6.500000000000000000 ) ) ;
#15318=DIRECTION ( 'NONE',  ( 0.000000000000000000, 0.000000000000000000, 1.000000000000000000 ) ) ;
#15319=CARTESIAN_POINT ( 'NONE',  ( -16.16421332384701515, -26.25859848311253941, -6.500000000000000000 ) ) ;
#15326=ORIENTED_EDGE ( 'NONE', *, *, #13164, .T. ) ;
#15328=ORIENTED_EDGE ( 'NONE', *, *, #18531, .F. ) ;
#15331=DIRECTION ( 'NONE',  ( 1.000000000000000000, 0.000000000000000000, 0.000000000000000000 ) ) ;
#15335=CARTESIAN_POINT ( 'NONE',  ( -26.25859848311247902, 16.66421332384710752, -6.500000000000000000 ) ) ;
#15336=EDGE_CURVE ( 'NONE', #8603, #19269, #13332, .T. ) ;
#15337=ORIENTED_EDGE ( 'NONE', *, *, #11231, .F. ) ;
#15344=FACE_OUTER_BOUND ( 'NONE', #24884, .T. ) ;
#15351=DIRECTION ( 'NONE',  ( 0.000000000000000000, 0.000000000000000000, 1.000000000000000000 ) ) ;
#15353=CYLINDRICAL_SURFACE ( 'NONE', #1232, 31.10000000000000142 ) ;
#15356=ORIENTED_EDGE ( 'NONE', *, *, #13506, .F. ) ;
#15358=DIRECTION ( 'NONE',  ( 1.000000000000000000, 0.000000000000000000, 0.000000000000000000 ) ) ;
#15361=DIRECTION ( 'NONE',  ( -0.000000000000000000, 0.000000000000000000, 1.000000000000000000 ) ) ;
#15362=ORIENTED_EDGE ( 'NONE', *, *, #13846, .F. ) ;
#15364=DIRECTION ( 'NONE',  ( 0.000000000000000000, -0.000000000000000000, 1.000000000000000000 ) ) ;
#15368=DIRECTION ( 'NONE',  ( 1.000000000000000000, 0.000000000000000000, 0.000000000000000000 ) ) ;
#15371=ADVANCED_FACE ( 'NONE', ( #18723 ), #10343, .T. ) ;
#15383=DIRECTION ( 'NONE',  ( -0.000000000000000000, 0.000000000000000000, 1.000000000000000000 ) ) ;
#15384=ORIENTED_EDGE ( 'NONE', *, *, #12733, .F. ) ;
#15387=EDGE_CURVE ( 'NONE', #10075, #11934, #2775, .T. ) ;
#15392=ORIENTED_EDGE ( 'NONE', *, *, #19751, .T. ) ;
#15396=DIRECTION ( 'NONE',  ( 0.000000000000000000, 0.000000000000000000, 1.000000000000000000 ) ) ;
#15399=CIRCLE ( 'NONE', #4520, 31.10000000000000142 ) ;
#15402=AXIS2_PLACEMENT_3D ( 'NONE', #2844, #12669, #6902 ) ;
#15403=AXIS2_PLACEMENT_3D ( 'NONE', #23294, #1588, #4777 ) ;
#15406=ADVANCED_FACE ( 'NONE', ( #14163 ), #20169, .F. ) ;
#15407=FACE_OUTER_BOUND ( 'NONE', #9261, .T. ) ;
#15410=DIRECTION ( 'NONE',  ( 0.000000000000000000, -0.000000000000000000, 1.000000000000000000 ) ) ;
#15418=DIRECTION ( 'NONE',  ( 0.000000000000000000, 0.000000000000000000, 1.000000000000000000 ) ) ;
#15420=DIRECTION ( 'NONE',  ( 1.000000000000000000, 0.000000000000000000, 0.000000000000000000 ) ) ;
#15422=CIRCLE ( 'NONE', #25430, 0.5000000000000007772 ) ;
#15424=AXIS2_PLACEMENT_3D ( 'NONE', #23840, #1998, #5544 ) ;
#15425=ORIENTED_EDGE ( 'NONE', *, *, #23557, .F. ) ;
#15426=CARTESIAN_POINT ( 'NONE',  ( -3.397863563850083146, -30.85476721088024021, -6.500000000000000000 ) ) ;
#15427=CARTESIAN_POINT ( 'NONE',  ( -20.20656826142300133, -23.64116323484216053, -2.750000000000000000 ) ) ;
#15428=DIRECTION ( 'NONE',  ( 0.000000000000000000, 0.000000000000000000, 1.000000000000000000 ) ) ;
#15429=ORIENTED_EDGE ( 'NONE', *, *, #13144, .F. ) ;
#15431=AXIS2_PLACEMENT_3D ( 'NONE', #24194, #14275, #9819 ) ;
#15432=ORIENTED_EDGE ( 'NONE', *, *, #2294, .F. ) ;
#15435=DIRECTION ( 'NONE',  ( 0.000000000000000000, 0.000000000000000000, 1.000000000000000000 ) ) ;
#15436=DIRECTION ( 'NONE',  ( -0.1253332335642912687, 0.9921147013144795412, 0.000000000000000000 ) ) ;
#15438=VECTOR ( 'NONE', #14477, 1000.000000000000000 ) ;
#15439=CIRCLE ( 'NONE', #6247, 31.10000000000000142 ) ;
#15444=CIRCLE ( 'NONE', #5814, 0.4999999999999999445 ) ;
#15445=ADVANCED_FACE ( 'NONE', ( #18344 ), #4754, .F. ) ;
#15451=CARTESIAN_POINT ( 'NONE',  ( 10.08469938919477649, -29.41953157733097868, 1.000000000000000000 ) ) ;
#15453=CARTESIAN_POINT ( 'NONE',  ( 0.000000000000000000, 0.000000000000000000, -6.500000000000000000 ) ) ;
#15457=CARTESIAN_POINT ( 'NONE',  ( 0.000000000000000000, 0.000000000000000000, -6.500000000000000000 ) ) ;
#15461=ORIENTED_EDGE ( 'NONE', *, *, #7545, .F. ) ;
#15462=CARTESIAN_POINT ( 'NONE',  ( 22.32573188046920265, 21.65113613650335367, 1.000000000000000000 ) ) ;
#15464=AXIS2_PLACEMENT_3D ( 'NONE', #11953, #8050, #17851 ) ;
#15467=ORIENTED_EDGE ( 'NONE', *, *, #9613, .T. ) ;
#15469=ORIENTED_EDGE ( 'NONE', *, *, #20875, .T. ) ;
#15471=CIRCLE ( 'NONE', #840, 27.10000000000000142 ) ;
#15474=DIRECTION ( 'NONE',  ( 1.000000000000000000, 0.000000000000000000, 0.000000000000000000 ) ) ;
#15480=VECTOR ( 'NONE', #4316, 1000.000000000000000 ) ;
#15482=EDGE_CURVE ( 'NONE', #16373, #3186, #2852, .T. ) ;
#15487=CARTESIAN_POINT ( 'NONE',  ( 0.000000000000000000, 0.000000000000000000, -6.500000000000000000 ) ) ;
#15488=ORIENTED_EDGE ( 'NONE', *, *, #15761, .T. ) ;
#15494=CARTESIAN_POINT ( 'NONE',  ( 0.000000000000000000, 0.000000000000000000, -6.500000000000000000 ) ) ;
#15498=ORIENTED_EDGE ( 'NONE', *, *, #14019, .T. ) ;
#15500=AXIS2_PLACEMENT_3D ( 'NONE', #5064, #19167, #5311 ) ;
#15502=CARTESIAN_POINT ( 'NONE',  ( 28.14012133169314822, -13.24173596767388794, -6.500000000000000000 ) ) ;
#15503=VERTEX_POINT ( 'NONE', #11131 ) ;
#15504=AXIS2_PLACEMENT_3D ( 'NONE', #2045, #19942, #22309 ) ;
#15509=CARTESIAN_POINT ( 'NONE',  ( -0.4999838450259764255, -31.09598070739550124, -6.500000000000000000 ) ) ;
#15511=VECTOR ( 'NONE', #17187, 1000.000000000000000 ) ;
#15513=DIRECTION ( 'NONE',  ( 0.000000000000000000, 0.000000000000000000, 1.000000000000000000 ) ) ;
#15514=CIRCLE ( 'NONE', #6751, 31.10000000000000142 ) ;
#15515=CIRCLE ( 'NONE', #4232, 31.10000000000000142 ) ;
#15516=CARTESIAN_POINT ( 'NONE',  ( -28.41604871112448549, 11.44867358849382910, -6.500000000000000000 ) ) ;
#15518=ADVANCED_FACE ( 'NONE', ( #17032 ), #5255, .F. ) ;
#15519=CARTESIAN_POINT ( 'NONE',  ( 0.000000000000000000, 0.000000000000000000, 1.000000000000000000 ) ) ;
#15522=DIRECTION ( 'NONE',  ( 0.000000000000000000, 0.000000000000000000, 1.000000000000000000 ) ) ;
#15524=VECTOR ( 'NONE', #14088, 1000.000000000000000 ) ;
#15525=DIRECTION ( 'NONE',  ( 0.000000000000000000, 0.000000000000000000, 1.000000000000000000 ) ) ;
#15528=ORIENTED_EDGE ( 'NONE', *, *, #21124, .T. ) ;
#15532=ORIENTED_EDGE ( 'NONE', *, *, #9750, .F. ) ;
#15534=DIRECTION ( 'NONE',  ( -0.000000000000000000, -0.000000000000000000, 1.000000000000000000 ) ) ;
#15543=CIRCLE ( 'NONE', #23468, 0.5000000000000003331 ) ;
#15545=CARTESIAN_POINT ( 'NONE',  ( 25.98730014090430274, -17.08421000182786997, -6.500000000000000000 ) ) ;
#15550=CARTESIAN_POINT ( 'NONE',  ( 0.000000000000000000, 0.000000000000000000, -6.500000000000000000 ) ) ;
#15552=CARTESIAN_POINT ( 'NONE',  ( -27.25313774936430633, -14.98253926456308172, -6.500000000000000000 ) ) ;
#15553=ORIENTED_EDGE ( 'NONE', *, *, #10098, .T. ) ;
#15555=CARTESIAN_POINT ( 'NONE',  ( -30.54913349766228592, -5.827558883615738594, 1.000000000000000000 ) ) ;
#15557=AXIS2_PLACEMENT_3D ( 'NONE', #9135, #11217, #24711 ) ;
#15559=ADVANCED_FACE ( 'NONE', ( #10869 ), #6959, .F. ) ;
#15562=VERTEX_POINT ( 'NONE', #14938 ) ;
#15563=DIRECTION ( 'NONE',  ( 0.4257792915650852050, 0.9048270524660135816, 0.000000000000000000 ) ) ;
#15566=EDGE_CURVE ( 'NONE', #8668, #10289, #14955, .T. ) ;
#15568=ORIENTED_EDGE ( 'NONE', *, *, #9060, .F. ) ;
#15572=DIRECTION ( 'NONE',  ( 0.000000000000000000, 0.000000000000000000, 1.000000000000000000 ) ) ;
#15574=CARTESIAN_POINT ( 'NONE',  ( -23.64116323484217830, 20.20656826142297646, 1.000000000000000000 ) ) ;
#15576=VECTOR ( 'NONE', #16613, 1000.000000000000000 ) ;
#15583=FACE_OUTER_BOUND ( 'NONE', #22528, .T. ) ;
#15585=DIRECTION ( 'NONE',  ( 1.000000000000000000, 0.000000000000000000, 0.000000000000000000 ) ) ;
#15586=LINE ( 'NONE', #21082, #18725 ) ;
#15587=CYLINDRICAL_SURFACE ( 'NONE', #19727, 0.5000000000000004441 ) ;
#15590=CARTESIAN_POINT ( 'NONE',  ( 0.000000000000000000, 0.000000000000000000, -6.500000000000000000 ) ) ;
#15591=CARTESIAN_POINT ( 'NONE',  ( 20.92219106202033529, -23.01025686871653875, -6.500000000000000000 ) ) ;
#15593=ORIENTED_EDGE ( 'NONE', *, *, #3064, .T. ) ;
#15596=VERTEX_POINT ( 'NONE', #12979 ) ;
#15597=CARTESIAN_POINT ( 'NONE',  ( 0.000000000000000000, 0.000000000000000000, 1.000000000000000000 ) ) ;
#15604=EDGE_CURVE ( 'NONE', #23080, #9004, #18715, .T. ) ;
#15606=ORIENTED_EDGE ( 'NONE', *, *, #21894, .F. ) ;
#15608=EDGE_CURVE ( 'NONE', #2274, #13061, #16203, .T. ) ;
#15610=AXIS2_PLACEMENT_3D ( 'NONE', #1088, #19983, #16347 ) ;
#15611=DIRECTION ( 'NONE',  ( 1.000000000000000000, 0.000000000000000000, 0.000000000000000000 ) ) ;
#15612=DIRECTION ( 'NONE',  ( 0.000000000000000000, 0.000000000000000000, 1.000000000000000000 ) ) ;
#15621=ORIENTED_EDGE ( 'NONE', *, *, #15608, .F. ) ;
#15623=AXIS2_PLACEMENT_3D ( 'NONE', #9362, #999, #7000 ) ;
#15624=VERTEX_POINT ( 'NONE', #8794 ) ;
#15625=CARTESIAN_POINT ( 'NONE',  ( 13.69242354489141711, 27.92360179968378375, 1.000000000000000000 ) ) ;
#15629=ORIENTED_EDGE ( 'NONE', *, *, #14968, .T. ) ;
#15631=EDGE_CURVE ( 'NONE', #2787, #6210, #13115, .T. ) ;
#15633=ORIENTED_EDGE ( 'NONE', *, *, #24924, .T. ) ;
#15634=CARTESIAN_POINT ( 'NONE',  ( 0.000000000000000000, 0.000000000000000000, -6.500000000000000000 ) ) ;
#15635=LINE ( 'NONE', #3852, #5531 ) ;
#15642=CARTESIAN_POINT ( 'NONE',  ( 3.897863563849651936, -30.85476721088028640, 1.000000000000000000 ) ) ;
#15650=CARTESIAN_POINT ( 'NONE',  ( 0.000000000000000000, 0.000000000000000000, -6.500000000000000000 ) ) ;
#15657=DIRECTION ( 'NONE',  ( -0.000000000000000000, -0.000000000000000000, 1.000000000000000000 ) ) ;
#15662=CYLINDRICAL_SURFACE ( 'NONE', #22162, 31.10000000000000142 ) ;
#15665=LINE ( 'NONE', #23632, #4705 ) ;
#15674=DIRECTION ( 'NONE',  ( 0.000000000000000000, 0.000000000000000000, 1.000000000000000000 ) ) ;
#15682=CARTESIAN_POINT ( 'NONE',  ( 0.000000000000000000, 0.000000000000000000, 1.000000000000000000 ) ) ;
#15685=DIRECTION ( 'NONE',  ( 1.000000000000000000, 0.000000000000000000, 0.000000000000000000 ) ) ;
#15686=CARTESIAN_POINT ( 'NONE',  ( 0.000000000000000000, 0.000000000000000000, -6.500000000000000000 ) ) ;
#15687=CARTESIAN_POINT ( 'NONE',  ( -23.96296185032722548, -19.82388608118403539, -6.500000000000000000 ) ) ;
#15694=DIRECTION ( 'NONE',  ( 0.000000000000000000, -0.000000000000000000, 1.000000000000000000 ) ) ;
#15695=FACE_OUTER_BOUND ( 'NONE', #3052, .T. ) ;
#15696=EDGE_CURVE ( 'NONE', #10041, #12524, #21339, .T. ) ;
#15698=DIRECTION ( 'NONE',  ( 0.6845471059286972748, 0.7289686274214034478, 0.000000000000000000 ) ) ;
#15699=EDGE_CURVE ( 'NONE', #10594, #6260, #24977, .T. ) ;
#15700=AXIS2_PLACEMENT_3D ( 'NONE', #24104, #22282, #6187 ) ;
#15703=DIRECTION ( 'NONE',  ( 0.000000000000000000, 0.000000000000000000, 1.000000000000000000 ) ) ;
#15706=DIRECTION ( 'NONE',  ( -0.06279051952930156388, 0.9980267284282724471, 0.000000000000000000 ) ) ;
#15707=CARTESIAN_POINT ( 'NONE',  ( 23.64116323484224225, -20.20656826142291251, -2.750000000000000000 ) ) ;
#15709=DIRECTION ( 'NONE',  ( 0.000000000000000000, 0.000000000000000000, 1.000000000000000000 ) ) ;
#15711=EDGE_CURVE ( 'NONE', #19766, #3578, #23713, .T. ) ;
#15715=CARTESIAN_POINT ( 'NONE',  ( 0.000000000000000000, 0.000000000000000000, -6.500000000000000000 ) ) ;
#15716=CARTESIAN_POINT ( 'NONE',  ( 15.41874213889396117, -27.00874656207311020, -6.500000000000000000 ) ) ;
#15719=DIRECTION ( 'NONE',  ( -0.000000000000000000, 0.000000000000000000, 1.000000000000000000 ) ) ;
#15725=ORIENTED_EDGE ( 'NONE', *, *, #25543, .T. ) ;
#15726=CARTESIAN_POINT ( 'NONE',  ( 1.952785157361432100, -31.03863125411925949, -6.500000000000000000 ) ) ;
#15727=ORIENTED_EDGE ( 'NONE', *, *, #17721, .T. ) ;
#15737=ADVANCED_FACE ( 'NONE', ( #21855 ), #23943, .F. ) ;
#15739=EDGE_CURVE ( 'NONE', #9082, #4731, #17418, .T. ) ;
#15743=EDGE_LOOP ( 'NONE', ( #5763, #7923, #10813, #13655 ) ) ;
#15745=ORIENTED_EDGE ( 'NONE', *, *, #25866, .F. ) ;
#15746=CARTESIAN_POINT ( 'NONE',  ( -11.91206721063072393, -28.72825533807120735, -6.500000000000000000 ) ) ;
#15748=CARTESIAN_POINT ( 'NONE',  ( -11.91206721063010754, 28.72825533807145959, 1.000000000000000000 ) ) ;
#15753=CYLINDRICAL_SURFACE ( 'NONE', #3465, 0.5000000000000004441 ) ;
#15756=CARTESIAN_POINT ( 'NONE',  ( -21.28941499438242246, -22.67092431280570963, -6.500000000000000000 ) ) ;
#15758=EDGE_CURVE ( 'NONE', #24490, #10388, #22889, .T. ) ;
#15760=FACE_OUTER_BOUND ( 'NONE', #11759, .T. ) ;
#15761=EDGE_CURVE ( 'NONE', #13301, #8478, #12023, .T. ) ;
#15766=CARTESIAN_POINT ( 'NONE',  ( 24.86329371854761661, -18.68225429291740625, -6.500000000000000000 ) ) ;
#15769=CARTESIAN_POINT ( 'NONE',  ( 27.92360179968367362, -13.69242354489162850, -6.500000000000000000 ) ) ;
#15776=CARTESIAN_POINT ( 'NONE',  ( -4.393401135981204852, -30.78811501957142127, 1.000000000000000000 ) ) ;
#15777=CARTESIAN_POINT ( 'NONE',  ( 0.000000000000000000, 0.000000000000000000, -6.500000000000000000 ) ) ;
#15778=DIRECTION ( 'NONE',  ( 0.5358267949789962126, -0.8443279255020154084, 0.000000000000000000 ) ) ;
#15780=ORIENTED_EDGE ( 'NONE', *, *, #2766, .F. ) ;
#15787=EDGE_CURVE ( 'NONE', #19787, #8351, #7850, .T. ) ;
#15790=DIRECTION ( 'NONE',  ( 1.000000000000000000, 0.000000000000000000, 0.000000000000000000 ) ) ;
#15791=DIRECTION ( 'NONE',  ( -0.000000000000000000, -0.000000000000000000, 1.000000000000000000 ) ) ;
#15792=AXIS2_PLACEMENT_3D ( 'NONE', #9310, #17028, #21582 ) ;
#15797=EDGE_LOOP ( 'NONE', ( #1204, #13898, #13258, #17009 ) ) ;
#15803=CARTESIAN_POINT ( 'NONE',  ( -31.09598070739550124, 0.4999838450261748779, 1.000000000000000000 ) ) ;
#15805=ORIENTED_EDGE ( 'NONE', *, *, #23366, .F. ) ;
#15807=DIRECTION ( 'NONE',  ( 0.9980267284282724471, 0.06279051952930156388, 0.000000000000000000 ) ) ;
#15808=FACE_OUTER_BOUND ( 'NONE', #19015, .T. ) ;
#15809=ORIENTED_EDGE ( 'NONE', *, *, #18852, .T. ) ;
#15810=ADVANCED_FACE ( 'NONE', ( #9556, #5755 ), #3805, .F. ) ;
#15811=VERTEX_POINT ( 'NONE', #11785 ) ;
#15812=CIRCLE ( 'NONE', #7031, 31.10000000000000142 ) ;
#15814=ORIENTED_EDGE ( 'NONE', *, *, #239, .T. ) ;
#15815=AXIS2_PLACEMENT_3D ( 'NONE', #11319, #19299, #19540 ) ;
#15818=LINE ( 'NONE', #19600, #20715 ) ;
#15825=CARTESIAN_POINT ( 'NONE',  ( 29.41953157733093960, 10.08469938919488484, 1.000000000000000000 ) ) ;
#15828=CIRCLE ( 'NONE', #22033, 31.10000000000000142 ) ;
#15834=DIRECTION ( 'NONE',  ( -0.9685831611286283005, 0.2486898871648657861, 0.000000000000000000 ) ) ;
#15836=VECTOR ( 'NONE', #6626, 1000.000000000000000 ) ;
#15838=CARTESIAN_POINT ( 'NONE',  ( 28.14012133169324414, 13.24173596767369254, -6.500000000000000000 ) ) ;
#15840=DIRECTION ( 'NONE',  ( 0.000000000000000000, -0.000000000000000000, 1.000000000000000000 ) ) ;
#15842=EDGE_CURVE ( 'NONE', #6572, #17588, #12441, .T. ) ;
#15845=ORIENTED_EDGE ( 'NONE', *, *, #9378, .T. ) ;
#15846=ADVANCED_FACE ( 'NONE', ( #3547 ), #21587, .T. ) ;
#15849=DIRECTION ( 'NONE',  ( -0.000000000000000000, 0.000000000000000000, 1.000000000000000000 ) ) ;
#15850=AXIS2_PLACEMENT_3D ( 'NONE', #24547, #10419, #6389 ) ;
#15851=VERTEX_POINT ( 'NONE', #11520 ) ;
#15852=EDGE_CURVE ( 'NONE', #17935, #18582, #9940, .T. ) ;
#15853=CARTESIAN_POINT ( 'NONE',  ( -20.20656826142249685, 23.64116323484259752, 1.000000000000000000 ) ) ;
#15855=CIRCLE ( 'NONE', #12085, 31.10000000000000142 ) ;
#15856=AXIS2_PLACEMENT_3D ( 'NONE', #14970, #4898, #17205 ) ;
#15868=DIRECTION ( 'NONE',  ( 0.000000000000000000, -0.000000000000000000, 1.000000000000000000 ) ) ;
#15869=ORIENTED_EDGE ( 'NONE', *, *, #16767, .T. ) ;
#15870=VERTEX_POINT ( 'NONE', #18193 ) ;
#15873=EDGE_CURVE ( 'NONE', #14980, #5929, #6186, .T. ) ;
#15875=DIRECTION ( 'NONE',  ( 0.9685831611286337406, 0.2486898871648445808, 0.000000000000000000 ) ) ;
#15879=VERTEX_POINT ( 'NONE', #10317 ) ;
#15883=AXIS2_PLACEMENT_3D ( 'NONE', #3844, #13922, #7641 ) ;
#15884=VERTEX_POINT ( 'NONE', #12551 ) ;
#15889=VECTOR ( 'NONE', #1018, 1000.000000000000000 ) ;
#15890=CARTESIAN_POINT ( 'NONE',  ( -18.28012134629558716, 25.16042852506110705, -6.500000000000000000 ) ) ;
#15895=DIRECTION ( 'NONE',  ( 1.000000000000000000, 0.000000000000000000, 0.000000000000000000 ) ) ;
#15897=DIRECTION ( 'NONE',  ( 1.000000000000000000, 0.000000000000000000, 0.000000000000000000 ) ) ;
#15902=AXIS2_PLACEMENT_3D ( 'NONE', #16358, #2476, #16216 ) ;
#15903=DIRECTION ( 'NONE',  ( 1.000000000000000000, 0.000000000000000000, 0.000000000000000000 ) ) ;
#15904=AXIS2_PLACEMENT_3D ( 'NONE', #24478, #10728, #8145 ) ;
#15905=CARTESIAN_POINT ( 'NONE',  ( 17.87326343783943017, 25.45105997952919097, -6.500000000000000000 ) ) ;
#15911=CIRCLE ( 'NONE', #21344, 31.10000000000000142 ) ;
#15913=CIRCLE ( 'NONE', #18408, 0.5000000000000002220 ) ;
#15914=PLANE ( 'NONE',  #23888 ) ;
#15915=DIRECTION ( 'NONE',  ( 0.000000000000000000, 0.000000000000000000, 1.000000000000000000 ) ) ;
#15916=CARTESIAN_POINT ( 'NONE',  ( 26.25859848311271705, 16.66421332384673804, -6.500000000000000000 ) ) ;
#15921=EDGE_CURVE ( 'NONE', #13306, #21660, #16241, .T. ) ;
#15922=CIRCLE ( 'NONE', #20966, 0.4999999999999998890 ) ;
#15927=DIRECTION ( 'NONE',  ( -0.000000000000000000, -0.000000000000000000, 1.000000000000000000 ) ) ;
#15929=AXIS2_PLACEMENT_3D ( 'NONE', #11450, #11061, #19421 ) ;
#15932=CARTESIAN_POINT ( 'NONE',  ( 22.67092431280594056, 21.28941499438218088, -6.500000000000000000 ) ) ;
#15936=EDGE_LOOP ( 'NONE', ( #19377, #3489, #15187, #14790 ) ) ;
#15937=DIRECTION ( 'NONE',  ( 1.000000000000000000, 0.000000000000000000, 0.000000000000000000 ) ) ;
#15949=ORIENTED_EDGE ( 'NONE', *, *, #6190, .F. ) ;
#15950=CIRCLE ( 'NONE', #25538, 31.10000000000000142 ) ;
#15951=AXIS2_PLACEMENT_3D ( 'NONE', #20815, #17415, #19233 ) ;
#15954=EDGE_LOOP ( 'NONE', ( #9178, #22611, #25525, #13634 ) ) ;
#15958=CARTESIAN_POINT ( 'NONE',  ( 30.45149776762729488, 6.317933499823326748, -2.750000000000000000 ) ) ;
#15962=VECTOR ( 'NONE', #14114, 1000.000000000000000 ) ;
#15966=AXIS2_PLACEMENT_3D ( 'NONE', #8724, #14756, #11191 ) ;
#15968=VECTOR ( 'NONE', #17799, 1000.000000000000000 ) ;
#15969=EDGE_CURVE ( 'NONE', #3288, #10049, #19538, .T. ) ;
#15970=CARTESIAN_POINT ( 'NONE',  ( -16.66421332384646448, 26.25859848311288403, -6.500000000000000000 ) ) ;
#15973=VECTOR ( 'NONE', #15364, 1000.000000000000000 ) ;
#15974=LINE ( 'NONE', #18441, #21322 ) ;
#15976=DIRECTION ( 'NONE',  ( 1.000000000000000000, 0.000000000000000000, 0.000000000000000000 ) ) ;
#15978=AXIS2_PLACEMENT_3D ( 'NONE', #24243, #6331, #18504 ) ;
#15981=CYLINDRICAL_SURFACE ( 'NONE', #10819, 31.10000000000000142 ) ;
#15984=DIRECTION ( 'NONE',  ( -0.9048270524660229075, -0.4257792915650654986, 0.000000000000000000 ) ) ;
#15987=AXIS2_PLACEMENT_3D ( 'NONE', #9297, #15435, #25249 ) ;
#15988=ORIENTED_EDGE ( 'NONE', *, *, #12397, .F. ) ;
#15990=ORIENTED_EDGE ( 'NONE', *, *, #3818, .F. ) ;
#15991=VERTEX_POINT ( 'NONE', #4321 ) ;
#15992=DIRECTION ( 'NONE',  ( -0.000000000000000000, 0.000000000000000000, 1.000000000000000000 ) ) ;
#15994=CARTESIAN_POINT ( 'NONE',  ( -12.78762572734017411, 28.34936733434218681, -6.500000000000000000 ) ) ;
#16001=VECTOR ( 'NONE', #647, 1000.000000000000000 ) ;
#16006=AXIS2_PLACEMENT_3D ( 'NONE', #8095, #5863, #3772 ) ;
#16009=ORIENTED_EDGE ( 'NONE', *, *, #4132, .F. ) ;
#16010=ORIENTED_EDGE ( 'NONE', *, *, #25667, .T. ) ;
#16012=ORIENTED_EDGE ( 'NONE', *, *, #24631, .T. ) ;
#16014=AXIS2_PLACEMENT_3D ( 'NONE', #10509, #2289, #10635 ) ;
#16022=DIRECTION ( 'NONE',  ( 1.000000000000000000, 0.000000000000000000, 0.000000000000000000 ) ) ;
#16025=EDGE_CURVE ( 'NONE', #5115, #19269, #8298, .T. ) ;
#16026=DIRECTION ( 'NONE',  ( 1.000000000000000000, 0.000000000000000000, 0.000000000000000000 ) ) ;
#16029=EDGE_CURVE ( 'NONE', #25447, #5108, #22905, .T. ) ;
#16032=CARTESIAN_POINT ( 'NONE',  ( -10.08469938919458286, 29.41953157733104263, -2.750000000000000000 ) ) ;
#16034=DIRECTION ( 'NONE',  ( -0.5877852522924775780, -0.8090169943749443426, 0.000000000000000000 ) ) ;
#16037=CARTESIAN_POINT ( 'NONE',  ( 0.000000000000000000, 0.000000000000000000, -6.500000000000000000 ) ) ;
#16038=ADVANCED_FACE ( 'NONE', ( #21057 ), #8904, .F. ) ;
#16041=CARTESIAN_POINT ( 'NONE',  ( 26.25859848311271705, 16.66421332384673804, -6.500000000000000000 ) ) ;
#16043=ORIENTED_EDGE ( 'NONE', *, *, #1716, .T. ) ;
#16050=CARTESIAN_POINT ( 'NONE',  ( 28.72825533807133169, 11.91206721063041485, 1.000000000000000000 ) ) ;
#16051=EDGE_LOOP ( 'NONE', ( #17743, #3634, #191, #6541 ) ) ;
#16052=ORIENTED_EDGE ( 'NONE', *, *, #20649, .F. ) ;
#16060=LINE ( 'NONE', #2319, #19681 ) ;
#16066=ADVANCED_FACE ( 'NONE', ( #3137 ), #25236, .T. ) ;
#16068=DIRECTION ( 'NONE',  ( -0.8090169943749417891, 0.5877852522924807976, 0.000000000000000000 ) ) ;
#16069=DIRECTION ( 'NONE',  ( 1.000000000000000000, 0.000000000000000000, 0.000000000000000000 ) ) ;
#16073=DIRECTION ( 'NONE',  ( -6.938893903907225222E-15, -1.000000000000000000, 0.000000000000000000 ) ) ;
#16075=EDGE_LOOP ( 'NONE', ( #5451, #17556, #23456, #666 ) ) ;
#16081=ORIENTED_EDGE ( 'NONE', *, *, #11122, .F. ) ;
#16083=ORIENTED_EDGE ( 'NONE', *, *, #9829, .T. ) ;
#16084=FACE_OUTER_BOUND ( 'NONE', #24046, .T. ) ;
#16085=PLANE ( 'NONE',  #17225 ) ;
#16095=CYLINDRICAL_SURFACE ( 'NONE', #20052, 0.5000000000000004441 ) ;
#16097=CARTESIAN_POINT ( 'NONE',  ( -28.72825533807142051, -11.91206721063020701, -6.500000000000000000 ) ) ;
#16100=EDGE_CURVE ( 'NONE', #8164, #12818, #13311, .T. ) ;
#16103=CYLINDRICAL_SURFACE ( 'NONE', #7228, 0.5000000000000004441 ) ;
#16110=ORIENTED_EDGE ( 'NONE', *, *, #24436, .F. ) ;
#16111=ORIENTED_EDGE ( 'NONE', *, *, #2812, .F. ) ;
#16112=ORIENTED_EDGE ( 'NONE', *, *, #460, .T. ) ;
#16113=LINE ( 'NONE', #8258, #1715 ) ;
#16115=EDGE_CURVE ( 'NONE', #15245, #25364, #9284, .T. ) ;
#16116=VERTEX_POINT ( 'NONE', #15177 ) ;
#16120=LINE ( 'NONE', #3957, #25032 ) ;
#16123=CARTESIAN_POINT ( 'NONE',  ( -1.453535542772288247, 31.06601413805604039, 1.000000000000000000 ) ) ;
#16132=DIRECTION ( 'NONE',  ( 1.000000000000000000, 0.000000000000000000, 0.000000000000000000 ) ) ;
#16134=ORIENTED_EDGE ( 'NONE', *, *, #23660, .F. ) ;
#16137=EDGE_LOOP ( 'NONE', ( #24978, #9346, #17335, #8720 ) ) ;
#16138=DIRECTION ( 'NONE',  ( 0.000000000000000000, -0.000000000000000000, 1.000000000000000000 ) ) ;
#16142=VERTEX_POINT ( 'NONE', #12692 ) ;
#16144=CYLINDRICAL_SURFACE ( 'NONE', #15700, 31.10000000000000142 ) ;
#16145=EDGE_LOOP ( 'NONE', ( #20399, #11134 ) ) ;
#16153=FACE_OUTER_BOUND ( 'NONE', #8154, .T. ) ;
#16154=LINE ( 'NONE', #18633, #12883 ) ;
#16155=DIRECTION ( 'NONE',  ( 1.000000000000000000, 0.000000000000000000, 0.000000000000000000 ) ) ;
#16161=ORIENTED_EDGE ( 'NONE', *, *, #21628, .T. ) ;
#16165=EDGE_LOOP ( 'NONE', ( #13020, #13887, #7477, #23566 ) ) ;
#16167=EDGE_CURVE ( 'NONE', #19798, #11078, #2868, .T. ) ;
#16170=VERTEX_POINT ( 'NONE', #12815 ) ;
#16174=EDGE_CURVE ( 'NONE', #16720, #16921, #4963, .T. ) ;
#16175=DIRECTION ( 'NONE',  ( 0.000000000000000000, 0.000000000000000000, 1.000000000000000000 ) ) ;
#16176=LINE ( 'NONE', #354, #10951 ) ;
#16185=FACE_OUTER_BOUND ( 'NONE', #15052, .T. ) ;
#16186=FACE_OUTER_BOUND ( 'NONE', #10426, .T. ) ;
#16191=VERTEX_POINT ( 'NONE', #17647 ) ;
#16192=DIRECTION ( 'NONE',  ( 0.000000000000000000, 0.000000000000000000, 1.000000000000000000 ) ) ;
#16193=CARTESIAN_POINT ( 'NONE',  ( -31.00322564728516639, -2.451530025008796798, -2.750000000000000000 ) ) ;
#16195=CARTESIAN_POINT ( 'NONE',  ( -29.72853858738287869, -9.133673601486284710, 1.000000000000000000 ) ) ;
#16198=ORIENTED_EDGE ( 'NONE', *, *, #13607, .T. ) ;
#16201=CYLINDRICAL_SURFACE ( 'NONE', #22245, 31.10000000000000142 ) ;
#16202=CARTESIAN_POINT ( 'NONE',  ( 9.133673601486471227, 29.72853858738282185, 1.000000000000000000 ) ) ;
#16203=CIRCLE ( 'NONE', #2412, 0.5000000000000003331 ) ;
#16209=AXIS2_PLACEMENT_3D ( 'NONE', #25133, #1335, #23421 ) ;
#16216=DIRECTION ( 'NONE',  ( -0.7705132427757935831, -0.6374239897486843054, 0.000000000000000000 ) ) ;
#16217=CARTESIAN_POINT ( 'NONE',  ( 31.03863125411925239, 1.952785157361540236, -6.500000000000000000 ) ) ;
#16223=DIRECTION ( 'NONE',  ( 1.000000000000000000, 0.000000000000000000, 0.000000000000000000 ) ) ;
#16225=ORIENTED_EDGE ( 'NONE', *, *, #22803, .F. ) ;
#16226=CARTESIAN_POINT ( 'NONE',  ( -23.96296185032722548, -19.82388608118403539, -6.500000000000000000 ) ) ;
#16228=ORIENTED_EDGE ( 'NONE', *, *, #25118, .T. ) ;
#16230=VERTEX_POINT ( 'NONE', #7434 ) ;
#16231=CIRCLE ( 'NONE', #15403, 0.5000000000000005551 ) ;
#16232=ORIENTED_EDGE ( 'NONE', *, *, #21869, .F. ) ;
#16234=VERTEX_POINT ( 'NONE', #21438 ) ;
#16238=CARTESIAN_POINT ( 'NONE',  ( 30.54913349766223973, 5.827558883615938434, -6.500000000000000000 ) ) ;
#16240=EDGE_CURVE ( 'NONE', #51, #8668, #25616, .T. ) ;
#16241=CIRCLE ( 'NONE', #4108, 31.10000000000000142 ) ;
#16243=AXIS2_PLACEMENT_3D ( 'NONE', #20062, #11837, #6076 ) ;
#16246=ADVANCED_FACE ( 'NONE', ( #7700 ), #21825, .F. ) ;
#16250=CIRCLE ( 'NONE', #24193, 31.10000000000000142 ) ;
#16255=CARTESIAN_POINT ( 'NONE',  ( -29.41953157733084012, 10.08469938919518327, 1.000000000000000000 ) ) ;
#16261=VECTOR ( 'NONE', #24463, 1000.000000000000000 ) ;
#16262=ORIENTED_EDGE ( 'NONE', *, *, #23753, .T. ) ;
#16266=ORIENTED_EDGE ( 'NONE', *, *, #19003, .T. ) ;
#16268=DIRECTION ( 'NONE',  ( -0.000000000000000000, -0.000000000000000000, 1.000000000000000000 ) ) ;
#16269=AXIS2_PLACEMENT_3D ( 'NONE', #16612, #4965, #10453 ) ;
#16277=DIRECTION ( 'NONE',  ( -0.000000000000000000, 0.000000000000000000, -1.000000000000000000 ) ) ;
#16280=CIRCLE ( 'NONE', #21704, 0.5000000000000009992 ) ;
#16281=AXIS2_PLACEMENT_3D ( 'NONE', #15183, #25243, #9290 ) ;
#16284=EDGE_CURVE ( 'NONE', #1590, #9464, #3684, .T. ) ;
#16285=DIRECTION ( 'NONE',  ( 0.000000000000000000, -0.000000000000000000, 1.000000000000000000 ) ) ;
#16289=CARTESIAN_POINT ( 'NONE',  ( -30.63887302793240508, 5.335677986745117174, 1.000000000000000000 ) ) ;
#16290=DIRECTION ( 'NONE',  ( -0.000000000000000000, -0.000000000000000000, 1.000000000000000000 ) ) ;
#16291=CARTESIAN_POINT ( 'NONE',  ( 0.000000000000000000, 0.000000000000000000, -6.500000000000000000 ) ) ;
#16292=CIRCLE ( 'NONE', #25466, 0.5000000000000001110 ) ;
#16298=ORIENTED_EDGE ( 'NONE', *, *, #11312, .T. ) ;
#16299=LINE ( 'NONE', #24267, #23344 ) ;
#16301=CARTESIAN_POINT ( 'NONE',  ( -3.401318489840788661, 30.91344420362550593, 1.000000000000000000 ) ) ;
#16303=EDGE_LOOP ( 'NONE', ( #10178, #8039, #8919, #17282 ) ) ;
#16307=CYLINDRICAL_SURFACE ( 'NONE', #22655, 31.10000000000000142 ) ;
#16309=DIRECTION ( 'NONE',  ( 1.000000000000000000, 0.000000000000000000, 0.000000000000000000 ) ) ;
#16311=EDGE_CURVE ( 'NONE', #2754, #414, #15812, .T. ) ;
#16313=LINE ( 'NONE', #19713, #21276 ) ;
#16314=CIRCLE ( 'NONE', #13388, 0.4999999999999996669 ) ;
#16316=DIRECTION ( 'NONE',  ( 0.000000000000000000, 0.000000000000000000, 1.000000000000000000 ) ) ;
#16318=CARTESIAN_POINT ( 'NONE',  ( 0.000000000000000000, 0.000000000000000000, -6.500000000000000000 ) ) ;
#16322=ORIENTED_EDGE ( 'NONE', *, *, #10727, .F. ) ;
#16323=CARTESIAN_POINT ( 'NONE',  ( 23.64116323484224225, -20.20656826142291251, -6.500000000000000000 ) ) ;
#16327=DIRECTION ( 'NONE',  ( 1.000000000000000000, 0.000000000000000000, 0.000000000000000000 ) ) ;
#16328=ORIENTED_EDGE ( 'NONE', *, *, #11210, .T. ) ;
#16330=CARTESIAN_POINT ( 'NONE',  ( 7.734255490826784651, -30.12293631110048153, 1.000000000000000000 ) ) ;
#16331=ORIENTED_EDGE ( 'NONE', *, *, #25449, .T. ) ;
#16335=CARTESIAN_POINT ( 'NONE',  ( -25.45105997952899912, 17.87326343783971083, -6.500000000000000000 ) ) ;
#16337=CIRCLE ( 'NONE', #5052, 0.5000000000000001110 ) ;
#16340=ORIENTED_EDGE ( 'NONE', *, *, #13347, .T. ) ;
#16343=CYLINDRICAL_SURFACE ( 'NONE', #112, 0.5000000000000004441 ) ;
#16346=AXIS2_PLACEMENT_3D ( 'NONE', #24565, #6655, #24840 ) ;
#16347=DIRECTION ( 'NONE',  ( -0.8090169943749498938, -0.5877852522924696954, 0.000000000000000000 ) ) ;
#16354=CARTESIAN_POINT ( 'NONE',  ( 15.41874213889414591, 27.00874656207299651, -2.750000000000000000 ) ) ;
#16355=CIRCLE ( 'NONE', #14263, 0.4999999999999997224 ) ;
#16358=CARTESIAN_POINT ( 'NONE',  ( 19.82388608118411710, -23.96296185032715798, -6.500000000000000000 ) ) ;
#16361=EDGE_CURVE ( 'NONE', #7791, #19636, #19139, .T. ) ;
#16363=AXIS2_PLACEMENT_3D ( 'NONE', #21561, #1693, #15685 ) ;
#16367=CARTESIAN_POINT ( 'NONE',  ( -22.32573188046889356, 21.65113613650366986, -6.500000000000000000 ) ) ;
#16368=DIRECTION ( 'NONE',  ( 1.000000000000000000, 0.000000000000000000, 0.000000000000000000 ) ) ;
#16369=ORIENTED_EDGE ( 'NONE', *, *, #25866, .T. ) ;
#16371=DIRECTION ( 'NONE',  ( -0.000000000000000000, -0.000000000000000000, 1.000000000000000000 ) ) ;
#16372=DIRECTION ( 'NONE',  ( -0.000000000000000000, 0.000000000000000000, -1.000000000000000000 ) ) ;
#16373=VERTEX_POINT ( 'NONE', #4152 ) ;
#16374=AXIS2_PLACEMENT_3D ( 'NONE', #9137, #4349, #20168 ) ;
#16377=ORIENTED_EDGE ( 'NONE', *, *, #5227, .F. ) ;
#16378=ORIENTED_EDGE ( 'NONE', *, *, #13664, .F. ) ;
#16381=AXIS2_PLACEMENT_3D ( 'NONE', #2820, #10184, #12285 ) ;
#16382=ORIENTED_EDGE ( 'NONE', *, *, #5842, .T. ) ;
#16387=DIRECTION ( 'NONE',  ( 0.000000000000000000, 0.000000000000000000, 1.000000000000000000 ) ) ;
#16390=CARTESIAN_POINT ( 'NONE',  ( -22.67092431280609688, -21.28941499438201745, -6.500000000000000000 ) ) ;
#16391=DIRECTION ( 'NONE',  ( -0.000000000000000000, 0.000000000000000000, 1.000000000000000000 ) ) ;
#16394=CARTESIAN_POINT ( 'NONE',  ( -1.952785157361865753, -31.03863125411923463, -6.500000000000000000 ) ) ;
#16398=DIRECTION ( 'NONE',  ( -0.000000000000000000, -0.000000000000000000, 1.000000000000000000 ) ) ;
#16401=EDGE_CURVE ( 'NONE', #4731, #2838, #21234, .T. ) ;
#16402=ORIENTED_EDGE ( 'NONE', *, *, #13888, .T. ) ;
#16404=ADVANCED_FACE ( 'NONE', ( #12263 ), #8092, .F. ) ;
#16406=FACE_OUTER_BOUND ( 'NONE', #577, .T. ) ;
#16407=ORIENTED_EDGE ( 'NONE', *, *, #16934, .T. ) ;
#16409=ORIENTED_EDGE ( 'NONE', *, *, #13212, .F. ) ;
#16410=CARTESIAN_POINT ( 'NONE',  ( 0.000000000000000000, 0.000000000000000000, 1.000000000000000000 ) ) ;
#16413=EDGE_LOOP ( 'NONE', ( #23403, #21553, #18459, #16266 ) ) ;
#16414=CYLINDRICAL_SURFACE ( 'NONE', #13090, 31.10000000000000142 ) ;
#16416=DIRECTION ( 'NONE',  ( 0.000000000000000000, 0.000000000000000000, 1.000000000000000000 ) ) ;
#16417=AXIS2_PLACEMENT_3D ( 'NONE', #20367, #12532, #6517 ) ;
#16420=CARTESIAN_POINT ( 'NONE',  ( 9.610428525060889626, 29.57785765677927614, -6.500000000000000000 ) ) ;
#16421=AXIS2_PLACEMENT_3D ( 'NONE', #14194, #12227, #959 ) ;
#16424=FACE_OUTER_BOUND ( 'NONE', #5390, .T. ) ;
#16425=CIRCLE ( 'NONE', #10151, 0.4999999999999998890 ) ;
#16426=EDGE_CURVE ( 'NONE', #25364, #17650, #2433, .T. ) ;
#16429=CARTESIAN_POINT ( 'NONE',  ( -10.94867358849371541, -28.91604871112453168, 1.000000000000000000 ) ) ;
#16432=AXIS2_PLACEMENT_3D ( 'NONE', #23986, #12075, #8040 ) ;
#16433=CARTESIAN_POINT ( 'NONE',  ( 21.65113613650327196, -22.32573188046928436, -6.500000000000000000 ) ) ;
#16444=ORIENTED_EDGE ( 'NONE', *, *, #25140, .T. ) ;
#16449=DIRECTION ( 'NONE',  ( 0.000000000000000000, 0.000000000000000000, 1.000000000000000000 ) ) ;
#16450=AXIS2_PLACEMENT_3D ( 'NONE', #5224, #25235, #15292 ) ;
#16453=CARTESIAN_POINT ( 'NONE',  ( -31.03863125411922752, 1.952785157361987878, -6.500000000000000000 ) ) ;
#16464=COLOUR_RGB ( '',0.8941176470588234615, 0.8941176470588234615, 0.8941176470588234615 ) ;
#16465=CARTESIAN_POINT ( 'NONE',  ( 13.69242354489153080, 27.92360179968372691, -2.750000000000000000 ) ) ;
#16472=ORIENTED_EDGE ( 'NONE', *, *, #11122, .T. ) ;
#16479=CARTESIAN_POINT ( 'NONE',  ( -21.65113613650359525, -22.32573188046897172, -2.750000000000000000 ) ) ;
#16487=DIRECTION ( 'NONE',  ( 0.9685831611286337406, 0.2486898871648445808, 0.000000000000000000 ) ) ;
#16489=DIRECTION ( 'NONE',  ( 0.000000000000000000, 0.000000000000000000, 1.000000000000000000 ) ) ;
#16494=DIRECTION ( 'NONE',  ( 1.000000000000000000, 0.000000000000000000, 0.000000000000000000 ) ) ;
#16495=DIRECTION ( 'NONE',  ( 1.000000000000000000, 0.000000000000000000, 0.000000000000000000 ) ) ;
#16497=ORIENTED_EDGE ( 'NONE', *, *, #9060, .T. ) ;
#16500=VERTEX_POINT ( 'NONE', #11185 ) ;
#16501=EDGE_CURVE ( 'NONE', #9218, #16230, #3273, .T. ) ;
#16502=ORIENTED_EDGE ( 'NONE', *, *, #4530, .F. ) ;
#16503=ORIENTED_EDGE ( 'NONE', *, *, #13303, .T. ) ;
#16504=EDGE_LOOP ( 'NONE', ( #20707, #4262, #4513, #19656 ) ) ;
#16505=ORIENTED_EDGE ( 'NONE', *, *, #14968, .F. ) ;
#16506=ORIENTED_EDGE ( 'NONE', *, *, #5206, .F. ) ;
#16508=ADVANCED_FACE ( 'NONE', ( #2711 ), #23113, .F. ) ;
#16516=EDGE_CURVE ( 'NONE', #9980, #9464, #10812, .T. ) ;
#16517=DIRECTION ( 'NONE',  ( 0.000000000000000000, -0.000000000000000000, -1.000000000000000000 ) ) ;
#16518=CARTESIAN_POINT ( 'NONE',  ( 11.44867358849329619, -28.91604871112469510, 1.000000000000000000 ) ) ;
#16520=LINE ( 'NONE', #16032, #3348 ) ;
#16527=VERTEX_POINT ( 'NONE', #22729 ) ;
#16529=VERTEX_POINT ( 'NONE', #6624 ) ;
#16531=ORIENTED_EDGE ( 'NONE', *, *, #9891, .F. ) ;
#16537=DIRECTION ( 'NONE',  ( 0.000000000000000000, 0.000000000000000000, 1.000000000000000000 ) ) ;
#16538=EDGE_CURVE ( 'NONE', #16142, #4937, #12061, .T. ) ;
#16541=DIRECTION ( 'NONE',  ( 1.000000000000000000, 0.000000000000000000, 0.000000000000000000 ) ) ;
#16542=CARTESIAN_POINT ( 'NONE',  ( 0.000000000000000000, 0.000000000000000000, -6.500000000000000000 ) ) ;
#16543=DIRECTION ( 'NONE',  ( 1.000000000000000000, 0.000000000000000000, 0.000000000000000000 ) ) ;
#16544=EDGE_CURVE ( 'NONE', #21567, #7608, #14876, .T. ) ;
#16545=EDGE_CURVE ( 'NONE', #1492, #10494, #15422, .T. ) ;
#16554=EDGE_LOOP ( 'NONE', ( #23206, #16595, #8060, #1061 ) ) ;
#16558=ORIENTED_EDGE ( 'NONE', *, *, #208, .F. ) ;
#16559=ORIENTED_EDGE ( 'NONE', *, *, #3416, .T. ) ;
#16560=CARTESIAN_POINT ( 'NONE',  ( -5.827558883616271501, -30.54913349766217934, -6.500000000000000000 ) ) ;
#16566=EDGE_CURVE ( 'NONE', #16529, #5616, #22596, .T. ) ;
#16567=DIRECTION ( 'NONE',  ( 0.3090169943749456194, -0.9510565162951541973, 0.000000000000000000 ) ) ;
#16572=CARTESIAN_POINT ( 'NONE',  ( -28.91604871112448549, 11.44867358849382910, 1.000000000000000000 ) ) ;
#16578=FACE_OUTER_BOUND ( 'NONE', #21270, .T. ) ;
#16580=FACE_OUTER_BOUND ( 'NONE', #6837, .T. ) ;
#16585=DIRECTION ( 'NONE',  ( -0.9297764858882481276, 0.3681245526846864125, 0.000000000000000000 ) ) ;
#16588=CYLINDRICAL_SURFACE ( 'NONE', #17528, 31.10000000000000142 ) ;
#16589=EDGE_LOOP ( 'NONE', ( #844, #13786, #4693, #7028 ) ) ;
#16590=CARTESIAN_POINT ( 'NONE',  ( 27.25313774936419620, 14.98253926456328244, -6.500000000000000000 ) ) ;
#16592=ADVANCED_BREP_SHAPE_REPRESENTATION ( '', ( #4627, #21036 ), #23570 ) ;
#16594=VERTEX_POINT ( 'NONE', #1014 ) ;
#16595=ORIENTED_EDGE ( 'NONE', *, *, #16426, .F. ) ;
#16596=DIRECTION ( 'NONE',  ( 1.000000000000000000, 0.000000000000000000, 0.000000000000000000 ) ) ;
#16598=EDGE_CURVE ( 'NONE', #1524, #18550, #17915, .T. ) ;
#16601=ADVANCED_FACE ( 'NONE', ( #16580 ), #4677, .F. ) ;
#16602=DIRECTION ( 'NONE',  ( -0.06279051952930156388, 0.9980267284282724471, 0.000000000000000000 ) ) ;
#16603=DIRECTION ( 'NONE',  ( 0.000000000000000000, 0.000000000000000000, 1.000000000000000000 ) ) ;
#16612=CARTESIAN_POINT ( 'NONE',  ( -28.91604871112448549, 11.44867358849382910, -6.500000000000000000 ) ) ;
#16613=DIRECTION ( 'NONE',  ( 0.000000000000000000, -0.000000000000000000, -1.000000000000000000 ) ) ;
#16615=CARTESIAN_POINT ( 'NONE',  ( 13.69242354489133895, -27.92360179968382283, -6.500000000000000000 ) ) ;
#16616=DIRECTION ( 'NONE',  ( -0.000000000000000000, -0.000000000000000000, 1.000000000000000000 ) ) ;
#16618=VERTEX_POINT ( 'NONE', #2834 ) ;
#16619=VECTOR ( 'NONE', #23904, 1000.000000000000000 ) ;
#16620=EDGE_LOOP ( 'NONE', ( #14210, #14495, #17945, #17360 ) ) ;
#16621=ORIENTED_EDGE ( 'NONE', *, *, #11592, .F. ) ;
#16622=ORIENTED_EDGE ( 'NONE', *, *, #17910, .F. ) ;
#16624=VERTEX_POINT ( 'NONE', #22851 ) ;
#16630=CARTESIAN_POINT ( 'NONE',  ( 10.98232076577200722, -29.09636799667087459, -2.750000000000000000 ) ) ;
#16631=ADVANCED_FACE ( 'NONE', ( #10802 ), #8866, .T. ) ;
#16632=DIRECTION ( 'NONE',  ( -0.9297764858882532346, -0.3681245526846732008, 0.000000000000000000 ) ) ;
#16633=AXIS2_PLACEMENT_3D ( 'NONE', #25650, #12022, #21473 ) ;
#16635=CYLINDRICAL_SURFACE ( 'NONE', #24223, 0.5000000000000004441 ) ;
#16638=CARTESIAN_POINT ( 'NONE',  ( 19.43607991388971712, -24.27856662945514543, -2.750000000000000000 ) ) ;
#16644=ORIENTED_EDGE ( 'NONE', *, *, #8244, .T. ) ;
#16648=CARTESIAN_POINT ( 'NONE',  ( 28.91604871112465602, 11.44867358849340633, -6.500000000000000000 ) ) ;
#16649=ORIENTED_EDGE ( 'NONE', *, *, #4303, .T. ) ;
#16653=AXIS2_PLACEMENT_3D ( 'NONE', #9020, #7192, #17003 ) ;
#16655=AXIS2_PLACEMENT_3D ( 'NONE', #18788, #875, #7396 ) ;
#16666=DIRECTION ( 'NONE',  ( -0.000000000000000000, 0.000000000000000000, 1.000000000000000000 ) ) ;
#16669=ADVANCED_FACE ( 'NONE', ( #7285 ), #5443, .T. ) ;
#16676=VERTEX_POINT ( 'NONE', #19430 ) ;
#16680=CARTESIAN_POINT ( 'NONE',  ( 0.000000000000000000, 0.000000000000000000, 1.000000000000000000 ) ) ;
#16685=ORIENTED_EDGE ( 'NONE', *, *, #4093, .F. ) ;
#16689=AXIS2_PLACEMENT_3D ( 'NONE', #9482, #19161, #9615 ) ;
#16690=CIRCLE ( 'NONE', #4561, 31.10000000000000142 ) ;
#16693=CIRCLE ( 'NONE', #21284, 0.4999999999999995004 ) ;
#16694=VECTOR ( 'NONE', #16138, 1000.000000000000000 ) ;
#16696=FACE_OUTER_BOUND ( 'NONE', #21896, .T. ) ;
#16697=DIRECTION ( 'NONE',  ( 0.000000000000000000, 0.000000000000000000, 1.000000000000000000 ) ) ;
#16700=DIRECTION ( 'NONE',  ( 0.000000000000000000, 0.000000000000000000, 1.000000000000000000 ) ) ;
#16706=CIRCLE ( 'NONE', #7514, 0.4999999999999991118 ) ;
#16707=CARTESIAN_POINT ( 'NONE',  ( -30.12293631110035363, 7.734255490827311341, -6.500000000000000000 ) ) ;
#16708=VERTEX_POINT ( 'NONE', #7402 ) ;
#16709=CARTESIAN_POINT ( 'NONE',  ( -8.217531866530787710, 29.99470236596041772, -6.500000000000000000 ) ) ;
#16711=DIRECTION ( 'NONE',  ( 0.000000000000000000, 0.000000000000000000, 1.000000000000000000 ) ) ;
#16714=EDGE_CURVE ( 'NONE', #16527, #7608, #5791, .T. ) ;
#16715=DIRECTION ( 'NONE',  ( 0.000000000000000000, 0.000000000000000000, 1.000000000000000000 ) ) ;
#16716=ORIENTED_EDGE ( 'NONE', *, *, #20753, .T. ) ;
#16718=CIRCLE ( 'NONE', #2918, 0.5000000000000002220 ) ;
#16720=VERTEX_POINT ( 'NONE', #9376 ) ;
#16729=CIRCLE ( 'NONE', #858, 31.10000000000000142 ) ;
#16730=VECTOR ( 'NONE', #18168, 1000.000000000000000 ) ;
#16731=ADVANCED_FACE ( 'NONE', ( #9490 ), #7528, .T. ) ;
#16736=CIRCLE ( 'NONE', #12964, 0.5000000000000002220 ) ;
#16738=CARTESIAN_POINT ( 'NONE',  ( -14.98253926456298579, 27.25313774936435962, -6.500000000000000000 ) ) ;
#16743=DIRECTION ( 'NONE',  ( -0.9822872507286897203, -0.1873813145857189666, 0.000000000000000000 ) ) ;
#16745=CARTESIAN_POINT ( 'NONE',  ( 23.01025686871637177, 20.92219106202051293, 1.000000000000000000 ) ) ;
#16748=CYLINDRICAL_SURFACE ( 'NONE', #7486, 0.5000000000000004441 ) ;
#16750=ORIENTED_EDGE ( 'NONE', *, *, #16284, .F. ) ;
#16753=ORIENTED_EDGE ( 'NONE', *, *, #12112, .T. ) ;
#16756=AXIS2_PLACEMENT_3D ( 'NONE', #20914, #22873, #1039 ) ;
#16759=ORIENTED_EDGE ( 'NONE', *, *, #19420, .F. ) ;
#16760=ORIENTED_EDGE ( 'NONE', *, *, #24725, .F. ) ;
#16763=AXIS2_PLACEMENT_3D ( 'NONE', #12155, #21969, #8364 ) ;
#16764=ORIENTED_EDGE ( 'NONE', *, *, #13772, .T. ) ;
#16767=EDGE_CURVE ( 'NONE', #3783, #18040, #12093, .T. ) ;
#16768=VECTOR ( 'NONE', #16277, 1000.000000000000000 ) ;
#16771=CYLINDRICAL_SURFACE ( 'NONE', #18112, 27.10000000000000142 ) ;
#16773=CARTESIAN_POINT ( 'NONE',  ( 29.99470236596032535, 8.217531866531109230, -6.500000000000000000 ) ) ;
#16774=AXIS2_PLACEMENT_3D ( 'NONE', #7423, #7181, #3509 ) ;
#16777=DIRECTION ( 'NONE',  ( 0.000000000000000000, 0.000000000000000000, 1.000000000000000000 ) ) ;
#16779=DIRECTION ( 'NONE',  ( 0.000000000000000000, 0.000000000000000000, 1.000000000000000000 ) ) ;
#16780=CARTESIAN_POINT ( 'NONE',  ( 0.4999838450259763700, 31.09598070739550124, -2.750000000000000000 ) ) ;
#16784=DIRECTION ( 'NONE',  ( 0.5877852522924853496, 0.8090169943749385695, 0.000000000000000000 ) ) ;
#16785=ORIENTED_EDGE ( 'NONE', *, *, #9525, .T. ) ;
#16796=AXIS2_PLACEMENT_3D ( 'NONE', #15335, #11267, #9569 ) ;
#16797=EDGE_LOOP ( 'NONE', ( #25361, #21448, #7128, #20039 ) ) ;
#16798=EDGE_CURVE ( 'NONE', #25452, #25113, #14338, .T. ) ;
#16800=CARTESIAN_POINT ( 'NONE',  ( 0.000000000000000000, 0.000000000000000000, -6.500000000000000000 ) ) ;
#16819=DIRECTION ( 'NONE',  ( 0.000000000000000000, 0.000000000000000000, 1.000000000000000000 ) ) ;
#16823=VERTEX_POINT ( 'NONE', #9875 ) ;
#16825=CIRCLE ( 'NONE', #5540, 0.5000000000000003331 ) ;
#16827=DIRECTION ( 'NONE',  ( 1.000000000000000000, 0.000000000000000000, 0.000000000000000000 ) ) ;
#16828=ORIENTED_EDGE ( 'NONE', *, *, #21161, .F. ) ;
#16830=CARTESIAN_POINT ( 'NONE',  ( -28.14012133169306296, 13.24173596767408867, 1.000000000000000000 ) ) ;
#16832=AXIS2_PLACEMENT_3D ( 'NONE', #16037, #6203, #12090 ) ;
#16836=ADVANCED_FACE ( 'NONE', ( #8304 ), #13944, .F. ) ;
#16840=ADVANCED_FACE ( 'NONE', ( #4377 ), #21912, .F. ) ;
#16841=DIRECTION ( 'NONE',  ( 0.000000000000000000, 0.000000000000000000, 1.000000000000000000 ) ) ;
#16843=AXIS2_PLACEMENT_3D ( 'NONE', #18234, #317, #18358 ) ;
#16848=LINE ( 'NONE', #12781, #12210 ) ;
#16851=CARTESIAN_POINT ( 'NONE',  ( 28.34936733434205536, 12.78762572734047254, -2.750000000000000000 ) ) ;
#16860=CARTESIAN_POINT ( 'NONE',  ( -29.99470236596021167, 8.217531866531519569, -2.750000000000000000 ) ) ;
#16861=AXIS2_PLACEMENT_3D ( 'NONE', #19638, #23186, #15474 ) ;
#16866=FACE_OUTER_BOUND ( 'NONE', #4474, .T. ) ;
#16869=CARTESIAN_POINT ( 'NONE',  ( -30.91344420362550593, -3.401318489840770010, -6.500000000000000000 ) ) ;
#16873=DIRECTION ( 'NONE',  ( 0.000000000000000000, 0.000000000000000000, 1.000000000000000000 ) ) ;
#16876=FACE_OUTER_BOUND ( 'NONE', #15936, .T. ) ;
#16877=CARTESIAN_POINT ( 'NONE',  ( -10.94867358849309547, 28.91604871112477326, -6.500000000000000000 ) ) ;
#16880=CARTESIAN_POINT ( 'NONE',  ( -30.45149776762733751, -6.317933499823126908, -6.500000000000000000 ) ) ;
#16881=FACE_OUTER_BOUND ( 'NONE', #4939, .T. ) ;
#16882=DIRECTION ( 'NONE',  ( 1.000000000000000000, 0.000000000000000000, 0.000000000000000000 ) ) ;
#16886=AXIS2_PLACEMENT_3D ( 'NONE', #12770, #2698, #16309 ) ;
#16887=FACE_OUTER_BOUND ( 'NONE', #16303, .T. ) ;
#16890=DIRECTION ( 'NONE',  ( 0.000000000000000000, 0.000000000000000000, 1.000000000000000000 ) ) ;
#16891=CARTESIAN_POINT ( 'NONE',  ( 10.98232076577222038, 29.09636799667079288, -6.500000000000000000 ) ) ;
#16892=ORIENTED_EDGE ( 'NONE', *, *, #4735, .F. ) ;
#16894=EDGE_LOOP ( 'NONE', ( #14021, #16110, #20938, #20640 ) ) ;
#16896=VERTEX_POINT ( 'NONE', #17330 ) ;
#16902=EDGE_CURVE ( 'NONE', #19632, #14980, #10367, .T. ) ;
#16919=ORIENTED_EDGE ( 'NONE', *, *, #12919, .T. ) ;
#16920=DIRECTION ( 'NONE',  ( 1.000000000000000000, 0.000000000000000000, 0.000000000000000000 ) ) ;
#16921=VERTEX_POINT ( 'NONE', #3316 ) ;
#16923=ORIENTED_EDGE ( 'NONE', *, *, #14254, .T. ) ;
#16925=ORIENTED_EDGE ( 'NONE', *, *, #22050, .F. ) ;
#16928=CARTESIAN_POINT ( 'NONE',  ( -26.75313774936430633, -14.98253926456308172, 1.000000000000000000 ) ) ;
#16934=EDGE_CURVE ( 'NONE', #6185, #17868, #17444, .T. ) ;
#16936=CARTESIAN_POINT ( 'NONE',  ( -1.952785157361201618, 31.03863125411927371, 1.000000000000000000 ) ) ;
#16940=EDGE_CURVE ( 'NONE', #15884, #15503, #19138, .T. ) ;
#16945=ORIENTED_EDGE ( 'NONE', *, *, #22768, .F. ) ;
#16946=ORIENTED_EDGE ( 'NONE', *, *, #4828, .T. ) ;
#16950=ORIENTED_EDGE ( 'NONE', *, *, #2915, .F. ) ;
#16954=DIRECTION ( 'NONE',  ( -0.9921147013144768767, 0.1253332335643120576, 0.000000000000000000 ) ) ;
#16955=AXIS2_PLACEMENT_3D ( 'NONE', #9032, #15055, #23034 ) ;
#16958=CARTESIAN_POINT ( 'NONE',  ( 10.98232076577222038, 29.09636799667079288, -2.750000000000000000 ) ) ;
#16959=DIRECTION ( 'NONE',  ( 1.000000000000000000, 0.000000000000000000, 0.000000000000000000 ) ) ;
#16960=DIRECTION ( 'NONE',  ( 1.000000000000000000, 0.000000000000000000, 0.000000000000000000 ) ) ;
#16969=EDGE_CURVE ( 'NONE', #1309, #12702, #14574, .T. ) ;
#16974=CARTESIAN_POINT ( 'NONE',  ( -21.28941499438192864, 22.67092431280617859, 1.000000000000000000 ) ) ;
#16987=FACE_OUTER_BOUND ( 'NONE', #6937, .T. ) ;
#16990=EDGE_CURVE ( 'NONE', #20797, #2274, #10712, .T. ) ;
#16991=DIRECTION ( 'NONE',  ( 1.000000000000000000, 0.000000000000000000, 0.000000000000000000 ) ) ;
#16993=DIRECTION ( 'NONE',  ( 1.000000000000000000, 0.000000000000000000, 0.000000000000000000 ) ) ;
#16997=CARTESIAN_POINT ( 'NONE',  ( -9.610428525061097460, -29.57785765677920509, 1.000000000000000000 ) ) ;
#17000=DIRECTION ( 'NONE',  ( 1.000000000000000000, 0.000000000000000000, 0.000000000000000000 ) ) ;
#17003=DIRECTION ( 'NONE',  ( -0.2486898871648449971, 0.9685831611286336296, 0.000000000000000000 ) ) ;
#17004=LINE ( 'NONE', #23021, #9577 ) ;
#17005=CARTESIAN_POINT ( 'NONE',  ( -19.82388608118395013, 23.96296185032730364, -6.500000000000000000 ) ) ;
#17006=VERTEX_POINT ( 'NONE', #24337 ) ;
#17007=LINE ( 'NONE', #1441, #10433 ) ;
#17009=ORIENTED_EDGE ( 'NONE', *, *, #19948, .T. ) ;
#17011=ORIENTED_EDGE ( 'NONE', *, *, #19677, .F. ) ;
#17012=ORIENTED_EDGE ( 'NONE', *, *, #23952, .F. ) ;
#17013=VERTEX_POINT ( 'NONE', #2489 ) ;
#17014=EDGE_CURVE ( 'NONE', #21660, #22219, #14657, .T. ) ;
#17015=ORIENTED_EDGE ( 'NONE', *, *, #21739, .T. ) ;
#17016=DIRECTION ( 'NONE',  ( 1.000000000000000000, 0.000000000000000000, 0.000000000000000000 ) ) ;
#17018=EDGE_CURVE ( 'NONE', #7884, #19632, #8378, .T. ) ;
#17022=DIRECTION ( 'NONE',  ( 0.9980267284282724471, 0.06279051952930156388, 0.000000000000000000 ) ) ;
#17027=CARTESIAN_POINT ( 'NONE',  ( 19.82388608118429119, 23.96296185032701587, -6.500000000000000000 ) ) ;
#17028=DIRECTION ( 'NONE',  ( -0.000000000000000000, -0.000000000000000000, 1.000000000000000000 ) ) ;
#17029=DIRECTION ( 'NONE',  ( 0.000000000000000000, 0.000000000000000000, 1.000000000000000000 ) ) ;
#17032=FACE_OUTER_BOUND ( 'NONE', #19001, .T. ) ;
#17034=ORIENTED_EDGE ( 'NONE', *, *, #7074, .F. ) ;
#17036=ORIENTED_EDGE ( 'NONE', *, *, #1628, .F. ) ;
#17039=DIRECTION ( 'NONE',  ( -0.000000000000000000, -0.000000000000000000, 1.000000000000000000 ) ) ;
#17042=EDGE_CURVE ( 'NONE', #14631, #23924, #4578, .T. ) ;
#17048=AXIS2_PLACEMENT_3D ( 'NONE', #15590, #23560, #4053 ) ;
#17061=AXIS2_PLACEMENT_3D ( 'NONE', #10584, #18579, #2103 ) ;
#17066=EDGE_LOOP ( 'NONE', ( #22006, #8689, #7646, #22568 ) ) ;
#17068=DIRECTION ( 'NONE',  ( -0.000000000000000000, -0.000000000000000000, 1.000000000000000000 ) ) ;
#17070=EDGE_CURVE ( 'NONE', #8796, #2564, #2365, .T. ) ;
#17073=ORIENTED_EDGE ( 'NONE', *, *, #3970, .T. ) ;
#17074=DIRECTION ( 'NONE',  ( -0.3090169943749382919, 0.9510565162951566398, 0.000000000000000000 ) ) ;
#17076=FACE_OUTER_BOUND ( 'NONE', #15954, .T. ) ;
#17080=AXIS2_PLACEMENT_3D ( 'NONE', #25295, #15351, #13147 ) ;
#17084=DIRECTION ( 'NONE',  ( 1.000000000000000000, 0.000000000000000000, 0.000000000000000000 ) ) ;
#17091=DIRECTION ( 'NONE',  ( 0.000000000000000000, 0.000000000000000000, -1.000000000000000000 ) ) ;
#17093=CARTESIAN_POINT ( 'NONE',  ( 0.000000000000000000, 0.000000000000000000, 1.000000000000000000 ) ) ;
#17100=CARTESIAN_POINT ( 'NONE',  ( 23.96296185032695192, -19.82388608118436935, -6.500000000000000000 ) ) ;
#17101=ORIENTED_EDGE ( 'NONE', *, *, #12482, .F. ) ;
#17105=ORIENTED_EDGE ( 'NONE', *, *, #25465, .T. ) ;
#17107=VERTEX_POINT ( 'NONE', #22365 ) ;
#17108=ORIENTED_EDGE ( 'NONE', *, *, #1646, .T. ) ;
#17111=VECTOR ( 'NONE', #593, 1000.000000000000000 ) ;
#17112=AXIS2_PLACEMENT_3D ( 'NONE', #15494, #23708, #5793 ) ;
#17113=ADVANCED_FACE ( 'NONE', ( #20145 ), #6288, .F. ) ;
#17115=CIRCLE ( 'NONE', #11670, 0.5000000000000001110 ) ;
#17118=ADVANCED_FACE ( 'NONE', ( #8251 ), #12421, .T. ) ;
#17120=AXIS2_PLACEMENT_3D ( 'NONE', #1253, #22969, #9236 ) ;
#17122=AXIS2_PLACEMENT_3D ( 'NONE', #6900, #25213, #4933 ) ;
#17125=DIRECTION ( 'NONE',  ( 1.000000000000000000, 0.000000000000000000, 0.000000000000000000 ) ) ;
#17126=CARTESIAN_POINT ( 'NONE',  ( -25.75859848311282363, -16.66421332384654974, -6.500000000000000000 ) ) ;
#17130=DIRECTION ( 'NONE',  ( 1.000000000000000000, 0.000000000000000000, 0.000000000000000000 ) ) ;
#17131=CIRCLE ( 'NONE', #5010, 31.10000000000000142 ) ;
#17137=ORIENTED_EDGE ( 'NONE', *, *, #17280, .T. ) ;
#17138=DIRECTION ( 'NONE',  ( 0.000000000000000000, -0.000000000000000000, 1.000000000000000000 ) ) ;
#17139=DIRECTION ( 'NONE',  ( -0.8443279255020205154, -0.5358267949789882190, 0.000000000000000000 ) ) ;
#17142=CIRCLE ( 'NONE', #20453, 31.10000000000000142 ) ;
#17146=DIRECTION ( 'NONE',  ( -0.000000000000000000, 0.000000000000000000, 1.000000000000000000 ) ) ;
#17149=CIRCLE ( 'NONE', #1264, 31.10000000000000142 ) ;
#17154=ADVANCED_FACE ( 'NONE', ( #14279 ), #22243, .F. ) ;
#17160=DIRECTION ( 'NONE',  ( 0.000000000000000000, 0.000000000000000000, 1.000000000000000000 ) ) ;
#17161=CARTESIAN_POINT ( 'NONE',  ( 0.000000000000000000, 0.000000000000000000, -6.500000000000000000 ) ) ;
#17162=EDGE_CURVE ( 'NONE', #23030, #4688, #23367, .T. ) ;
#17163=CARTESIAN_POINT ( 'NONE',  ( -27.64012133169306296, 13.24173596767408867, -6.500000000000000000 ) ) ;
#17165=AXIS2_PLACEMENT_3D ( 'NONE', #9516, #9399, #13582 ) ;
#17167=AXIS2_PLACEMENT_3D ( 'NONE', #17822, #8015, #25789 ) ;
#17170=VERTEX_POINT ( 'NONE', #7321 ) ;
#17171=DIRECTION ( 'NONE',  ( 0.000000000000000000, 0.000000000000000000, 1.000000000000000000 ) ) ;
#17172=AXIS2_PLACEMENT_3D ( 'NONE', #24791, #10915, #10652 ) ;
#17173=ORIENTED_EDGE ( 'NONE', *, *, #25260, .F. ) ;
#17174=AXIS2_PLACEMENT_3D ( 'NONE', #18185, #24323, #20130 ) ;
#17184=CARTESIAN_POINT ( 'NONE',  ( -13.24173596767398742, -28.14012133169310559, 1.000000000000000000 ) ) ;
#17187=DIRECTION ( 'NONE',  ( 0.000000000000000000, -0.000000000000000000, 1.000000000000000000 ) ) ;
#17193=ADVANCED_FACE ( 'NONE', ( #15301 ), #4970, .F. ) ;
#17195=EDGE_CURVE ( 'NONE', #21040, #14500, #9587, .T. ) ;
#17200=VERTEX_POINT ( 'NONE', #16891 ) ;
#17202=CIRCLE ( 'NONE', #10498, 0.4999999999999996114 ) ;
#17204=AXIS2_PLACEMENT_3D ( 'NONE', #16394, #2385, #10338 ) ;
#17205=DIRECTION ( 'NONE',  ( 1.000000000000000000, 0.000000000000000000, 0.000000000000000000 ) ) ;
#17208=LINE ( 'NONE', #11161, #7521 ) ;
#17211=DIRECTION ( 'NONE',  ( -0.4817536741017063306, 0.8763066800438685799, 0.000000000000000000 ) ) ;
#17213=DIRECTION ( 'NONE',  ( 1.000000000000000000, 0.000000000000000000, 0.000000000000000000 ) ) ;
#17214=ORIENTED_EDGE ( 'NONE', *, *, #17014, .T. ) ;
#17216=DIRECTION ( 'NONE',  ( -0.000000000000000000, -0.000000000000000000, 1.000000000000000000 ) ) ;
#17221=CIRCLE ( 'NONE', #23077, 31.10000000000000142 ) ;
#17225=AXIS2_PLACEMENT_3D ( 'NONE', #12004, #18053, #5494 ) ;
#17227=EDGE_CURVE ( 'NONE', #20939, #25359, #21277, .T. ) ;
#17233=LINE ( 'NONE', #1260, #18429 ) ;
#17236=VECTOR ( 'NONE', #17146, 1000.000000000000000 ) ;
#17243=DIRECTION ( 'NONE',  ( 1.000000000000000000, 0.000000000000000000, 0.000000000000000000 ) ) ;
#17244=ORIENTED_EDGE ( 'NONE', *, *, #16311, .T. ) ;
#17246=VECTOR ( 'NONE', #9051, 1000.000000000000000 ) ;
#17247=EDGE_CURVE ( 'NONE', #19150, #22740, #9990, .T. ) ;
#17248=ORIENTED_EDGE ( 'NONE', *, *, #8819, .T. ) ;
#17256=DIRECTION ( 'NONE',  ( -0.000000000000000000, 0.000000000000000000, -1.000000000000000000 ) ) ;
#17258=CIRCLE ( 'NONE', #25188, 31.10000000000000142 ) ;
#17260=CARTESIAN_POINT ( 'NONE',  ( 0.000000000000000000, 0.000000000000000000, 1.000000000000000000 ) ) ;
#17264=DIRECTION ( 'NONE',  ( -0.000000000000000000, -0.000000000000000000, 1.000000000000000000 ) ) ;
#17269=DIRECTION ( 'NONE',  ( 1.000000000000000000, 0.000000000000000000, 0.000000000000000000 ) ) ;
#17270=EDGE_CURVE ( 'NONE', #14460, #20150, #1053, .T. ) ;
#17272=VECTOR ( 'NONE', #3442, 1000.000000000000000 ) ;
#17274=DIRECTION ( 'NONE',  ( 0.7705132427757999114, 0.6374239897486768669, 0.000000000000000000 ) ) ;
#17277=DIRECTION ( 'NONE',  ( 0.000000000000000000, 0.000000000000000000, 1.000000000000000000 ) ) ;
#17278=CARTESIAN_POINT ( 'NONE',  ( 0.000000000000000000, 0.000000000000000000, 1.000000000000000000 ) ) ;
#17279=VERTEX_POINT ( 'NONE', #18838 ) ;
#17280=EDGE_CURVE ( 'NONE', #2220, #16594, #7904, .T. ) ;
#17281=ORIENTED_EDGE ( 'NONE', *, *, #1835, .F. ) ;
#17282=ORIENTED_EDGE ( 'NONE', *, *, #7691, .T. ) ;
#17284=ORIENTED_EDGE ( 'NONE', *, *, #14801, .T. ) ;
#17291=CYLINDRICAL_SURFACE ( 'NONE', #13819, 0.5000000000000004441 ) ;
#17295=FACE_OUTER_BOUND ( 'NONE', #1078, .T. ) ;
#17300=EDGE_CURVE ( 'NONE', #11375, #18764, #15439, .T. ) ;
#17302=CYLINDRICAL_SURFACE ( 'NONE', #11812, 31.10000000000000142 ) ;
#17303=ORIENTED_EDGE ( 'NONE', *, *, #21226, .F. ) ;
#17306=ADVANCED_FACE ( 'NONE', ( #20932 ), #3015, .T. ) ;
#17307=ORIENTED_EDGE ( 'NONE', *, *, #3735, .F. ) ;
#17308=DIRECTION ( 'NONE',  ( -0.9980267284282710039, 0.06279051952932233893, 0.000000000000000000 ) ) ;
#17314=DIRECTION ( 'NONE',  ( 0.000000000000000000, 0.000000000000000000, 1.000000000000000000 ) ) ;
#17316=EDGE_CURVE ( 'NONE', #8421, #2048, #22766, .T. ) ;
#17323=EDGE_CURVE ( 'NONE', #19968, #12673, #20017, .T. ) ;
#17326=CARTESIAN_POINT ( 'NONE',  ( 6.317933499823220167, -30.45149776762731975, 1.000000000000000000 ) ) ;
#17327=ORIENTED_EDGE ( 'NONE', *, *, #23484, .F. ) ;
#17330=CARTESIAN_POINT ( 'NONE',  ( -14.48253926456356666, -27.25313774936403988, -6.500000000000000000 ) ) ;
#17335=ORIENTED_EDGE ( 'NONE', *, *, #932, .F. ) ;
#17336=EDGE_CURVE ( 'NONE', #24543, #13216, #7494, .T. ) ;
#17338=CARTESIAN_POINT ( 'NONE',  ( -23.96296185032681336, 19.82388608118453632, -6.500000000000000000 ) ) ;
#17339=CARTESIAN_POINT ( 'NONE',  ( 0.000000000000000000, 0.000000000000000000, -6.500000000000000000 ) ) ;
#17341=EDGE_CURVE ( 'NONE', #17107, #6707, #16690, .T. ) ;
#17345=EDGE_CURVE ( 'NONE', #13848, #14914, #15029, .T. ) ;
#17346=CARTESIAN_POINT ( 'NONE',  ( 29.41953157733093960, 10.08469938919488484, -2.750000000000000000 ) ) ;
#17349=CARTESIAN_POINT ( 'NONE',  ( -0.4999838450259763700, -31.09598070739550124, -2.750000000000000000 ) ) ;
#17350=CYLINDRICAL_SURFACE ( 'NONE', #6310, 0.5000000000000004441 ) ;
#17360=ORIENTED_EDGE ( 'NONE', *, *, #12071, .T. ) ;
#17370=ORIENTED_EDGE ( 'NONE', *, *, #4364, .T. ) ;
#17371=DIRECTION ( 'NONE',  ( 0.000000000000000000, 0.000000000000000000, 1.000000000000000000 ) ) ;
#17373=ADVANCED_FACE ( 'NONE', ( #15808 ), #13596, .T. ) ;
#17374=CARTESIAN_POINT ( 'NONE',  ( -8.217531866531428975, -29.99470236596023653, -2.750000000000000000 ) ) ;
#17375=EDGE_CURVE ( 'NONE', #9259, #15106, #19606, .T. ) ;
#17378=DIRECTION ( 'NONE',  ( 1.000000000000000000, 0.000000000000000000, 0.000000000000000000 ) ) ;
#17382=DIRECTION ( 'NONE',  ( 0.000000000000000000, -0.000000000000000000, 1.000000000000000000 ) ) ;
#17383=ORIENTED_EDGE ( 'NONE', *, *, #14254, .F. ) ;
#17384=DIRECTION ( 'NONE',  ( 0.000000000000000000, 0.000000000000000000, 1.000000000000000000 ) ) ;
#17385=CARTESIAN_POINT ( 'NONE',  ( -5.827558883616271501, -30.54913349766217934, -6.500000000000000000 ) ) ;
#17386=DIRECTION ( 'NONE',  ( 0.000000000000000000, 0.000000000000000000, 1.000000000000000000 ) ) ;
#17392=CARTESIAN_POINT ( 'NONE',  ( -3.401318489841309578, -30.91344420362545264, 1.000000000000000000 ) ) ;
#17397=ORIENTED_EDGE ( 'NONE', *, *, #2406, .F. ) ;
#17398=VERTEX_POINT ( 'NONE', #21563 ) ;
#17399=EDGE_CURVE ( 'NONE', #10033, #7472, #22530, .T. ) ;
#17400=CARTESIAN_POINT ( 'NONE',  ( 31.00322564728514152, -2.451530025009115654, 1.000000000000000000 ) ) ;
#17414=DIRECTION ( 'NONE',  ( 1.000000000000000000, 0.000000000000000000, 0.000000000000000000 ) ) ;
#17415=DIRECTION ( 'NONE',  ( 0.000000000000000000, 0.000000000000000000, 1.000000000000000000 ) ) ;
#17418=LINE ( 'NONE', #19490, #23309 ) ;
#17422=DIRECTION ( 'NONE',  ( 1.000000000000000000, 0.000000000000000000, 0.000000000000000000 ) ) ;
#17423=VERTEX_POINT ( 'NONE', #1561 ) ;
#17428=EDGE_LOOP ( 'NONE', ( #21863, #16622, #5856, #4096 ) ) ;
#17430=ORIENTED_EDGE ( 'NONE', *, *, #11951, .F. ) ;
#17434=DIRECTION ( 'NONE',  ( -0.9685831611286319642, -0.2486898871648515197, 0.000000000000000000 ) ) ;
#17435=DIRECTION ( 'NONE',  ( 0.000000000000000000, 0.000000000000000000, 1.000000000000000000 ) ) ;
#17437=DIRECTION ( 'NONE',  ( 0.000000000000000000, -0.000000000000000000, -1.000000000000000000 ) ) ;
#17440=CARTESIAN_POINT ( 'NONE',  ( -30.53863125411927371, -1.952785157361310198, 1.000000000000000000 ) ) ;
#17441=ORIENTED_EDGE ( 'NONE', *, *, #6970, .F. ) ;
#17442=VERTEX_POINT ( 'NONE', #9530 ) ;
#17444=LINE ( 'NONE', #8129, #25012 ) ;
#17446=FACE_OUTER_BOUND ( 'NONE', #17844, .T. ) ;
#17453=ORIENTED_EDGE ( 'NONE', *, *, #20383, .T. ) ;
#17457=DIRECTION ( 'NONE',  ( 0.000000000000000000, 0.000000000000000000, 1.000000000000000000 ) ) ;
#17464=VECTOR ( 'NONE', #25138, 1000.000000000000000 ) ;
#17469=EDGE_CURVE ( 'NONE', #19944, #9003, #17944, .T. ) ;
#17470=DIRECTION ( 'NONE',  ( 0.000000000000000000, 0.000000000000000000, 1.000000000000000000 ) ) ;
#17477=DIRECTION ( 'NONE',  ( 1.000000000000000000, 0.000000000000000000, 0.000000000000000000 ) ) ;
#17479=CARTESIAN_POINT ( 'NONE',  ( -27.49048467073837898, 14.54246377227389075, -2.750000000000000000 ) ) ;
#17482=CARTESIAN_POINT ( 'NONE',  ( 9.133673601486375304, -29.72853858738285027, 1.000000000000000000 ) ) ;
#17483=ORIENTED_EDGE ( 'NONE', *, *, #16969, .F. ) ;
#17485=ORIENTED_EDGE ( 'NONE', *, *, #3058, .T. ) ;
#17488=AXIS2_PLACEMENT_3D ( 'NONE', #14062, #2167, #19683 ) ;
#17490=VECTOR ( 'NONE', #13021, 1000.000000000000000 ) ;
#17491=CIRCLE ( 'NONE', #6209, 31.10000000000000142 ) ;
#17494=DIRECTION ( 'NONE',  ( 0.000000000000000000, 0.000000000000000000, 1.000000000000000000 ) ) ;
#17495=CYLINDRICAL_SURFACE ( 'NONE', #3804, 0.5000000000000004441 ) ;
#17498=CARTESIAN_POINT ( 'NONE',  ( 2.451530025009136970, 31.00322564728514152, -2.750000000000000000 ) ) ;
#17500=EDGE_CURVE ( 'NONE', #7090, #22371, #14189, .T. ) ;
#17510=EDGE_LOOP ( 'NONE', ( #10326, #2080, #18464, #16716 ) ) ;
#17514=EDGE_LOOP ( 'NONE', ( #22014, #23955, #13749, #7263 ) ) ;
#17517=EDGE_LOOP ( 'NONE', ( #5707, #12675, #14497, #13753 ) ) ;
#17518=VECTOR ( 'NONE', #3939, 1000.000000000000000 ) ;
#17522=CYLINDRICAL_SURFACE ( 'NONE', #12634, 31.10000000000000142 ) ;
#17523=DIRECTION ( 'NONE',  ( 0.000000000000000000, 0.000000000000000000, 1.000000000000000000 ) ) ;
#17525=CIRCLE ( 'NONE', #17957, 31.10000000000000142 ) ;
#17526=CYLINDRICAL_SURFACE ( 'NONE', #10562, 31.10000000000000142 ) ;
#17527=AXIS2_PLACEMENT_3D ( 'NONE', #1813, #12253, #17755 ) ;
#17528=AXIS2_PLACEMENT_3D ( 'NONE', #14624, #22604, #129 ) ;
#17536=AXIS2_PLACEMENT_3D ( 'NONE', #332, #14339, #2413 ) ;
#17537=EDGE_CURVE ( 'NONE', #27, #7266, #12935, .T. ) ;
#17541=CARTESIAN_POINT ( 'NONE',  ( 21.28941499438209206, -22.67092431280601872, -6.500000000000000000 ) ) ;
#17545=DIRECTION ( 'NONE',  ( -0.1873813145857259888, -0.9822872507286884991, 0.000000000000000000 ) ) ;
#17547=DIRECTION ( 'NONE',  ( 0.000000000000000000, 0.000000000000000000, 1.000000000000000000 ) ) ;
#17548=CARTESIAN_POINT ( 'NONE',  ( 16.66421332384682685, 26.25859848311265310, -6.500000000000000000 ) ) ;
#17549=ORIENTED_EDGE ( 'NONE', *, *, #15566, .T. ) ;
#17550=DIRECTION ( 'NONE',  ( 0.000000000000000000, 0.000000000000000000, 1.000000000000000000 ) ) ;
#17551=ORIENTED_EDGE ( 'NONE', *, *, #25505, .T. ) ;
#17553=CARTESIAN_POINT ( 'NONE',  ( 0.000000000000000000, 0.000000000000000000, -6.500000000000000000 ) ) ;
#17556=ORIENTED_EDGE ( 'NONE', *, *, #1842, .F. ) ;
#17562=FACE_OUTER_BOUND ( 'NONE', #22764, .T. ) ;
#17565=CARTESIAN_POINT ( 'NONE',  ( -31.06601413805600842, 1.453535542772947942, -6.500000000000000000 ) ) ;
#17569=AXIS2_PLACEMENT_3D ( 'NONE', #24684, #3105, #12911 ) ;
#17571=CIRCLE ( 'NONE', #13416, 0.4999999999999997224 ) ;
#17577=ADVANCED_FACE ( 'NONE', ( #24303 ), #24432, .T. ) ;
#17580=AXIS2_PLACEMENT_3D ( 'NONE', #14048, #22400, #22279 ) ;
#17584=EDGE_LOOP ( 'NONE', ( #21833, #13296, #4878, #11230 ) ) ;
#17585=VECTOR ( 'NONE', #4806, 1000.000000000000000 ) ;
#17586=AXIS2_PLACEMENT_3D ( 'NONE', #2509, #8401, #6436 ) ;
#17587=DIRECTION ( 'NONE',  ( 1.000000000000000000, 0.000000000000000000, 0.000000000000000000 ) ) ;
#17588=VERTEX_POINT ( 'NONE', #16195 ) ;
#17589=DIRECTION ( 'NONE',  ( 1.000000000000000000, 0.000000000000000000, 0.000000000000000000 ) ) ;
#17601=CARTESIAN_POINT ( 'NONE',  ( 0.000000000000000000, 0.000000000000000000, -6.500000000000000000 ) ) ;
#17604=CARTESIAN_POINT ( 'NONE',  ( 28.14012133169324414, 13.24173596767369254, -6.500000000000000000 ) ) ;
#17608=VERTEX_POINT ( 'NONE', #4420 ) ;
#17612=ORIENTED_EDGE ( 'NONE', *, *, #16025, .T. ) ;
#17614=EDGE_CURVE ( 'NONE', #12311, #21597, #14595, .T. ) ;
#17615=CARTESIAN_POINT ( 'NONE',  ( 5.827558883615830965, -30.54913349766226105, 1.000000000000000000 ) ) ;
#17616=AXIS2_PLACEMENT_3D ( 'NONE', #4482, #17870, #11852 ) ;
#17619=VERTEX_POINT ( 'NONE', #16335 ) ;
#17621=ADVANCED_FACE ( 'NONE', ( #12272 ), #16588, .T. ) ;
#17623=AXIS2_PLACEMENT_3D ( 'NONE', #16974, #13050, #14621 ) ;
#17631=SURFACE_STYLE_USAGE ( .BOTH. , #1673 ) ;
#17635=AXIS2_PLACEMENT_3D ( 'NONE', #17904, #11763, #3784 ) ;
#17636=LINE ( 'NONE', #7308, #20512 ) ;
#17640=DIRECTION ( 'NONE',  ( 0.000000000000000000, -0.000000000000000000, 1.000000000000000000 ) ) ;
#17642=CARTESIAN_POINT ( 'NONE',  ( -18.28012134629613783, -25.16042852506070560, 1.000000000000000000 ) ) ;
#17646=AXIS2_PLACEMENT_3D ( 'NONE', #2100, #9936, #12 ) ;
#17647=CARTESIAN_POINT ( 'NONE',  ( 30.24338421796779386, -7.248980000274303670, 1.000000000000000000 ) ) ;
#17650=VERTEX_POINT ( 'NONE', #2337 ) ;
#17654=ORIENTED_EDGE ( 'NONE', *, *, #6565, .F. ) ;
#17657=EDGE_LOOP ( 'NONE', ( #16378, #18318, #23690, #7352 ) ) ;
#17661=CARTESIAN_POINT ( 'NONE',  ( -16.23990935651735867, -26.52310962334733446, -6.500000000000000000 ) ) ;
#17662=FACE_OUTER_BOUND ( 'NONE', #16554, .T. ) ;
#17665=ADVANCED_FACE ( 'NONE', ( #19174 ), #3222, .T. ) ;
#17667=ADVANCED_FACE ( 'NONE', ( #9255 ), #13053, .F. ) ;
#17674=AXIS2_PLACEMENT_3D ( 'NONE', #17184, #24896, #8810 ) ;
#17678=CARTESIAN_POINT ( 'NONE',  ( 0.000000000000000000, 0.000000000000000000, -6.500000000000000000 ) ) ;
#17682=AXIS2_PLACEMENT_3D ( 'NONE', #9062, #12996, #25635 ) ;
#17684=CARTESIAN_POINT ( 'NONE',  ( -26.75313774936430633, -14.98253926456308172, -6.500000000000000000 ) ) ;
#17687=ORIENTED_EDGE ( 'NONE', *, *, #5241, .T. ) ;
#17688=VERTEX_POINT ( 'NONE', #8874 ) ;
#17689=CYLINDRICAL_SURFACE ( 'NONE', #3750, 31.10000000000000142 ) ;
#17693=CARTESIAN_POINT ( 'NONE',  ( -29.07785765677917311, 9.610428525061202265, -6.500000000000000000 ) ) ;
#17694=VECTOR ( 'NONE', #25255, 1000.000000000000000 ) ;
#17695=EDGE_CURVE ( 'NONE', #19787, #12101, #7094, .T. ) ;
#17698=LINE ( 'NONE', #7622, #18917 ) ;
#17699=ADVANCED_FACE ( 'NONE', ( #8997 ), #10809, .F. ) ;
#17710=ORIENTED_EDGE ( 'NONE', *, *, #105, .F. ) ;
#17716=ORIENTED_EDGE ( 'NONE', *, *, #5464, .F. ) ;
#17717=ORIENTED_EDGE ( 'NONE', *, *, #18457, .T. ) ;
#17721=EDGE_CURVE ( 'NONE', #15212, #4479, #3332, .T. ) ;
#17722=DIRECTION ( 'NONE',  ( 1.000000000000000000, 0.000000000000000000, 0.000000000000000000 ) ) ;
#17726=EDGE_CURVE ( 'NONE', #583, #17840, #12516, .T. ) ;
#17731=DIRECTION ( 'NONE',  ( 1.000000000000000000, 0.000000000000000000, 0.000000000000000000 ) ) ;
#17743=ORIENTED_EDGE ( 'NONE', *, *, #3569, .T. ) ;
#17745=ORIENTED_EDGE ( 'NONE', *, *, #13555, .T. ) ;
#17746=DIRECTION ( 'NONE',  ( 0.000000000000000000, 0.000000000000000000, 1.000000000000000000 ) ) ;
#17747=VERTEX_POINT ( 'NONE', #7161 ) ;
#17748=ORIENTED_EDGE ( 'NONE', *, *, #4672, .T. ) ;
#17752=ADVANCED_FACE ( 'NONE', ( #12916 ), #19053, .F. ) ;
#17755=DIRECTION ( 'NONE',  ( -0.8090169943749417891, 0.5877852522924807976, 0.000000000000000000 ) ) ;
#17758=CARTESIAN_POINT ( 'NONE',  ( 15.41874213889414591, 27.00874656207299651, -6.500000000000000000 ) ) ;
#17759=EDGE_CURVE ( 'NONE', #22817, #25447, #4588, .T. ) ;
#17761=CARTESIAN_POINT ( 'NONE',  ( -19.43607991389006528, -24.27856662945486832, -6.500000000000000000 ) ) ;
#17771=ORIENTED_EDGE ( 'NONE', *, *, #10247, .F. ) ;
#17773=EDGE_CURVE ( 'NONE', #9386, #7582, #23120, .T. ) ;
#17774=DIRECTION ( 'NONE',  ( -0.000000000000000000, -0.000000000000000000, 1.000000000000000000 ) ) ;
#17777=ORIENTED_EDGE ( 'NONE', *, *, #3064, .F. ) ;
#17778=EDGE_LOOP ( 'NONE', ( #18975, #11020, #2184, #24682 ) ) ;
#17779=ORIENTED_EDGE ( 'NONE', *, *, #12211, .T. ) ;
#17786=EDGE_CURVE ( 'NONE', #11078, #16594, #19194, .T. ) ;
#17797=DIRECTION ( 'NONE',  ( -0.000000000000000000, 0.000000000000000000, -1.000000000000000000 ) ) ;
#17799=DIRECTION ( 'NONE',  ( 0.000000000000000000, -0.000000000000000000, 1.000000000000000000 ) ) ;
#17800=EDGE_CURVE ( 'NONE', #2754, #24465, #7536, .T. ) ;
#17804=FACE_OUTER_BOUND ( 'NONE', #23705, .T. ) ;
#17805=CYLINDRICAL_SURFACE ( 'NONE', #8891, 0.5000000000000004441 ) ;
#17812=ORIENTED_EDGE ( 'NONE', *, *, #18411, .F. ) ;
#17820=DIRECTION ( 'NONE',  ( -0.8443279255020122998, 0.5358267949790012086, 0.000000000000000000 ) ) ;
#17822=CARTESIAN_POINT ( 'NONE',  ( 0.000000000000000000, 0.000000000000000000, 1.000000000000000000 ) ) ;
#17824=SHAPE_DEFINITION_REPRESENTATION ( #22165, #23199 ) ;
#17826=CARTESIAN_POINT ( 'NONE',  ( 0.000000000000000000, 0.000000000000000000, 1.000000000000000000 ) ) ;
#17830=EDGE_CURVE ( 'NONE', #14918, #3258, #25050, .T. ) ;
#17833=EDGE_CURVE ( 'NONE', #8878, #89, #7927, .T. ) ;
#17834=ORIENTED_EDGE ( 'NONE', *, *, #3132, .T. ) ;
#17835=CARTESIAN_POINT ( 'NONE',  ( -25.75859848311282363, -16.66421332384654974, -6.500000000000000000 ) ) ;
#17837=DIRECTION ( 'NONE',  ( 0.000000000000000000, 0.000000000000000000, 1.000000000000000000 ) ) ;
#17838=CARTESIAN_POINT ( 'NONE',  ( -30.10000000000000142, 3.686186865433532535E-15, 0.000000000000000000 ) ) ;
#17839=EDGE_LOOP ( 'NONE', ( #10380, #8521, #23405, #8804 ) ) ;
#17840=VERTEX_POINT ( 'NONE', #23362 ) ;
#17844=EDGE_LOOP ( 'NONE', ( #23749, #117, #15328, #25774 ) ) ;
#17845=DIRECTION ( 'NONE',  ( 0.000000000000000000, 0.000000000000000000, 1.000000000000000000 ) ) ;
#17851=DIRECTION ( 'NONE',  ( 1.000000000000000000, 0.000000000000000000, 0.000000000000000000 ) ) ;
#17854=CARTESIAN_POINT ( 'NONE',  ( -16.16421332384646448, 26.25859848311288403, -6.500000000000000000 ) ) ;
#17857=FACE_OUTER_BOUND ( 'NONE', #8662, .T. ) ;
#17861=AXIS2_PLACEMENT_3D ( 'NONE', #25857, #4284, #18272 ) ;
#17862=CARTESIAN_POINT ( 'NONE',  ( -7.234255490827218082, -30.12293631110037140, 1.000000000000000000 ) ) ;
#17864=ORIENTED_EDGE ( 'NONE', *, *, #15130, .F. ) ;
#17868=VERTEX_POINT ( 'NONE', #1920 ) ;
#17870=DIRECTION ( 'NONE',  ( 0.000000000000000000, 0.000000000000000000, 1.000000000000000000 ) ) ;
#17875=CARTESIAN_POINT ( 'NONE',  ( -31.06601413805604039, -1.453535542772269595, -2.750000000000000000 ) ) ;
#17879=AXIS2_PLACEMENT_3D ( 'NONE', #24880, #3163, #19109 ) ;
#17888=ORIENTED_EDGE ( 'NONE', *, *, #23166, .T. ) ;
#17894=ORIENTED_EDGE ( 'NONE', *, *, #3425, .F. ) ;
#17897=DIRECTION ( 'NONE',  ( 0.000000000000000000, 0.000000000000000000, 1.000000000000000000 ) ) ;
#17899=ORIENTED_EDGE ( 'NONE', *, *, #12424, .T. ) ;
#17900=ORIENTED_EDGE ( 'NONE', *, *, #18861, .T. ) ;
#17902=VECTOR ( 'NONE', #10934, 1000.000000000000000 ) ;
#17904=CARTESIAN_POINT ( 'NONE',  ( -5.827558883615604479, 30.54913349766230724, -6.500000000000000000 ) ) ;
#17908=DIRECTION ( 'NONE',  ( 0.000000000000000000, 0.000000000000000000, 1.000000000000000000 ) ) ;
#17910=EDGE_CURVE ( 'NONE', #24490, #23177, #5765, .T. ) ;
#17914=DIRECTION ( 'NONE',  ( 0.000000000000000000, 0.000000000000000000, 1.000000000000000000 ) ) ;
#17915=CIRCLE ( 'NONE', #20846, 27.10000000000000142 ) ;
#17918=AXIS2_PLACEMENT_3D ( 'NONE', #19957, #18751, #7945 ) ;
#17921=DIRECTION ( 'NONE',  ( 1.000000000000000000, 0.000000000000000000, 0.000000000000000000 ) ) ;
#17924=CARTESIAN_POINT ( 'NONE',  ( 0.000000000000000000, 0.000000000000000000, -6.500000000000000000 ) ) ;
#17925=AXIS2_PLACEMENT_3D ( 'NONE', #14238, #13708, #4295 ) ;
#17928=EDGE_LOOP ( 'NONE', ( #24582, #7199, #23197, #11233 ) ) ;
#17929=ADVANCED_FACE ( 'NONE', ( #2687 ), #5035, .F. ) ;
#17934=EDGE_CURVE ( 'NONE', #2244, #21597, #24983, .T. ) ;
#17935=VERTEX_POINT ( 'NONE', #15114 ) ;
#17936=CARTESIAN_POINT ( 'NONE',  ( 27.49048467073852464, 14.54246377227360831, 1.000000000000000000 ) ) ;
#17937=ORIENTED_EDGE ( 'NONE', *, *, #19807, .F. ) ;
#17939=EDGE_LOOP ( 'NONE', ( #21615, #9519, #4847, #20991 ) ) ;
#17940=CARTESIAN_POINT ( 'NONE',  ( -15.41874213889433598, -27.00874656207289704, -6.500000000000000000 ) ) ;
#17942=AXIS2_PLACEMENT_3D ( 'NONE', #14541, #5686, #1782 ) ;
#17944=CIRCLE ( 'NONE', #10392, 0.5000000000000006661 ) ;
#17945=ORIENTED_EDGE ( 'NONE', *, *, #20164, .F. ) ;
#17946=EDGE_CURVE ( 'NONE', #3288, #19467, #4928, .T. ) ;
#17950=AXIS2_PLACEMENT_3D ( 'NONE', #1766, #5549, #9734 ) ;
#17951=DIRECTION ( 'NONE',  ( 0.000000000000000000, -0.000000000000000000, 1.000000000000000000 ) ) ;
#17953=EDGE_CURVE ( 'NONE', #9149, #13257, #11600, .T. ) ;
#17955=DIRECTION ( 'NONE',  ( 1.000000000000000000, 0.000000000000000000, 0.000000000000000000 ) ) ;
#17957=AXIS2_PLACEMENT_3D ( 'NONE', #11789, #19877, #10456 ) ;
#17959=VECTOR ( 'NONE', #1190, 1000.000000000000000 ) ;
#17962=CARTESIAN_POINT ( 'NONE',  ( -28.34936733434187062, 12.78762572734086866, -6.500000000000000000 ) ) ;
#17963=ORIENTED_EDGE ( 'NONE', *, *, #12893, .T. ) ;
#17966=ORIENTED_EDGE ( 'NONE', *, *, #25110, .T. ) ;
#17972=EDGE_LOOP ( 'NONE', ( #23242, #2343, #11014, #8489 ) ) ;
#17973=DIRECTION ( 'NONE',  ( 0.000000000000000000, 0.000000000000000000, 1.000000000000000000 ) ) ;
#17974=AXIS2_PLACEMENT_3D ( 'NONE', #7197, #16890, #25357 ) ;
#17975=ORIENTED_EDGE ( 'NONE', *, *, #4495, .T. ) ;
#17979=CARTESIAN_POINT ( 'NONE',  ( 0.000000000000000000, 0.000000000000000000, -6.500000000000000000 ) ) ;
#17980=AXIS2_PLACEMENT_3D ( 'NONE', #9550, #25261, #15585 ) ;
#17981=CYLINDRICAL_SURFACE ( 'NONE', #3385, 31.10000000000000142 ) ;
#17982=DIRECTION ( 'NONE',  ( 0.000000000000000000, 0.000000000000000000, 1.000000000000000000 ) ) ;
#17989=DIRECTION ( 'NONE',  ( 0.000000000000000000, 0.000000000000000000, 1.000000000000000000 ) ) ;
#17990=AXIS2_PLACEMENT_3D ( 'NONE', #18115, #6573, #190 ) ;
#17991=DIRECTION ( 'NONE',  ( 0.4817536741017267032, 0.8763066800438573667, 0.000000000000000000 ) ) ;
#17994=CYLINDRICAL_SURFACE ( 'NONE', #21009, 0.5000000000000002220 ) ;
#17997=AXIS2_PLACEMENT_3D ( 'NONE', #8367, #22483, #4180 ) ;
#18004=ORIENTED_EDGE ( 'NONE', *, *, #19200, .T. ) ;
#18005=CIRCLE ( 'NONE', #15504, 0.5000000000000003331 ) ;
#18008=DIRECTION ( 'NONE',  ( 0.000000000000000000, 0.000000000000000000, 1.000000000000000000 ) ) ;
#18009=CARTESIAN_POINT ( 'NONE',  ( -28.14012133169333651, -13.24173596767349359, 1.000000000000000000 ) ) ;
#18011=VERTEX_POINT ( 'NONE', #10865 ) ;
#18014=AXIS2_PLACEMENT_3D ( 'NONE', #1090, #9066, #11276 ) ;
#18019=ADVANCED_FACE ( 'NONE', ( #11516 ), #11251, .F. ) ;
#18020=CIRCLE ( 'NONE', #23042, 31.10000000000000142 ) ;
#18023=DIRECTION ( 'NONE',  ( 1.000000000000000000, 0.000000000000000000, 0.000000000000000000 ) ) ;
#18024=CIRCLE ( 'NONE', #15929, 31.10000000000000142 ) ;
#18025=DIRECTION ( 'NONE',  ( -0.1873813145857259888, -0.9822872507286884991, 0.000000000000000000 ) ) ;
#18026=DIRECTION ( 'NONE',  ( -0.000000000000000000, -0.000000000000000000, 1.000000000000000000 ) ) ;
#18027=FACE_OUTER_BOUND ( 'NONE', #14764, .T. ) ;
#18028=CARTESIAN_POINT ( 'NONE',  ( 0.000000000000000000, 0.000000000000000000, -6.500000000000000000 ) ) ;
#18031=VERTEX_POINT ( 'NONE', #21200 ) ;
#18037=CIRCLE ( 'NONE', #3835, 0.5000000000000006661 ) ;
#18040=VERTEX_POINT ( 'NONE', #9046 ) ;
#18042=CARTESIAN_POINT ( 'NONE',  ( -30.12293631110050995, -7.734255490826679846, 1.000000000000000000 ) ) ;
#18043=DIRECTION ( 'NONE',  ( -0.000000000000000000, -0.000000000000000000, 1.000000000000000000 ) ) ;
#18048=VERTEX_POINT ( 'NONE', #23046 ) ;
#18050=ORIENTED_EDGE ( 'NONE', *, *, #4495, .F. ) ;
#18051=CARTESIAN_POINT ( 'NONE',  ( 0.000000000000000000, 0.000000000000000000, -6.500000000000000000 ) ) ;
#18052=AXIS2_PLACEMENT_3D ( 'NONE', #6859, #20447, #4496 ) ;
#18053=DIRECTION ( 'NONE',  ( 0.000000000000000000, 0.000000000000000000, 1.000000000000000000 ) ) ;
#18054=ADVANCED_FACE ( 'NONE', ( #13111 ), #13362, .F. ) ;
#18059=VECTOR ( 'NONE', #3274, 1000.000000000000000 ) ;
#18062=AXIS2_PLACEMENT_3D ( 'NONE', #21851, #3933, #7987 ) ;
#18063=DIRECTION ( 'NONE',  ( -0.000000000000000000, -0.000000000000000000, 1.000000000000000000 ) ) ;
#18064=CARTESIAN_POINT ( 'NONE',  ( -3.401318489840662096, 30.91344420362552015, -6.500000000000000000 ) ) ;
#18070=AXIS2_PLACEMENT_3D ( 'NONE', #997, #14860, #16954 ) ;
#18075=DIRECTION ( 'NONE',  ( 1.000000000000000000, 0.000000000000000000, 0.000000000000000000 ) ) ;
#18076=ORIENTED_EDGE ( 'NONE', *, *, #9801, .T. ) ;
#18080=STYLED_ITEM('',(#25900),#4627);
#18081=ORIENTED_EDGE ( 'NONE', *, *, #21927, .T. ) ;
#18082=ORIENTED_EDGE ( 'NONE', *, *, #24924, .F. ) ;
#18084=ORIENTED_EDGE ( 'NONE', *, *, #13303, .F. ) ;
#18086=VECTOR ( 'NONE', #22100, 1000.000000000000000 ) ;
#18091=DIRECTION ( 'NONE',  ( 0.000000000000000000, 0.000000000000000000, 1.000000000000000000 ) ) ;
#18094=VECTOR ( 'NONE', #9773, 1000.000000000000000 ) ;
#18100=LINE ( 'NONE', #8149, #903 ) ;
#18102=CIRCLE ( 'NONE', #16006, 31.10000000000000142 ) ;
#18103=EDGE_CURVE ( 'NONE', #15991, #10494, #2019, .T. ) ;
#18110=ORIENTED_EDGE ( 'NONE', *, *, #12577, .T. ) ;
#18111=CARTESIAN_POINT ( 'NONE',  ( 0.000000000000000000, 0.000000000000000000, -6.500000000000000000 ) ) ;
#18112=AXIS2_PLACEMENT_3D ( 'NONE', #14674, #22654, #13103 ) ;
#18115=CARTESIAN_POINT ( 'NONE',  ( 30.12293631110040693, -7.734255490827107948, -6.500000000000000000 ) ) ;
#18116=ADVANCED_FACE ( 'NONE', ( #1461 ), #11392, .F. ) ;
#18117=ORIENTED_EDGE ( 'NONE', *, *, #13099, .T. ) ;
#18120=ORIENTED_EDGE ( 'NONE', *, *, #20059, .T. ) ;
#18126=EDGE_CURVE ( 'NONE', #7103, #14795, #15586, .T. ) ;
#18127=CARTESIAN_POINT ( 'NONE',  ( 9.610428525060889626, 29.57785765677927614, -6.500000000000000000 ) ) ;
#18133=CARTESIAN_POINT ( 'NONE',  ( 22.32573188046913160, -21.65113613650342472, 1.000000000000000000 ) ) ;
#18134=ADVANCED_FACE ( 'NONE', ( #17295 ), #23555, .T. ) ;
#18139=ORIENTED_EDGE ( 'NONE', *, *, #18457, .F. ) ;
#18147=DIRECTION ( 'NONE',  ( 1.000000000000000000, 0.000000000000000000, 0.000000000000000000 ) ) ;
#18149=VERTEX_POINT ( 'NONE', #25377 ) ;
#18150=VERTEX_POINT ( 'NONE', #5508 ) ;
#18156=CARTESIAN_POINT ( 'NONE',  ( 0.000000000000000000, 0.000000000000000000, -6.500000000000000000 ) ) ;
#18158=CYLINDRICAL_SURFACE ( 'NONE', #17918, 0.5000000000000004441 ) ;
#18163=LINE ( 'NONE', #19724, #2129 ) ;
#18168=DIRECTION ( 'NONE',  ( -0.000000000000000000, -0.000000000000000000, 1.000000000000000000 ) ) ;
#18169=VERTEX_POINT ( 'NONE', #15319 ) ;
#18171=CARTESIAN_POINT ( 'NONE',  ( -26.75313774936397948, 14.98253926456367502, 1.000000000000000000 ) ) ;
#18173=EDGE_CURVE ( 'NONE', #5321, #18031, #13617, .T. ) ;
#18175=VERTEX_POINT ( 'NONE', #1581 ) ;
#18178=ORIENTED_EDGE ( 'NONE', *, *, #18724, .F. ) ;
#18180=DIRECTION ( 'NONE',  ( 0.000000000000000000, 0.000000000000000000, 1.000000000000000000 ) ) ;
#18185=CARTESIAN_POINT ( 'NONE',  ( -1.952785157361865753, -31.03863125411923463, 1.000000000000000000 ) ) ;
#18186=CARTESIAN_POINT ( 'NONE',  ( 0.000000000000000000, 0.000000000000000000, 1.000000000000000000 ) ) ;
#18188=DIRECTION ( 'NONE',  ( 0.000000000000000000, 0.000000000000000000, 1.000000000000000000 ) ) ;
#18190=CARTESIAN_POINT ( 'NONE',  ( 3.401318489841003601, -30.91344420362548107, 1.000000000000000000 ) ) ;
#18193=CARTESIAN_POINT ( 'NONE',  ( -27.64012133169333651, -13.24173596767349359, -6.500000000000000000 ) ) ;
#18197=CARTESIAN_POINT ( 'NONE',  ( -27.25313774936397948, 14.98253926456367502, -6.500000000000000000 ) ) ;
#18198=CARTESIAN_POINT ( 'NONE',  ( -2.451530025008688440, 31.00322564728517349, -2.750000000000000000 ) ) ;
#18203=ORIENTED_EDGE ( 'NONE', *, *, #3132, .F. ) ;
#18208=AXIS2_PLACEMENT_3D ( 'NONE', #13541, #23714, #13788 ) ;
#18211=EDGE_CURVE ( 'NONE', #14144, #8766, #3264, .T. ) ;
#18213=CARTESIAN_POINT ( 'NONE',  ( 9.133673601486252736, -29.72853858738288935, -6.500000000000000000 ) ) ;
#18215=FACE_OUTER_BOUND ( 'NONE', #1499, .T. ) ;
#18218=LINE ( 'NONE', #17163, #12184 ) ;
#18221=LINE ( 'NONE', #4960, #25562 ) ;
#18227=DIRECTION ( 'NONE',  ( 1.000000000000000000, 0.000000000000000000, 0.000000000000000000 ) ) ;
#18228=ORIENTED_EDGE ( 'NONE', *, *, #12366, .T. ) ;
#18230=EDGE_LOOP ( 'NONE', ( #15241, #13631, #11328, #16112 ) ) ;
#18232=ORIENTED_EDGE ( 'NONE', *, *, #8740, .T. ) ;
#18234=CARTESIAN_POINT ( 'NONE',  ( -21.28941499438192864, 22.67092431280617859, -6.500000000000000000 ) ) ;
#18236=DIRECTION ( 'NONE',  ( 1.000000000000000000, 0.000000000000000000, 0.000000000000000000 ) ) ;
#18238=CARTESIAN_POINT ( 'NONE',  ( 28.14012133169314822, -13.24173596767388794, -6.500000000000000000 ) ) ;
#18239=DIRECTION ( 'NONE',  ( 0.000000000000000000, 0.000000000000000000, 1.000000000000000000 ) ) ;
#18243=DIRECTION ( 'NONE',  ( 0.000000000000000000, 0.000000000000000000, 1.000000000000000000 ) ) ;
#18245=DIRECTION ( 'NONE',  ( 0.1253332335643120576, 0.9921147013144768767, 0.000000000000000000 ) ) ;
#18254=ORIENTED_EDGE ( 'NONE', *, *, #741, .F. ) ;
#18255=ORIENTED_EDGE ( 'NONE', *, *, #6894, .T. ) ;
#18256=CARTESIAN_POINT ( 'NONE',  ( 17.87326343783943017, 25.45105997952919097, 1.000000000000000000 ) ) ;
#18259=ORIENTED_EDGE ( 'NONE', *, *, #20422, .T. ) ;
#18266=EDGE_CURVE ( 'NONE', #24375, #23177, #6603, .T. ) ;
#18267=CARTESIAN_POINT ( 'NONE',  ( -18.28012134629558716, 25.16042852506110705, 1.000000000000000000 ) ) ;
#18268=ADVANCED_FACE ( 'NONE', ( #8241 ), #12017, .F. ) ;
#18270=DIRECTION ( 'NONE',  ( 0.3090169943749591086, 0.9510565162951497564, 0.000000000000000000 ) ) ;
#18272=DIRECTION ( 'NONE',  ( 0.5877852522924853496, 0.8090169943749385695, 0.000000000000000000 ) ) ;
#18278=DIRECTION ( 'NONE',  ( 0.000000000000000000, 0.000000000000000000, 1.000000000000000000 ) ) ;
#18281=ORIENTED_EDGE ( 'NONE', *, *, #4215, .F. ) ;
#18283=CYLINDRICAL_SURFACE ( 'NONE', #15057, 0.5000000000000004441 ) ;
#18286=DIRECTION ( 'NONE',  ( -0.000000000000000000, -0.000000000000000000, 1.000000000000000000 ) ) ;
#18290=ORIENTED_EDGE ( 'NONE', *, *, #7331, .F. ) ;
#18291=EDGE_LOOP ( 'NONE', ( #1563, #10773, #7882, #19579 ) ) ;
#18293=CARTESIAN_POINT ( 'NONE',  ( -30.85476721088030061, -3.897863563849544466, 1.000000000000000000 ) ) ;
#18296=FACE_OUTER_BOUND ( 'NONE', #7414, .T. ) ;
#18297=AXIS2_PLACEMENT_3D ( 'NONE', #6800, #14782, #8368 ) ;
#18305=CARTESIAN_POINT ( 'NONE',  ( 29.09636799667083906, 10.98232076577211558, -6.500000000000000000 ) ) ;
#18307=DIRECTION ( 'NONE',  ( -0.3681245526846803617, -0.9297764858882504591, 0.000000000000000000 ) ) ;
#18312=AXIS2_PLACEMENT_3D ( 'NONE', #9788, #21305, #3769 ) ;
#18313=DIRECTION ( 'NONE',  ( 1.000000000000000000, 0.000000000000000000, 0.000000000000000000 ) ) ;
#18318=ORIENTED_EDGE ( 'NONE', *, *, #14336, .T. ) ;
#18321=VERTEX_POINT ( 'NONE', #6658 ) ;
#18322=ORIENTED_EDGE ( 'NONE', *, *, #13156, .T. ) ;
#18323=EDGE_LOOP ( 'NONE', ( #6696, #15305, #3910, #13333 ) ) ;
#18325=ORIENTED_EDGE ( 'NONE', *, *, #4423, .T. ) ;
#18330=VECTOR ( 'NONE', #11984, 1000.000000000000000 ) ;
#18331=DIRECTION ( 'NONE',  ( 0.000000000000000000, 0.000000000000000000, 1.000000000000000000 ) ) ;
#18333=CARTESIAN_POINT ( 'NONE',  ( -24.66042852506064165, 18.28012134629622309, -6.500000000000000000 ) ) ;
#18334=CIRCLE ( 'NONE', #4114, 31.10000000000000142 ) ;
#18341=CARTESIAN_POINT ( 'NONE',  ( 20.20656826142266738, -23.64116323484245541, -6.500000000000000000 ) ) ;
#18343=CARTESIAN_POINT ( 'NONE',  ( 27.92360179968372691, -13.69242354489151836, 1.000000000000000000 ) ) ;
#18344=FACE_OUTER_BOUND ( 'NONE', #12822, .T. ) ;
#18345=ORIENTED_EDGE ( 'NONE', *, *, #3890, .T. ) ;
#18346=ORIENTED_EDGE ( 'NONE', *, *, #8900, .T. ) ;
#18348=ADVANCED_FACE ( 'NONE', ( #4317 ), #10447, .F. ) ;
#18350=VERTEX_POINT ( 'NONE', #8898 ) ;
#18356=CIRCLE ( 'NONE', #12947, 31.10000000000000142 ) ;
#18358=DIRECTION ( 'NONE',  ( 1.000000000000000000, 0.000000000000000000, 0.000000000000000000 ) ) ;
#18364=CIRCLE ( 'NONE', #22550, 0.4999999999999993894 ) ;
#18365=VECTOR ( 'NONE', #3110, 1000.000000000000000 ) ;
#18367=EDGE_CURVE ( 'NONE', #4477, #5974, #1596, .T. ) ;
#18368=CARTESIAN_POINT ( 'NONE',  ( -7.248980000273892443, 30.24338421796789333, 1.000000000000000000 ) ) ;
#18369=AXIS2_PLACEMENT_3D ( 'NONE', #18998, #9324, #7353 ) ;
#18371=DIRECTION ( 'NONE',  ( 0.000000000000000000, 0.000000000000000000, 1.000000000000000000 ) ) ;
#18375=VECTOR ( 'NONE', #3014, 1000.000000000000000 ) ;
#18376=ORIENTED_EDGE ( 'NONE', *, *, #1122, .F. ) ;
#18381=ORIENTED_EDGE ( 'NONE', *, *, #5227, .T. ) ;
#18382=DIRECTION ( 'NONE',  ( 0.000000000000000000, -0.000000000000000000, 1.000000000000000000 ) ) ;
#18386=CARTESIAN_POINT ( 'NONE',  ( 27.00874656207300717, -15.41874213889412815, 1.000000000000000000 ) ) ;
#18387=VERTEX_POINT ( 'NONE', #16880 ) ;
#18392=FACE_OUTER_BOUND ( 'NONE', #14974, .T. ) ;
#18397=VECTOR ( 'NONE', #5470, 1000.000000000000000 ) ;
#18399=CARTESIAN_POINT ( 'NONE',  ( -24.27856662945480437, 19.43607991389013989, -2.750000000000000000 ) ) ;
#18400=EDGE_CURVE ( 'NONE', #19344, #3259, #12448, .T. ) ;
#18402=DIRECTION ( 'NONE',  ( 0.000000000000000000, 0.000000000000000000, 1.000000000000000000 ) ) ;
#18406=LINE ( 'NONE', #12512, #17585 ) ;
#18408=AXIS2_PLACEMENT_3D ( 'NONE', #8747, #12684, #16602 ) ;
#18411=EDGE_CURVE ( 'NONE', #25359, #6673, #12033, .T. ) ;
#18422=ORIENTED_EDGE ( 'NONE', *, *, #20875, .F. ) ;
#18424=ORIENTED_EDGE ( 'NONE', *, *, #16544, .T. ) ;
#18428=CARTESIAN_POINT ( 'NONE',  ( 13.69242354489133895, -27.92360179968382283, 1.000000000000000000 ) ) ;
#18429=VECTOR ( 'NONE', #25320, 1000.000000000000000 ) ;
#18431=CIRCLE ( 'NONE', #9238, 31.10000000000000142 ) ;
#18433=CIRCLE ( 'NONE', #1732, 0.5000000000000001110 ) ;
#18437=DIRECTION ( 'NONE',  ( 0.000000000000000000, 0.000000000000000000, 1.000000000000000000 ) ) ;
#18438=AXIS2_PLACEMENT_3D ( 'NONE', #3443, #15221, #3179 ) ;
#18439=CARTESIAN_POINT ( 'NONE',  ( 0.000000000000000000, 0.000000000000000000, -6.500000000000000000 ) ) ;
#18441=CARTESIAN_POINT ( 'NONE',  ( -25.98730014090418194, 17.08421000182805471, -2.750000000000000000 ) ) ;
#18445=AXIS2_PLACEMENT_3D ( 'NONE', #5693, #13805, #22031 ) ;
#18448=CARTESIAN_POINT ( 'NONE',  ( -28.91604871112473418, -11.44867358849319849, 1.000000000000000000 ) ) ;
#18451=CARTESIAN_POINT ( 'NONE',  ( -12.74173596767398742, -28.14012133169310559, -6.500000000000000000 ) ) ;
#18452=ORIENTED_EDGE ( 'NONE', *, *, #1178, .T. ) ;
#18453=VECTOR ( 'NONE', #23859, 1000.000000000000000 ) ;
#18456=ORIENTED_EDGE ( 'NONE', *, *, #10643, .F. ) ;
#18457=EDGE_CURVE ( 'NONE', #7884, #23296, #24132, .T. ) ;
#18458=AXIS2_PLACEMENT_3D ( 'NONE', #17642, #14232, #16068 ) ;
#18459=ORIENTED_EDGE ( 'NONE', *, *, #8853, .F. ) ;
#18461=ORIENTED_EDGE ( 'NONE', *, *, #6227, .F. ) ;
#18462=ADVANCED_FACE ( 'NONE', ( #14513 ), #22484, .T. ) ;
#18464=ORIENTED_EDGE ( 'NONE', *, *, #16284, .T. ) ;
#18465=FACE_OUTER_BOUND ( 'NONE', #20073, .T. ) ;
#18467=AXIS2_PLACEMENT_3D ( 'NONE', #24619, #6846, #1086 ) ;
#18469=DIRECTION ( 'NONE',  ( 0.000000000000000000, 0.000000000000000000, 1.000000000000000000 ) ) ;
#18471=VECTOR ( 'NONE', #14506, 1000.000000000000000 ) ;
#18472=CIRCLE ( 'NONE', #14713, 0.5000000000000002220 ) ;
#18481=DIRECTION ( 'NONE',  ( 0.000000000000000000, 0.000000000000000000, 1.000000000000000000 ) ) ;
#18487=CIRCLE ( 'NONE', #19716, 31.10000000000000142 ) ;
#18491=AXIS2_PLACEMENT_3D ( 'NONE', #25652, #2106, #18075 ) ;
#18492=VERTEX_POINT ( 'NONE', #8752 ) ;
#18493=DIRECTION ( 'NONE',  ( 0.9980267284282714479, -0.06279051952931540004, 0.000000000000000000 ) ) ;
#18494=EDGE_CURVE ( 'NONE', #8835, #19766, #14905, .T. ) ;
#18498=CYLINDRICAL_SURFACE ( 'NONE', #4242, 0.5000000000000004441 ) ;
#18500=FACE_OUTER_BOUND ( 'NONE', #19739, .T. ) ;
#18501=ORIENTED_EDGE ( 'NONE', *, *, #24953, .F. ) ;
#18502=CARTESIAN_POINT ( 'NONE',  ( -29.57785765677917311, 9.610428525061202265, 1.000000000000000000 ) ) ;
#18504=DIRECTION ( 'NONE',  ( 1.000000000000000000, 0.000000000000000000, 0.000000000000000000 ) ) ;
#18506=DIRECTION ( 'NONE',  ( 1.000000000000000000, 0.000000000000000000, 0.000000000000000000 ) ) ;
#18507=CARTESIAN_POINT ( 'NONE',  ( 21.65113613650327196, -22.32573188046928436, -2.750000000000000000 ) ) ;
#18508=DIRECTION ( 'NONE',  ( 0.9510565162951541973, -0.3090169943749456194, 0.000000000000000000 ) ) ;
#18512=AXIS2_PLACEMENT_3D ( 'NONE', #23411, #13490, #21456 ) ;
#18517=CIRCLE ( 'NONE', #22264, 31.10000000000000142 ) ;
#18518=DIRECTION ( 'NONE',  ( 0.000000000000000000, 0.000000000000000000, 1.000000000000000000 ) ) ;
#18524=EDGE_CURVE ( 'NONE', #1683, #21954, #4947, .T. ) ;
#18525=ORIENTED_EDGE ( 'NONE', *, *, #18594, .F. ) ;
#18527=DIRECTION ( 'NONE',  ( -0.4257792915650642218, 0.9048270524660235736, 0.000000000000000000 ) ) ;
#18531=EDGE_CURVE ( 'NONE', #18492, #12855, #9277, .T. ) ;
#18533=CARTESIAN_POINT ( 'NONE',  ( 0.000000000000000000, -31.10000000000000142, 1.000000000000000000 ) ) ;
#18536=DIRECTION ( 'NONE',  ( 1.000000000000000000, 0.000000000000000000, 0.000000000000000000 ) ) ;
#18537=EDGE_CURVE ( 'NONE', #21381, #18175, #11627, .T. ) ;
#18539=CYLINDRICAL_SURFACE ( 'NONE', #6, 0.5000000000000004441 ) ;
#18542=DIRECTION ( 'NONE',  ( 0.000000000000000000, 0.000000000000000000, 1.000000000000000000 ) ) ;
#18547=DIRECTION ( 'NONE',  ( -0.9048270524660170233, 0.4257792915650782661, 0.000000000000000000 ) ) ;
#18550=VERTEX_POINT ( 'NONE', #21170 ) ;
#18552=DIRECTION ( 'NONE',  ( 0.000000000000000000, 0.000000000000000000, 1.000000000000000000 ) ) ;
#18560=ORIENTED_EDGE ( 'NONE', *, *, #8340, .T. ) ;
#18562=ORIENTED_EDGE ( 'NONE', *, *, #13888, .F. ) ;
#18563=ORIENTED_EDGE ( 'NONE', *, *, #8779, .F. ) ;
#18564=LINE ( 'NONE', #16479, #16001 ) ;
#18566=EDGE_CURVE ( 'NONE', #6672, #25291, #7046, .T. ) ;
#18579=DIRECTION ( 'NONE',  ( 0.000000000000000000, 0.000000000000000000, 1.000000000000000000 ) ) ;
#18580=DIRECTION ( 'NONE',  ( 0.000000000000000000, 0.000000000000000000, -1.000000000000000000 ) ) ;
#18582=VERTEX_POINT ( 'NONE', #17126 ) ;
#18584=DIRECTION ( 'NONE',  ( -0.000000000000000000, -0.000000000000000000, 1.000000000000000000 ) ) ;
#18586=ORIENTED_EDGE ( 'NONE', *, *, #14702, .F. ) ;
#18588=ORIENTED_EDGE ( 'NONE', *, *, #14804, .F. ) ;
#18589=ADVANCED_FACE ( 'NONE', ( #11216 ), #23387, .T. ) ;
#18591=ORIENTED_EDGE ( 'NONE', *, *, #8949, .T. ) ;
#18594=EDGE_CURVE ( 'NONE', #12237, #19902, #7311, .T. ) ;
#18598=ADVANCED_FACE ( 'NONE', ( #19458 ), #21299, .F. ) ;
#18601=AXIS2_PLACEMENT_3D ( 'NONE', #6661, #8755, #8513 ) ;
#18603=DIRECTION ( 'NONE',  ( -0.000000000000000000, -0.000000000000000000, 1.000000000000000000 ) ) ;
#18605=EDGE_CURVE ( 'NONE', #15851, #12275, #13198, .T. ) ;
#18609=DIRECTION ( 'NONE',  ( -0.000000000000000000, -0.000000000000000000, 1.000000000000000000 ) ) ;
#18610=VERTEX_POINT ( 'NONE', #5471 ) ;
#18614=CARTESIAN_POINT ( 'NONE',  ( -7.734255490827218971, -30.12293631110037140, -6.500000000000000000 ) ) ;
#18616=DIRECTION ( 'NONE',  ( 1.000000000000000000, 0.000000000000000000, 0.000000000000000000 ) ) ;
#18618=DIRECTION ( 'NONE',  ( -0.000000000000000000, -0.000000000000000000, 1.000000000000000000 ) ) ;
#18619=DIRECTION ( 'NONE',  ( 1.000000000000000000, 0.000000000000000000, 0.000000000000000000 ) ) ;
#18620=ORIENTED_EDGE ( 'NONE', *, *, #5330, .T. ) ;
#18627=FACE_OUTER_BOUND ( 'NONE', #9798, .T. ) ;
#18629=EDGE_CURVE ( 'NONE', #10460, #5837, #3513, .T. ) ;
#18633=CARTESIAN_POINT ( 'NONE',  ( 0.4999838450259763700, -31.09598070739550124, -2.750000000000000000 ) ) ;
#18634=DIRECTION ( 'NONE',  ( 1.000000000000000000, 0.000000000000000000, 0.000000000000000000 ) ) ;
#18635=ADVANCED_FACE ( 'NONE', ( #5097 ), #18956, .F. ) ;
#18636=FACE_OUTER_BOUND ( 'NONE', #14920, .T. ) ;
#18638=EDGE_CURVE ( 'NONE', #10717, #5108, #9558, .T. ) ;
#18639=VERTEX_POINT ( 'NONE', #3762 ) ;
#18644=ORIENTED_EDGE ( 'NONE', *, *, #2367, .T. ) ;
#18647=EDGE_LOOP ( 'NONE', ( #12174, #2279, #18178, #3587 ) ) ;
#18657=DIRECTION ( 'NONE',  ( 1.000000000000000000, 0.000000000000000000, 0.000000000000000000 ) ) ;
#18661=CARTESIAN_POINT ( 'NONE',  ( 0.000000000000000000, 0.000000000000000000, 1.000000000000000000 ) ) ;
#18663=DIRECTION ( 'NONE',  ( 0.000000000000000000, 0.000000000000000000, 1.000000000000000000 ) ) ;
#18664=ORIENTED_EDGE ( 'NONE', *, *, #14332, .T. ) ;
#18668=CARTESIAN_POINT ( 'NONE',  ( 11.91206721063030649, -28.72825533807137433, -6.500000000000000000 ) ) ;
#18671=DIRECTION ( 'NONE',  ( 1.000000000000000000, 0.000000000000000000, 0.000000000000000000 ) ) ;
#18683=CYLINDRICAL_SURFACE ( 'NONE', #12614, 31.10000000000000142 ) ;
#18685=CARTESIAN_POINT ( 'NONE',  ( -30.35476721088030061, -3.897863563849544466, 1.000000000000000000 ) ) ;
#18688=FACE_OUTER_BOUND ( 'NONE', #10283, .T. ) ;
#18690=CARTESIAN_POINT ( 'NONE',  ( 0.000000000000000000, 0.000000000000000000, -6.500000000000000000 ) ) ;
#18694=DIRECTION ( 'NONE',  ( 0.000000000000000000, 0.000000000000000000, 1.000000000000000000 ) ) ;
#18695=DIRECTION ( 'NONE',  ( 0.000000000000000000, 0.000000000000000000, 1.000000000000000000 ) ) ;
#18699=CARTESIAN_POINT ( 'NONE',  ( -18.68225429291750928, -24.86329371854754200, -2.750000000000000000 ) ) ;
#18700=ORIENTED_EDGE ( 'NONE', *, *, #15787, .T. ) ;
#18714=CARTESIAN_POINT ( 'NONE',  ( 14.54246377227340048, -27.49048467073863833, -6.500000000000000000 ) ) ;
#18715=CIRCLE ( 'NONE', #11595, 31.10000000000000142 ) ;
#18723=FACE_OUTER_BOUND ( 'NONE', #19385, .T. ) ;
#18724=EDGE_CURVE ( 'NONE', #24543, #10117, #11603, .T. ) ;
#18725=VECTOR ( 'NONE', #7601, 1000.000000000000000 ) ;
#18731=ORIENTED_EDGE ( 'NONE', *, *, #579, .F. ) ;
#18735=EDGE_CURVE ( 'NONE', #246, #1590, #24028, .T. ) ;
#18738=AXIS2_PLACEMENT_3D ( 'NONE', #8477, #12129, #6501 ) ;
#18739=ORIENTED_EDGE ( 'NONE', *, *, #17500, .F. ) ;
#18741=EDGE_CURVE ( 'NONE', #21732, #14041, #8085, .T. ) ;
#18744=CARTESIAN_POINT ( 'NONE',  ( 18.68225429291721795, 24.86329371854775161, 1.000000000000000000 ) ) ;
#18745=VECTOR ( 'NONE', #893, 1000.000000000000000 ) ;
#18751=DIRECTION ( 'NONE',  ( -0.000000000000000000, -0.000000000000000000, 1.000000000000000000 ) ) ;
#18752=AXIS2_PLACEMENT_3D ( 'NONE', #22005, #19652, #7757 ) ;
#18757=AXIS2_PLACEMENT_3D ( 'NONE', #19261, #17435, #21741 ) ;
#18759=DIRECTION ( 'NONE',  ( 1.000000000000000000, 0.000000000000000000, 0.000000000000000000 ) ) ;
#18760=CIRCLE ( 'NONE', #15431, 0.4999999999999997224 ) ;
#18763=CARTESIAN_POINT ( 'NONE',  ( 0.000000000000000000, 0.000000000000000000, 1.000000000000000000 ) ) ;
#18764=VERTEX_POINT ( 'NONE', #13701 ) ;
#18768=FACE_OUTER_BOUND ( 'NONE', #8870, .T. ) ;
#18775=AXIS2_PLACEMENT_3D ( 'NONE', #740, #8709, #2963 ) ;
#18779=AXIS2_PLACEMENT_3D ( 'NONE', #25852, #19952, #1672 ) ;
#18782=FACE_OUTER_BOUND ( 'NONE', #2491, .T. ) ;
#18787=VECTOR ( 'NONE', #6416, 1000.000000000000000 ) ;
#18788=CARTESIAN_POINT ( 'NONE',  ( 0.000000000000000000, 0.000000000000000000, 1.000000000000000000 ) ) ;
#18792=CARTESIAN_POINT ( 'NONE',  ( -13.24173596767339767, 28.14012133169338270, -6.500000000000000000 ) ) ;
#18804=CARTESIAN_POINT ( 'NONE',  ( 0.000000000000000000, 0.000000000000000000, -6.500000000000000000 ) ) ;
#18809=ORIENTED_EDGE ( 'NONE', *, *, #19307, .F. ) ;
#18810=VERTEX_POINT ( 'NONE', #22164 ) ;
#18811=CARTESIAN_POINT ( 'NONE',  ( 0.000000000000000000, 0.000000000000000000, -6.500000000000000000 ) ) ;
#18813=EDGE_CURVE ( 'NONE', #4477, #16624, #16154, .T. ) ;
#18814=AXIS2_PLACEMENT_3D ( 'NONE', #13784, #3583, #1622 ) ;
#18815=DIRECTION ( 'NONE',  ( 1.000000000000000000, 0.000000000000000000, 0.000000000000000000 ) ) ;
#18816=CIRCLE ( 'NONE', #4625, 31.10000000000000142 ) ;
#18823=CARTESIAN_POINT ( 'NONE',  ( -7.734255490826573265, 30.12293631110053838, 1.000000000000000000 ) ) ;
#18824=UNCERTAINTY_MEASURE_WITH_UNIT (LENGTH_MEASURE( 1.000000000000000082E-05 ), #9270, 'distance_accuracy_value', 'NONE');
#18826=CARTESIAN_POINT ( 'NONE',  ( 12.78762572734037484, -28.34936733434209444, -2.750000000000000000 ) ) ;
#18828=FACE_OUTER_BOUND ( 'NONE', #14551, .T. ) ;
#18834=CARTESIAN_POINT ( 'NONE',  ( -29.62293631110050995, -7.734255490826679846, 1.000000000000000000 ) ) ;
#18838=CARTESIAN_POINT ( 'NONE',  ( 25.45105997952912702, -17.87326343783951899, 1.000000000000000000 ) ) ;
#18840=CIRCLE ( 'NONE', #3394, 31.10000000000000142 ) ;
#18841=AXIS2_PLACEMENT_3D ( 'NONE', #16390, #10608, #22625 ) ;
#18842=ORIENTED_EDGE ( 'NONE', *, *, #22255, .T. ) ;
#18848=LINE ( 'NONE', #8527, #4266 ) ;
#18850=CARTESIAN_POINT ( 'NONE',  ( 0.000000000000000000, 0.000000000000000000, 1.000000000000000000 ) ) ;
#18852=EDGE_CURVE ( 'NONE', #12855, #25184, #3690, .T. ) ;
#18861=EDGE_CURVE ( 'NONE', #20629, #22953, #20063, .T. ) ;
#18871=ORIENTED_EDGE ( 'NONE', *, *, #6419, .T. ) ;
#18872=ORIENTED_EDGE ( 'NONE', *, *, #16501, .F. ) ;
#18873=AXIS2_PLACEMENT_3D ( 'NONE', #8554, #2529, #24496 ) ;
#18875=CARTESIAN_POINT ( 'NONE',  ( 0.000000000000000000, 0.000000000000000000, 1.000000000000000000 ) ) ;
#18876=ORIENTED_EDGE ( 'NONE', *, *, #5399, .F. ) ;
#18878=ORIENTED_EDGE ( 'NONE', *, *, #3818, .T. ) ;
#18879=FACE_OUTER_BOUND ( 'NONE', #3552, .T. ) ;
#18881=AXIS2_PLACEMENT_3D ( 'NONE', #25663, #17314, #7480 ) ;
#18882=ORIENTED_EDGE ( 'NONE', *, *, #8296, .F. ) ;
#18883=CYLINDRICAL_SURFACE ( 'NONE', #10989, 0.5000000000000004441 ) ;
#18886=EDGE_CURVE ( 'NONE', #16594, #3917, #20193, .T. ) ;
#18894=AXIS2_PLACEMENT_3D ( 'NONE', #5335, #13318, #23380 ) ;
#18895=AXIS2_PLACEMENT_3D ( 'NONE', #10580, #10313, #18307 ) ;
#18897=CARTESIAN_POINT ( 'NONE',  ( 0.000000000000000000, 0.000000000000000000, -6.500000000000000000 ) ) ;
#18905=DIRECTION ( 'NONE',  ( 1.000000000000000000, 0.000000000000000000, 0.000000000000000000 ) ) ;
#18907=ORIENTED_EDGE ( 'NONE', *, *, #24716, .T. ) ;
#18908=CARTESIAN_POINT ( 'NONE',  ( -30.60000000000000142, 3.257552089140643357E-13, -6.500000000000000000 ) ) ;
#18910=VERTEX_POINT ( 'NONE', #25651 ) ;
#18917=VECTOR ( 'NONE', #5271, 1000.000000000000000 ) ;
#18921=CYLINDRICAL_SURFACE ( 'NONE', #19605, 0.5000000000000004441 ) ;
#18922=DIRECTION ( 'NONE',  ( 0.8763066800438685799, 0.4817536741017063306, 0.000000000000000000 ) ) ;
#18934=CARTESIAN_POINT ( 'NONE',  ( 22.32573188046920265, 21.65113613650335367, -2.750000000000000000 ) ) ;
#18935=ORIENTED_EDGE ( 'NONE', *, *, #21610, .T. ) ;
#18939=DIRECTION ( 'NONE',  ( 0.6374239897486886353, -0.7705132427757902525, 0.000000000000000000 ) ) ;
#18941=CARTESIAN_POINT ( 'NONE',  ( 24.86329371854768766, -18.68225429291730677, 1.000000000000000000 ) ) ;
#18943=ORIENTED_EDGE ( 'NONE', *, *, #21358, .T. ) ;
#18945=ORIENTED_EDGE ( 'NONE', *, *, #13664, .T. ) ;
#18946=EDGE_LOOP ( 'NONE', ( #17370, #12260, #18325, #2038 ) ) ;
#18948=CYLINDRICAL_SURFACE ( 'NONE', #20615, 0.5000000000000004441 ) ;
#18953=CARTESIAN_POINT ( 'NONE',  ( 16.23990935651717393, 26.52310962334745170, -2.750000000000000000 ) ) ;
#18956=CYLINDRICAL_SURFACE ( 'NONE', #21245, 0.5000000000000004441 ) ;
#18959=DIRECTION ( 'NONE',  ( -0.000000000000000000, -0.000000000000000000, 1.000000000000000000 ) ) ;
#18963=DIRECTION ( 'NONE',  ( 1.000000000000000000, 0.000000000000000000, 0.000000000000000000 ) ) ;
#18965=CARTESIAN_POINT ( 'NONE',  ( 29.09636799667083906, 10.98232076577211558, -2.750000000000000000 ) ) ;
#18969=CARTESIAN_POINT ( 'NONE',  ( -14.98253926456356666, -27.25313774936403988, -6.500000000000000000 ) ) ;
#18971=EDGE_CURVE ( 'NONE', #17747, #4816, #16231, .T. ) ;
#18972=VERTEX_POINT ( 'NONE', #12870 ) ;
#18973=ORIENTED_EDGE ( 'NONE', *, *, #5637, .T. ) ;
#18975=ORIENTED_EDGE ( 'NONE', *, *, #18861, .F. ) ;
#18993=DIRECTION ( 'NONE',  ( 1.000000000000000000, 0.000000000000000000, 0.000000000000000000 ) ) ;
#18995=ORIENTED_EDGE ( 'NONE', *, *, #4870, .T. ) ;
#18996=ORIENTED_EDGE ( 'NONE', *, *, #2120, .T. ) ;
#18998=CARTESIAN_POINT ( 'NONE',  ( -28.14012133169333651, -13.24173596767349359, -6.500000000000000000 ) ) ;
#19001=EDGE_LOOP ( 'NONE', ( #1562, #17899, #14826, #3914 ) ) ;
#19003=EDGE_CURVE ( 'NONE', #7580, #18031, #22915, .T. ) ;
#19004=VERTEX_POINT ( 'NONE', #15591 ) ;
#19005=CARTESIAN_POINT ( 'NONE',  ( -27.92360179968363809, 13.69242354489171554, 1.000000000000000000 ) ) ;
#19007=DIRECTION ( 'NONE',  ( -0.9921147013144768767, 0.1253332335643120576, 0.000000000000000000 ) ) ;
#19008=FACE_OUTER_BOUND ( 'NONE', #11338, .T. ) ;
#19011=CARTESIAN_POINT ( 'NONE',  ( 0.000000000000000000, 0.000000000000000000, -6.500000000000000000 ) ) ;
#19014=LINE ( 'NONE', #23195, #9921 ) ;
#19015=EDGE_LOOP ( 'NONE', ( #20799, #6421, #8036, #3068 ) ) ;
#19018=CIRCLE ( 'NONE', #20685, 31.10000000000000142 ) ;
#19019=LINE ( 'NONE', #5286, #829 ) ;
#19028=ORIENTED_EDGE ( 'NONE', *, *, #21994, .T. ) ;
#19033=AXIS2_PLACEMENT_3D ( 'NONE', #588, #11115, #24497 ) ;
#19038=DIRECTION ( 'NONE',  ( -0.5877852522924652545, 0.8090169943749532244, 0.000000000000000000 ) ) ;
#19041=CARTESIAN_POINT ( 'NONE',  ( 10.98232076577200722, -29.09636799667087459, -6.500000000000000000 ) ) ;
#19046=CARTESIAN_POINT ( 'NONE',  ( -30.91344420362550593, -3.401318489840770454, -2.750000000000000000 ) ) ;
#19048=LINE ( 'NONE', #18934, #15889 ) ;
#19050=DIRECTION ( 'NONE',  ( -0.000000000000000000, -0.000000000000000000, 1.000000000000000000 ) ) ;
#19053=CYLINDRICAL_SURFACE ( 'NONE', #23792, 0.5000000000000004441 ) ;
#19054=ORIENTED_EDGE ( 'NONE', *, *, #19386, .T. ) ;
#19057=ORIENTED_EDGE ( 'NONE', *, *, #17934, .T. ) ;
#19066=EDGE_CURVE ( 'NONE', #2564, #184, #17491, .T. ) ;
#19074=DIRECTION ( 'NONE',  ( 1.000000000000000000, 0.000000000000000000, 0.000000000000000000 ) ) ;
#19075=DIRECTION ( 'NONE',  ( 0.6374239897486995154, 0.7705132427757811486, 0.000000000000000000 ) ) ;
#19076=DIRECTION ( 'NONE',  ( 0.000000000000000000, 0.000000000000000000, 1.000000000000000000 ) ) ;
#19077=DIRECTION ( 'NONE',  ( 0.000000000000000000, 0.000000000000000000, 1.000000000000000000 ) ) ;
#19082=CARTESIAN_POINT ( 'NONE',  ( 0.000000000000000000, 0.000000000000000000, -6.500000000000000000 ) ) ;
#19085=DIRECTION ( 'NONE',  ( 0.000000000000000000, 0.000000000000000000, 1.000000000000000000 ) ) ;
#19086=DIRECTION ( 'NONE',  ( 0.000000000000000000, -0.000000000000000000, 1.000000000000000000 ) ) ;
#19089=ORIENTED_EDGE ( 'NONE', *, *, #18173, .T. ) ;
#19090=ORIENTED_EDGE ( 'NONE', *, *, #14693, .F. ) ;
#19091=ORIENTED_EDGE ( 'NONE', *, *, #23124, .T. ) ;
#19092=CARTESIAN_POINT ( 'NONE',  ( 0.000000000000000000, 0.000000000000000000, -6.500000000000000000 ) ) ;
#19093=FACE_OUTER_BOUND ( 'NONE', #21037, .T. ) ;
#19102=CARTESIAN_POINT ( 'NONE',  ( 30.63887302793244061, -5.335677986744896906, -2.750000000000000000 ) ) ;
#19104=CARTESIAN_POINT ( 'NONE',  ( -30.85476721088030061, -3.897863563849544466, -6.500000000000000000 ) ) ;
#19106=DIRECTION ( 'NONE',  ( 0.9510565162951541973, -0.3090169943749456194, 0.000000000000000000 ) ) ;
#19109=DIRECTION ( 'NONE',  ( 1.000000000000000000, 0.000000000000000000, 0.000000000000000000 ) ) ;
#19111=ORIENTED_EDGE ( 'NONE', *, *, #17910, .T. ) ;
#19112=EDGE_LOOP ( 'NONE', ( #22035, #5008, #24857, #11113 ) ) ;
#19114=DIRECTION ( 'NONE',  ( 1.000000000000000000, 0.000000000000000000, 0.000000000000000000 ) ) ;
#19115=ORIENTED_EDGE ( 'NONE', *, *, #24563, .F. ) ;
#19119=ADVANCED_FACE ( 'NONE', ( #17804 ), #7851, .F. ) ;
#19124=EDGE_CURVE ( 'NONE', #10526, #3018, #18760, .T. ) ;
#19127=CARTESIAN_POINT ( 'NONE',  ( -27.92360179968358125, 13.69242354489182922, -2.750000000000000000 ) ) ;
#19129=CARTESIAN_POINT ( 'NONE',  ( 0.000000000000000000, 0.000000000000000000, -6.500000000000000000 ) ) ;
#19132=EDGE_CURVE ( 'NONE', #962, #23712, #406, .T. ) ;
#19136=ORIENTED_EDGE ( 'NONE', *, *, #13959, .T. ) ;
#19138=LINE ( 'NONE', #10077, #24183 ) ;
#19139=CIRCLE ( 'NONE', #18738, 31.10000000000000142 ) ;
#19140=DIRECTION ( 'NONE',  ( 0.000000000000000000, 0.000000000000000000, -1.000000000000000000 ) ) ;
#19141=CIRCLE ( 'NONE', #16655, 31.10000000000000142 ) ;
#19147=AXIS2_PLACEMENT_3D ( 'NONE', #18614, #20042, #20175 ) ;
#19148=CARTESIAN_POINT ( 'NONE',  ( -26.75313774936397948, 14.98253926456367502, -6.500000000000000000 ) ) ;
#19149=AXIS2_PLACEMENT_3D ( 'NONE', #20919, #9134, #19075 ) ;
#19150=VERTEX_POINT ( 'NONE', #15716 ) ;
#19153=DIRECTION ( 'NONE',  ( 1.000000000000000000, 0.000000000000000000, 0.000000000000000000 ) ) ;
#19158=DIRECTION ( 'NONE',  ( -0.000000000000000000, -0.000000000000000000, 1.000000000000000000 ) ) ;
#19161=DIRECTION ( 'NONE',  ( 0.000000000000000000, 0.000000000000000000, 1.000000000000000000 ) ) ;
#19162=CARTESIAN_POINT ( 'NONE',  ( -16.16421332384646448, 26.25859848311288403, 1.000000000000000000 ) ) ;
#19167=DIRECTION ( 'NONE',  ( 0.000000000000000000, 0.000000000000000000, 1.000000000000000000 ) ) ;
#19169=CARTESIAN_POINT ( 'NONE',  ( -9.610428525061097460, -29.57785765677920509, -6.500000000000000000 ) ) ;
#19174=FACE_OUTER_BOUND ( 'NONE', #23400, .T. ) ;
#19177=AXIS2_PLACEMENT_3D ( 'NONE', #3392, #12952, #9025 ) ;
#19184=CIRCLE ( 'NONE', #21692, 0.4999999999999986122 ) ;
#19188=CIRCLE ( 'NONE', #11256, 31.10000000000000142 ) ;
#19189=LINE ( 'NONE', #13317, #7498 ) ;
#19191=AXIS2_PLACEMENT_3D ( 'NONE', #12776, #20746, #21257 ) ;
#19192=ADVANCED_FACE ( 'NONE', ( #7994 ), #15981, .T. ) ;
#19194=CIRCLE ( 'NONE', #2499, 0.4999999999999989453 ) ;
#19195=FACE_OUTER_BOUND ( 'NONE', #6670, .T. ) ;
#19200=EDGE_CURVE ( 'NONE', #8252, #5263, #6536, .T. ) ;
#19201=CARTESIAN_POINT ( 'NONE',  ( -5.327558883616270613, -30.54913349766217934, -6.500000000000000000 ) ) ;
#19205=CARTESIAN_POINT ( 'NONE',  ( 0.000000000000000000, 0.000000000000000000, 1.000000000000000000 ) ) ;
#19207=ORIENTED_EDGE ( 'NONE', *, *, #17953, .T. ) ;
#19209=EDGE_CURVE ( 'NONE', #19467, #22219, #14178, .T. ) ;
#19212=ORIENTED_EDGE ( 'NONE', *, *, #6740, .F. ) ;
#19214=VECTOR ( 'NONE', #2943, 1000.000000000000000 ) ;
#19217=ORIENTED_EDGE ( 'NONE', *, *, #4652, .F. ) ;
#19218=DIRECTION ( 'NONE',  ( 0.000000000000000000, 0.000000000000000000, 1.000000000000000000 ) ) ;
#19220=AXIS2_PLACEMENT_3D ( 'NONE', #19129, #14839, #6979 ) ;
#19225=CARTESIAN_POINT ( 'NONE',  ( 29.99470236596026496, -8.217531866531317064, -2.750000000000000000 ) ) ;
#19229=AXIS2_PLACEMENT_3D ( 'NONE', #21472, #3546, #11519 ) ;
#19232=DIRECTION ( 'NONE',  ( 1.000000000000000000, 0.000000000000000000, 0.000000000000000000 ) ) ;
#19233=DIRECTION ( 'NONE',  ( 1.000000000000000000, 0.000000000000000000, 0.000000000000000000 ) ) ;
#19234=EDGE_CURVE ( 'NONE', #9004, #13890, #20928, .T. ) ;
#19236=AXIS2_PLACEMENT_3D ( 'NONE', #6920, #2863, #8897 ) ;
#19238=AXIS2_PLACEMENT_3D ( 'NONE', #20522, #773, #2617 ) ;
#19244=DIRECTION ( 'NONE',  ( 0.000000000000000000, 0.000000000000000000, 1.000000000000000000 ) ) ;
#19247=EDGE_CURVE ( 'NONE', #2083, #23233, #20002, .T. ) ;
#19249=CARTESIAN_POINT ( 'NONE',  ( 23.01025686871646059, 20.92219106202042056, -6.500000000000000000 ) ) ;
#19252=ORIENTED_EDGE ( 'NONE', *, *, #2922, .F. ) ;
#19254=AXIS2_PLACEMENT_3D ( 'NONE', #5017, #4885, #17434 ) ;
#19255=ORIENTED_EDGE ( 'NONE', *, *, #22425, .F. ) ;
#19259=AXIS2_PLACEMENT_3D ( 'NONE', #357, #12506, #20481 ) ;
#19261=CARTESIAN_POINT ( 'NONE',  ( -27.25313774936397948, 14.98253926456367502, -6.500000000000000000 ) ) ;
#19263=DIRECTION ( 'NONE',  ( 0.000000000000000000, 0.000000000000000000, 1.000000000000000000 ) ) ;
#19266=DIRECTION ( 'NONE',  ( 0.000000000000000000, 0.000000000000000000, 1.000000000000000000 ) ) ;
#19267=CIRCLE ( 'NONE', #17616, 31.10000000000000142 ) ;
#19268=ORIENTED_EDGE ( 'NONE', *, *, #8732, .F. ) ;
#19269=VERTEX_POINT ( 'NONE', #16367 ) ;
#19271=AXIS2_PLACEMENT_3D ( 'NONE', #8994, #16711, #754 ) ;
#19279=VERTEX_POINT ( 'NONE', #8759 ) ;
#19281=DIRECTION ( 'NONE',  ( 0.000000000000000000, 0.000000000000000000, 1.000000000000000000 ) ) ;
#19282=CIRCLE ( 'NONE', #20979, 31.10000000000000142 ) ;
#19283=CARTESIAN_POINT ( 'NONE',  ( -31.06601413805603329, -1.453535542772396605, 1.000000000000000000 ) ) ;
#19284=ORIENTED_EDGE ( 'NONE', *, *, #4498, .T. ) ;
#19288=CIRCLE ( 'NONE', #7611, 0.5000000000000001110 ) ;
#19289=LINE ( 'NONE', #19415, #4339 ) ;
#19291=CIRCLE ( 'NONE', #5101, 0.5000000000000004441 ) ;
#19292=CIRCLE ( 'NONE', #18895, 0.4999999999999997780 ) ;
#19296=CIRCLE ( 'NONE', #20137, 31.10000000000000142 ) ;
#19297=FACE_OUTER_BOUND ( 'NONE', #8836, .T. ) ;
#19299=DIRECTION ( 'NONE',  ( 0.000000000000000000, 0.000000000000000000, 1.000000000000000000 ) ) ;
#19302=ADVANCED_FACE ( 'NONE', ( #2746 ), #16748, .F. ) ;
#19307=EDGE_CURVE ( 'NONE', #21795, #23357, #14994, .T. ) ;
#19311=ORIENTED_EDGE ( 'NONE', *, *, #14571, .T. ) ;
#19316=ORIENTED_EDGE ( 'NONE', *, *, #9208, .F. ) ;
#19318=EDGE_CURVE ( 'NONE', #19944, #10324, #24719, .T. ) ;
#19319=CIRCLE ( 'NONE', #8048, 31.10000000000000142 ) ;
#19322=VERTEX_POINT ( 'NONE', #18834 ) ;
#19323=VERTEX_POINT ( 'NONE', #14912 ) ;
#19326=ADVANCED_FACE ( 'NONE', ( #16887 ), #24333, .T. ) ;
#19329=( NAMED_UNIT ( * ) PLANE_ANGLE_UNIT ( ) SI_UNIT ( $, .RADIAN. ) );
#19330=DIRECTION ( 'NONE',  ( 1.000000000000000000, 0.000000000000000000, 0.000000000000000000 ) ) ;
#19331=CIRCLE ( 'NONE', #22689, 31.10000000000000142 ) ;
#19332=DIRECTION ( 'NONE',  ( 1.000000000000000000, 0.000000000000000000, 0.000000000000000000 ) ) ;
#19334=DIRECTION ( 'NONE',  ( -0.000000000000000000, -0.000000000000000000, 1.000000000000000000 ) ) ;
#19336=DIRECTION ( 'NONE',  ( 0.000000000000000000, -0.000000000000000000, 1.000000000000000000 ) ) ;
#19337=DIRECTION ( 'NONE',  ( 1.000000000000000000, 0.000000000000000000, 0.000000000000000000 ) ) ;
#19340=LINE ( 'NONE', #9138, #15092 ) ;
#19342=CARTESIAN_POINT ( 'NONE',  ( 0.000000000000000000, 0.000000000000000000, -6.500000000000000000 ) ) ;
#19344=VERTEX_POINT ( 'NONE', #2485 ) ;
#19346=CARTESIAN_POINT ( 'NONE',  ( 0.000000000000000000, 0.000000000000000000, -6.500000000000000000 ) ) ;
#19347=CARTESIAN_POINT ( 'NONE',  ( 0.000000000000000000, 0.000000000000000000, -6.500000000000000000 ) ) ;
#19350=ORIENTED_EDGE ( 'NONE', *, *, #9525, .F. ) ;
#19352=VERTEX_POINT ( 'NONE', #2624 ) ;
#19353=ORIENTED_EDGE ( 'NONE', *, *, #18813, .F. ) ;
#19354=CARTESIAN_POINT ( 'NONE',  ( 29.72853858738278987, -9.133673601486577809, -2.750000000000000000 ) ) ;
#19355=CYLINDRICAL_SURFACE ( 'NONE', #3170, 31.10000000000000142 ) ;
#19362=CIRCLE ( 'NONE', #8104, 31.10000000000000142 ) ;
#19363=DIRECTION ( 'NONE',  ( 1.000000000000000000, 0.000000000000000000, 0.000000000000000000 ) ) ;
#19364=LINE ( 'NONE', #19102, #18059 ) ;
#19366=DIRECTION ( 'NONE',  ( 1.000000000000000000, 0.000000000000000000, 0.000000000000000000 ) ) ;
#19371=DIRECTION ( 'NONE',  ( -0.000000000000000000, -0.000000000000000000, 1.000000000000000000 ) ) ;
#19373=DIRECTION ( 'NONE',  ( 1.000000000000000000, 0.000000000000000000, 0.000000000000000000 ) ) ;
#19374=ORIENTED_EDGE ( 'NONE', *, *, #3265, .T. ) ;
#19375=EDGE_CURVE ( 'NONE', #15991, #23923, #6647, .T. ) ;
#19377=ORIENTED_EDGE ( 'NONE', *, *, #4807, .F. ) ;
#19378=ORIENTED_EDGE ( 'NONE', *, *, #4692, .F. ) ;
#19384=ADVANCED_FACE ( 'NONE', ( #6413 ), #14401, .T. ) ;
#19385=EDGE_LOOP ( 'NONE', ( #5175, #11816, #1698, #24914 ) ) ;
#19386=EDGE_CURVE ( 'NONE', #3288, #5826, #22490, .T. ) ;
#19392=EDGE_CURVE ( 'NONE', #9972, #13686, #17004, .T. ) ;
#19394=ORIENTED_EDGE ( 'NONE', *, *, #707, .F. ) ;
#19404=ORIENTED_EDGE ( 'NONE', *, *, #3597, .T. ) ;
#19405=LINE ( 'NONE', #6866, #24213 ) ;
#19411=ORIENTED_EDGE ( 'NONE', *, *, #6894, .F. ) ;
#19415=CARTESIAN_POINT ( 'NONE',  ( -19.32388608118395013, 23.96296185032730364, -6.500000000000000000 ) ) ;
#19419=LINE ( 'NONE', #17349, #9584 ) ;
#19420=EDGE_CURVE ( 'NONE', #24200, #7103, #12073, .T. ) ;
#19421=DIRECTION ( 'NONE',  ( 1.000000000000000000, 0.000000000000000000, 0.000000000000000000 ) ) ;
#19423=AXIS2_PLACEMENT_3D ( 'NONE', #6508, #4541, #14492 ) ;
#19430=CARTESIAN_POINT ( 'NONE',  ( -30.04913349766215802, 5.827558883616378083, -6.500000000000000000 ) ) ;
#19433=CARTESIAN_POINT ( 'NONE',  ( 30.24338421796779386, -7.248980000274303670, -6.500000000000000000 ) ) ;
#19434=ORIENTED_EDGE ( 'NONE', *, *, #4168, .T. ) ;
#19441=EDGE_LOOP ( 'NONE', ( #5176, #16377, #9822, #5516 ) ) ;
#19445=EDGE_CURVE ( 'NONE', #132, #12485, #16250, .T. ) ;
#19449=EDGE_CURVE ( 'NONE', #9415, #10376, #11492, .T. ) ;
#19454=CARTESIAN_POINT ( 'NONE',  ( 28.72825533807124287, -11.91206721063061913, -2.750000000000000000 ) ) ;
#19455=CARTESIAN_POINT ( 'NONE',  ( -31.00322564728512020, 2.451530025009346581, 1.000000000000000000 ) ) ;
#19458=FACE_OUTER_BOUND ( 'NONE', #306, .T. ) ;
#19459=ORIENTED_EDGE ( 'NONE', *, *, #13607, .F. ) ;
#19461=LINE ( 'NONE', #1553, #63 ) ;
#19463=DIRECTION ( 'NONE',  ( 1.000000000000000000, 0.000000000000000000, 0.000000000000000000 ) ) ;
#19466=DIRECTION ( 'NONE',  ( 0.000000000000000000, 0.000000000000000000, 1.000000000000000000 ) ) ;
#19467=VERTEX_POINT ( 'NONE', #21058 ) ;
#19468=CARTESIAN_POINT ( 'NONE',  ( 19.43607991388971712, -24.27856662945514543, -6.500000000000000000 ) ) ;
#19471=EDGE_LOOP ( 'NONE', ( #9708, #7855, #3198, #13342 ) ) ;
#19473=ORIENTED_EDGE ( 'NONE', *, *, #20905, .T. ) ;
#19476=CARTESIAN_POINT ( 'NONE',  ( 0.000000000000000000, 0.000000000000000000, -6.500000000000000000 ) ) ;
#19484=EDGE_CURVE ( 'NONE', #822, #13339, #22519, .T. ) ;
#19487=CARTESIAN_POINT ( 'NONE',  ( 28.91604871112465602, 11.44867358849340633, -6.500000000000000000 ) ) ;
#19490=CARTESIAN_POINT ( 'NONE',  ( -7.248980000274416469, -30.24338421796776544, -2.750000000000000000 ) ) ;
#19504=CARTESIAN_POINT ( 'NONE',  ( -31.09598070739550124, 0.4999838450263022760, -6.500000000000000000 ) ) ;
#19506=CARTESIAN_POINT ( 'NONE',  ( 0.000000000000000000, 0.000000000000000000, -6.500000000000000000 ) ) ;
#19514=VERTEX_POINT ( 'NONE', #3770 ) ;
#19515=ORIENTED_EDGE ( 'NONE', *, *, #4168, .F. ) ;
#19516=EDGE_CURVE ( 'NONE', #23656, #8280, #7894, .T. ) ;
#19518=VERTEX_POINT ( 'NONE', #2211 ) ;
#19521=CYLINDRICAL_SURFACE ( 'NONE', #22148, 31.10000000000000142 ) ;
#19522=EDGE_CURVE ( 'NONE', #23624, #12737, #25851, .T. ) ;
#19523=VERTEX_POINT ( 'NONE', #15803 ) ;
#19525=AXIS2_PLACEMENT_3D ( 'NONE', #15457, #9939, #13743 ) ;
#19526=DIRECTION ( 'NONE',  ( 0.000000000000000000, 0.000000000000000000, 1.000000000000000000 ) ) ;
#19527=ORIENTED_EDGE ( 'NONE', *, *, #9750, .T. ) ;
#19529=LINE ( 'NONE', #11830, #15973 ) ;
#19532=DIRECTION ( 'NONE',  ( 0.000000000000000000, 0.000000000000000000, 1.000000000000000000 ) ) ;
#19535=DIRECTION ( 'NONE',  ( 0.000000000000000000, 0.000000000000000000, 1.000000000000000000 ) ) ;
#19538=CIRCLE ( 'NONE', #19565, 31.10000000000000142 ) ;
#19540=DIRECTION ( 'NONE',  ( 0.5358267949790093132, 0.8443279255020070817, 0.000000000000000000 ) ) ;
#19545=VECTOR ( 'NONE', #310, 1000.000000000000000 ) ;
#19546=DIRECTION ( 'NONE',  ( 0.4257792915650712717, -0.9048270524660203540, 0.000000000000000000 ) ) ;
#19547=CARTESIAN_POINT ( 'NONE',  ( -22.67092431280609688, -21.28941499438201745, -6.500000000000000000 ) ) ;
#19553=EDGE_CURVE ( 'NONE', #12264, #4065, #3302, .T. ) ;
#19559=CARTESIAN_POINT ( 'NONE',  ( 25.98730014090442353, 17.08421000182768523, 1.000000000000000000 ) ) ;
#19560=CARTESIAN_POINT ( 'NONE',  ( -26.25859848311247902, 16.66421332384710752, -6.500000000000000000 ) ) ;
#19565=AXIS2_PLACEMENT_3D ( 'NONE', #2240, #8514, #6411 ) ;
#19566=AXIS2_PLACEMENT_3D ( 'NONE', #19575, #25344, #23641 ) ;
#19571=FILL_AREA_STYLE_COLOUR ( '', #16464 ) ;
#19574=DIRECTION ( 'NONE',  ( 0.000000000000000000, 0.000000000000000000, 1.000000000000000000 ) ) ;
#19575=CARTESIAN_POINT ( 'NONE',  ( 0.000000000000000000, 0.000000000000000000, -6.500000000000000000 ) ) ;
#19579=ORIENTED_EDGE ( 'NONE', *, *, #3890, .F. ) ;
#19580=CARTESIAN_POINT ( 'NONE',  ( -28.14012133169333651, -13.24173596767349359, -6.500000000000000000 ) ) ;
#19584=AXIS2_PLACEMENT_3D ( 'NONE', #6152, #4192, #20390 ) ;
#19589=DIRECTION ( 'NONE',  ( 0.000000000000000000, 0.000000000000000000, 1.000000000000000000 ) ) ;
#19591=ORIENTED_EDGE ( 'NONE', *, *, #20926, .T. ) ;
#19592=AXIS2_PLACEMENT_3D ( 'NONE', #20283, #18331, #21996 ) ;
#19594=VERTEX_POINT ( 'NONE', #23773 ) ;
#19595=EDGE_LOOP ( 'NONE', ( #25216, #18731, #14620, #1566 ) ) ;
#19597=ORIENTED_EDGE ( 'NONE', *, *, #9649, .T. ) ;
#19598=DIRECTION ( 'NONE',  ( 0.7289686274214236539, 0.6845471059286760696, 0.000000000000000000 ) ) ;
#19600=CARTESIAN_POINT ( 'NONE',  ( -20.78941499438192508, 22.67092431280617859, -6.500000000000000000 ) ) ;
#19601=CIRCLE ( 'NONE', #2492, 31.10000000000000142 ) ;
#19603=CYLINDRICAL_SURFACE ( 'NONE', #8905, 0.5000000000000004441 ) ;
#19605=AXIS2_PLACEMENT_3D ( 'NONE', #16453, #1006, #16959 ) ;
#19606=CIRCLE ( 'NONE', #1226, 0.4999999999999996669 ) ;
#19615=DIRECTION ( 'NONE',  ( -0.000000000000000000, -0.000000000000000000, 1.000000000000000000 ) ) ;
#19616=FACE_OUTER_BOUND ( 'NONE', #3322, .T. ) ;
#19619=CARTESIAN_POINT ( 'NONE',  ( -26.25859848311282363, -16.66421332384654974, -6.500000000000000000 ) ) ;
#19625=VERTEX_POINT ( 'NONE', #9790 ) ;
#19626=EDGE_CURVE ( 'NONE', #13647, #14723, #22098, .T. ) ;
#19629=LINE ( 'NONE', #13628, #21712 ) ;
#19632=VERTEX_POINT ( 'NONE', #24157 ) ;
#19634=CIRCLE ( 'NONE', #24660, 31.10000000000000142 ) ;
#19636=VERTEX_POINT ( 'NONE', #9908 ) ;
#19638=CARTESIAN_POINT ( 'NONE',  ( 0.000000000000000000, 0.000000000000000000, -6.500000000000000000 ) ) ;
#19640=AXIS2_PLACEMENT_3D ( 'NONE', #23595, #23710, #3460 ) ;
#19641=DIRECTION ( 'NONE',  ( 0.000000000000000000, 0.000000000000000000, 1.000000000000000000 ) ) ;
#19644=AXIS2_PLACEMENT_3D ( 'NONE', #14904, #11215, #9276 ) ;
#19646=AXIS2_PLACEMENT_3D ( 'NONE', #16738, #24707, #14643 ) ;
#19649=CIRCLE ( 'NONE', #8389, 0.5000000000000007772 ) ;
#19652=DIRECTION ( 'NONE',  ( 0.000000000000000000, 0.000000000000000000, 1.000000000000000000 ) ) ;
#19653=EDGE_LOOP ( 'NONE', ( #25337, #6861, #2814, #3358 ) ) ;
#19654=EDGE_LOOP ( 'NONE', ( #25210, #12332, #10381, #20209 ) ) ;
#19656=ORIENTED_EDGE ( 'NONE', *, *, #15128, .T. ) ;
#19657=CYLINDRICAL_SURFACE ( 'NONE', #17950, 0.5000000000000004441 ) ;
#19661=ORIENTED_EDGE ( 'NONE', *, *, #17300, .F. ) ;
#19663=AXIS2_PLACEMENT_3D ( 'NONE', #12654, #24537, #2709 ) ;
#19666=DIRECTION ( 'NONE',  ( 0.000000000000000000, 0.000000000000000000, -1.000000000000000000 ) ) ;
#19667=VERTEX_POINT ( 'NONE', #16709 ) ;
#19673=EDGE_CURVE ( 'NONE', #20210, #1627, #24426, .T. ) ;
#19676=CIRCLE ( 'NONE', #19254, 0.5000000000000006661 ) ;
#19677=EDGE_CURVE ( 'NONE', #19667, #11616, #1626, .T. ) ;
#19678=CARTESIAN_POINT ( 'NONE',  ( 29.41953157733086854, -10.08469938919509623, -6.500000000000000000 ) ) ;
#19681=VECTOR ( 'NONE', #18026, 1000.000000000000000 ) ;
#19682=DIRECTION ( 'NONE',  ( -0.9921147013144785420, -0.1253332335642980688, 0.000000000000000000 ) ) ;
#19683=DIRECTION ( 'NONE',  ( -0.6845471059286831750, 0.7289686274214168815, 0.000000000000000000 ) ) ;
#19687=DIRECTION ( 'NONE',  ( 0.000000000000000000, -0.000000000000000000, -1.000000000000000000 ) ) ;
#19688=CIRCLE ( 'NONE', #25136, 0.5000000000000007772 ) ;
#19692=EDGE_LOOP ( 'NONE', ( #10622, #19973, #25779, #5352 ) ) ;
#19700=CARTESIAN_POINT ( 'NONE',  ( -3.401318489841309578, -30.91344420362545264, -6.500000000000000000 ) ) ;
#19701=VERTEX_POINT ( 'NONE', #14618 ) ;
#19702=CARTESIAN_POINT ( 'NONE',  ( 0.000000000000000000, 0.000000000000000000, 1.000000000000000000 ) ) ;
#19704=ORIENTED_EDGE ( 'NONE', *, *, #5627, .F. ) ;
#19710=CARTESIAN_POINT ( 'NONE',  ( 27.49048467073848911, -14.54246377227368647, -6.500000000000000000 ) ) ;
#19713=CARTESIAN_POINT ( 'NONE',  ( -30.45149776762720961, 6.317933499823766397, -2.750000000000000000 ) ) ;
#19716=AXIS2_PLACEMENT_3D ( 'NONE', #5358, #21187, #1703 ) ;
#19717=CARTESIAN_POINT ( 'NONE',  ( -29.62293631110035363, 7.734255490827311341, 1.000000000000000000 ) ) ;
#19720=DIRECTION ( 'NONE',  ( 0.000000000000000000, -0.000000000000000000, 1.000000000000000000 ) ) ;
#19723=CARTESIAN_POINT ( 'NONE',  ( 28.14012133169324414, 13.24173596767369254, 1.000000000000000000 ) ) ;
#19724=CARTESIAN_POINT ( 'NONE',  ( -30.63887302793240508, 5.335677986745116286, -2.750000000000000000 ) ) ;
#19725=AXIS2_PLACEMENT_3D ( 'NONE', #9895, #25727, #12117 ) ;
#19727=AXIS2_PLACEMENT_3D ( 'NONE', #19487, #5752, #1582 ) ;
#19731=EDGE_LOOP ( 'NONE', ( #8761, #1871, #23404, #18322 ) ) ;
#19736=ORIENTED_EDGE ( 'NONE', *, *, #3624, .F. ) ;
#19739=EDGE_LOOP ( 'NONE', ( #17307, #6420, #9475, #15467 ) ) ;
#19742=CIRCLE ( 'NONE', #9315, 0.4999999999999999445 ) ;
#19745=VECTOR ( 'NONE', #24067, 1000.000000000000000 ) ;
#19751=EDGE_CURVE ( 'NONE', #16500, #1701, #25036, .T. ) ;
#19753=FACE_OUTER_BOUND ( 'NONE', #1896, .T. ) ;
#19755=DIRECTION ( 'NONE',  ( 1.000000000000000000, 0.000000000000000000, 0.000000000000000000 ) ) ;
#19764=ORIENTED_EDGE ( 'NONE', *, *, #15482, .F. ) ;
#19766=VERTEX_POINT ( 'NONE', #17862 ) ;
#19778=DIRECTION ( 'NONE',  ( 0.1253332335643120576, 0.9921147013144768767, 0.000000000000000000 ) ) ;
#19781=CARTESIAN_POINT ( 'NONE',  ( 0.000000000000000000, 0.000000000000000000, 1.000000000000000000 ) ) ;
#19782=ADVANCED_FACE ( 'NONE', ( #3871 ), #1790, .T. ) ;
#19785=CARTESIAN_POINT ( 'NONE',  ( 0.000000000000000000, 0.000000000000000000, 1.000000000000000000 ) ) ;
#19786=CYLINDRICAL_SURFACE ( 'NONE', #15424, 0.5000000000000004441 ) ;
#19787=VERTEX_POINT ( 'NONE', #15905 ) ;
#19788=VERTEX_POINT ( 'NONE', #15769 ) ;
#19790=EDGE_CURVE ( 'NONE', #4065, #24402, #9758, .T. ) ;
#19794=CARTESIAN_POINT ( 'NONE',  ( 18.68225429291731743, 24.86329371854767700, -6.500000000000000000 ) ) ;
#19798=VERTEX_POINT ( 'NONE', #13945 ) ;
#19800=LINE ( 'NONE', #7897, #18453 ) ;
#19802=CARTESIAN_POINT ( 'NONE',  ( -29.41953157733101065, -10.08469938919468945, -6.500000000000000000 ) ) ;
#19807=EDGE_CURVE ( 'NONE', #19911, #5263, #6257, .T. ) ;
#19808=CYLINDRICAL_SURFACE ( 'NONE', #16243, 0.5000000000000002220 ) ;
#19824=CARTESIAN_POINT ( 'NONE',  ( 30.91344420362545975, -3.401318489841208326, -2.750000000000000000 ) ) ;
#19826=VERTEX_POINT ( 'NONE', #12357 ) ;
#19834=CARTESIAN_POINT ( 'NONE',  ( 18.28012134629595309, 25.16042852506084770, -6.500000000000000000 ) ) ;
#19835=DIRECTION ( 'NONE',  ( 0.000000000000000000, 0.000000000000000000, 1.000000000000000000 ) ) ;
#19839=ORIENTED_EDGE ( 'NONE', *, *, #8937, .T. ) ;
#19848=LINE ( 'NONE', #887, #5083 ) ;
#19852=EDGE_CURVE ( 'NONE', #18040, #17840, #13359, .T. ) ;
#19854=ORIENTED_EDGE ( 'NONE', *, *, #1541, .F. ) ;
#19855=ADVANCED_FACE ( 'NONE', ( #20198 ), #6473, .T. ) ;
#19857=CARTESIAN_POINT ( 'NONE',  ( -24.66042852506104310, -18.28012134629567598, 1.000000000000000000 ) ) ;
#19859=DIRECTION ( 'NONE',  ( 0.000000000000000000, 0.000000000000000000, 1.000000000000000000 ) ) ;
#19861=CIRCLE ( 'NONE', #12349, 31.10000000000000142 ) ;
#19868=FACE_OUTER_BOUND ( 'NONE', #12334, .T. ) ;
#19873=DIRECTION ( 'NONE',  ( 0.000000000000000000, 0.000000000000000000, 1.000000000000000000 ) ) ;
#19875=DIRECTION ( 'NONE',  ( -0.000000000000000000, -0.000000000000000000, 1.000000000000000000 ) ) ;
#19877=DIRECTION ( 'NONE',  ( 0.000000000000000000, 0.000000000000000000, 1.000000000000000000 ) ) ;
#19881=CARTESIAN_POINT ( 'NONE',  ( 0.000000000000000000, 0.000000000000000000, -6.500000000000000000 ) ) ;
#19885=ORIENTED_EDGE ( 'NONE', *, *, #18494, .F. ) ;
#19902=VERTEX_POINT ( 'NONE', #14459 ) ;
#19911=VERTEX_POINT ( 'NONE', #16433 ) ;
#19917=FACE_OUTER_BOUND ( 'NONE', #6285, .T. ) ;
#19918=DIRECTION ( 'NONE',  ( -0.7289686274214034478, 0.6845471059286972748, 0.000000000000000000 ) ) ;
#19921=EDGE_CURVE ( 'NONE', #11648, #7998, #5011, .T. ) ;
#19925=CARTESIAN_POINT ( 'NONE',  ( 0.000000000000000000, 0.000000000000000000, 1.000000000000000000 ) ) ;
#19927=DIRECTION ( 'NONE',  ( 1.000000000000000000, 0.000000000000000000, 0.000000000000000000 ) ) ;
#19931=AXIS2_PLACEMENT_3D ( 'NONE', #5339, #21675, #3760 ) ;
#19933=DIRECTION ( 'NONE',  ( 0.000000000000000000, 0.000000000000000000, 1.000000000000000000 ) ) ;
#19938=ORIENTED_EDGE ( 'NONE', *, *, #539, .T. ) ;
#19941=DIRECTION ( 'NONE',  ( 0.000000000000000000, 0.000000000000000000, 1.000000000000000000 ) ) ;
#19942=DIRECTION ( 'NONE',  ( 0.000000000000000000, 0.000000000000000000, 1.000000000000000000 ) ) ;
#19944=VERTEX_POINT ( 'NONE', #20727 ) ;
#19946=CARTESIAN_POINT ( 'NONE',  ( 6.317933499823313426, 30.45149776762729843, 1.000000000000000000 ) ) ;
#19948=EDGE_CURVE ( 'NONE', #10075, #15562, #18356, .T. ) ;
#19951=AXIS2_PLACEMENT_3D ( 'NONE', #17924, #3666, #11644 ) ;
#19952=DIRECTION ( 'NONE',  ( -0.000000000000000000, -0.000000000000000000, 1.000000000000000000 ) ) ;
#19953=CARTESIAN_POINT ( 'NONE',  ( -13.69242354489114177, 27.92360179968391165, 1.000000000000000000 ) ) ;
#19956=AXIS2_PLACEMENT_3D ( 'NONE', #7081, #25513, #9433 ) ;
#19957=CARTESIAN_POINT ( 'NONE',  ( -18.28012134629558716, 25.16042852506110705, -6.500000000000000000 ) ) ;
#19958=FACE_OUTER_BOUND ( 'NONE', #6095, .T. ) ;
#19963=CARTESIAN_POINT ( 'NONE',  ( -27.25313774936430633, -14.98253926456308172, -6.500000000000000000 ) ) ;
#19968=VERTEX_POINT ( 'NONE', #25035 ) ;
#19971=DIRECTION ( 'NONE',  ( 0.000000000000000000, 0.000000000000000000, 1.000000000000000000 ) ) ;
#19973=ORIENTED_EDGE ( 'NONE', *, *, #10506, .F. ) ;
#19976=ORIENTED_EDGE ( 'NONE', *, *, #17786, .F. ) ;
#19977=CIRCLE ( 'NONE', #15815, 0.5000000000000001110 ) ;
#19978=EDGE_LOOP ( 'NONE', ( #17779, #553, #163, #17327 ) ) ;
#19979=DIRECTION ( 'NONE',  ( 0.000000000000000000, 0.000000000000000000, 1.000000000000000000 ) ) ;
#19981=EDGE_CURVE ( 'NONE', #19352, #19279, #13262, .T. ) ;
#19983=DIRECTION ( 'NONE',  ( 0.000000000000000000, 0.000000000000000000, 1.000000000000000000 ) ) ;
#19986=DIRECTION ( 'NONE',  ( 0.9510565162951586382, 0.3090169943749320192, 0.000000000000000000 ) ) ;
#19989=CARTESIAN_POINT ( 'NONE',  ( 27.00874656207304980, 15.41874213889405176, 1.000000000000000000 ) ) ;
#19993=AXIS2_PLACEMENT_3D ( 'NONE', #16936, #11035, #9207 ) ;
#19994=DIRECTION ( 'NONE',  ( -0.8443279255020205154, -0.5358267949789882190, 0.000000000000000000 ) ) ;
#19996=EDGE_CURVE ( 'NONE', #22681, #1345, #8965, .T. ) ;
#20000=AXIS2_PLACEMENT_3D ( 'NONE', #24519, #10262, #14588 ) ;
#20002=CIRCLE ( 'NONE', #2465, 31.10000000000000142 ) ;
#20005=ORIENTED_EDGE ( 'NONE', *, *, #2230, .T. ) ;
#20008=ORIENTED_EDGE ( 'NONE', *, *, #15761, .F. ) ;
#20011=ORIENTED_EDGE ( 'NONE', *, *, #7865, .F. ) ;
#20012=EDGE_CURVE ( 'NONE', #2636, #19518, #8758, .T. ) ;
#20013=ORIENTED_EDGE ( 'NONE', *, *, #21664, .F. ) ;
#20017=CIRCLE ( 'NONE', #22113, 0.5000000000000003331 ) ;
#20018=ORIENTED_EDGE ( 'NONE', *, *, #16538, .T. ) ;
#20019=FACE_OUTER_BOUND ( 'NONE', #22923, .T. ) ;
#20021=AXIS2_PLACEMENT_3D ( 'NONE', #4240, #6463, #12219 ) ;
#20022=DIRECTION ( 'NONE',  ( 0.000000000000000000, 0.000000000000000000, 1.000000000000000000 ) ) ;
#20023=DIRECTION ( 'NONE',  ( -0.2486898871648449971, 0.9685831611286336296, 0.000000000000000000 ) ) ;
#20030=EDGE_CURVE ( 'NONE', #2880, #672, #19405, .T. ) ;
#20033=CIRCLE ( 'NONE', #838, 0.5000000000000003331 ) ;
#20037=LINE ( 'NONE', #25677, #1587 ) ;
#20038=EDGE_LOOP ( 'NONE', ( #13687, #16382, #5210, #17248 ) ) ;
#20039=ORIENTED_EDGE ( 'NONE', *, *, #14360, .T. ) ;
#20042=DIRECTION ( 'NONE',  ( 0.000000000000000000, 0.000000000000000000, 1.000000000000000000 ) ) ;
#20044=DIRECTION ( 'NONE',  ( 1.000000000000000000, 0.000000000000000000, 0.000000000000000000 ) ) ;
#20046=ORIENTED_EDGE ( 'NONE', *, *, #10422, .T. ) ;
#20047=CARTESIAN_POINT ( 'NONE',  ( -9.110428525061097460, -29.57785765677920509, 1.000000000000000000 ) ) ;
#20049=DIRECTION ( 'NONE',  ( 1.000000000000000000, 0.000000000000000000, 0.000000000000000000 ) ) ;
#20052=AXIS2_PLACEMENT_3D ( 'NONE', #2235, #1968, #10192 ) ;
#20055=CARTESIAN_POINT ( 'NONE',  ( -9.110428525060477511, 29.57785765677940404, -6.500000000000000000 ) ) ;
#20057=ADVANCED_FACE ( 'NONE', ( #23202 ), #8831, .F. ) ;
#20059=EDGE_CURVE ( 'NONE', #21505, #6156, #4991, .T. ) ;
#20062=CARTESIAN_POINT ( 'NONE',  ( 0.000000000000000000, -31.10000000000000142, -6.500000000000000000 ) ) ;
#20063=LINE ( 'NONE', #10130, #24583 ) ;
#20065=DIRECTION ( 'NONE',  ( -0.000000000000000000, -0.000000000000000000, 1.000000000000000000 ) ) ;
#20066=CARTESIAN_POINT ( 'NONE',  ( 17.87326343783925253, -25.45105997952931176, -2.750000000000000000 ) ) ;
#20067=ADVANCED_FACE ( 'NONE', ( #20851 ), #15353, .T. ) ;
#20069=CIRCLE ( 'NONE', #8811, 0.5000000000000005551 ) ;
#20071=CIRCLE ( 'NONE', #9646, 0.5000000000000006661 ) ;
#20073=EDGE_LOOP ( 'NONE', ( #4546, #25496, #817, #23437 ) ) ;
#20076=VERTEX_POINT ( 'NONE', #9214 ) ;
#20081=DIRECTION ( 'NONE',  ( 1.000000000000000000, 0.000000000000000000, 0.000000000000000000 ) ) ;
#20083=ORIENTED_EDGE ( 'NONE', *, *, #19066, .F. ) ;
#20091=EDGE_CURVE ( 'NONE', #21352, #19826, #19019, .T. ) ;
#20095=CARTESIAN_POINT ( 'NONE',  ( 30.54913349766219710, -5.827558883616158703, -6.500000000000000000 ) ) ;
#20097=CARTESIAN_POINT ( 'NONE',  ( 0.000000000000000000, 0.000000000000000000, -6.500000000000000000 ) ) ;
#20098=DIRECTION ( 'NONE',  ( 0.3681245526846732008, -0.9297764858882532346, 0.000000000000000000 ) ) ;
#20099=DIRECTION ( 'NONE',  ( 1.000000000000000000, 0.000000000000000000, 0.000000000000000000 ) ) ;
#20101=ORIENTED_EDGE ( 'NONE', *, *, #23227, .F. ) ;
#20102=FACE_OUTER_BOUND ( 'NONE', #25621, .T. ) ;
#20105=CARTESIAN_POINT ( 'NONE',  ( -30.85476721088030061, -3.897863563849544466, -6.500000000000000000 ) ) ;
#20109=VERTEX_POINT ( 'NONE', #21112 ) ;
#20110=CYLINDRICAL_SURFACE ( 'NONE', #23867, 31.10000000000000142 ) ;
#20114=EDGE_LOOP ( 'NONE', ( #9473, #23947, #1272, #24004 ) ) ;
#20115=CIRCLE ( 'NONE', #22633, 0.5000000000000003331 ) ;
#20118=ORIENTED_EDGE ( 'NONE', *, *, #1898, .T. ) ;
#20120=CARTESIAN_POINT ( 'NONE',  ( -5.327558883616270613, -30.54913349766217934, 1.000000000000000000 ) ) ;
#20121=CIRCLE ( 'NONE', #10505, 31.10000000000000142 ) ;
#20127=CIRCLE ( 'NONE', #18894, 31.10000000000000142 ) ;
#20129=CIRCLE ( 'NONE', #22229, 0.4999999999999999445 ) ;
#20130=DIRECTION ( 'NONE',  ( -0.9980267284282710039, 0.06279051952932233893, 0.000000000000000000 ) ) ;
#20131=CARTESIAN_POINT ( 'NONE',  ( 20.92219106202050583, 23.01025686871638598, 1.000000000000000000 ) ) ;
#20135=DIRECTION ( 'NONE',  ( 0.000000000000000000, 0.000000000000000000, 1.000000000000000000 ) ) ;
#20137=AXIS2_PLACEMENT_3D ( 'NONE', #8211, #10165, #15937 ) ;
#20138=CARTESIAN_POINT ( 'NONE',  ( -11.44867358849309547, 28.91604871112477326, 1.000000000000000000 ) ) ;
#20139=CARTESIAN_POINT ( 'NONE',  ( 0.000000000000000000, 0.000000000000000000, -6.500000000000000000 ) ) ;
#20143=ORIENTED_EDGE ( 'NONE', *, *, #23166, .F. ) ;
#20145=FACE_OUTER_BOUND ( 'NONE', #12201, .T. ) ;
#20148=CIRCLE ( 'NONE', #24339, 0.4999999999999998335 ) ;
#20150=VERTEX_POINT ( 'NONE', #15746 ) ;
#20157=AXIS2_PLACEMENT_3D ( 'NONE', #6550, #5495, #7208 ) ;
#20159=CARTESIAN_POINT ( 'NONE',  ( 30.10000000000000142, 0.000000000000000000, 0.000000000000000000 ) ) ;
#20161=LINE ( 'NONE', #10477, #7972 ) ;
#20164=EDGE_CURVE ( 'NONE', #17619, #13787, #4087, .T. ) ;
#20168=DIRECTION ( 'NONE',  ( 1.000000000000000000, 0.000000000000000000, 0.000000000000000000 ) ) ;
#20169=CYLINDRICAL_SURFACE ( 'NONE', #8687, 0.4999999999999995559 ) ;
#20171=ORIENTED_EDGE ( 'NONE', *, *, #9208, .T. ) ;
#20175=DIRECTION ( 'NONE',  ( -0.9685831611286283005, 0.2486898871648657861, 0.000000000000000000 ) ) ;
#20176=ORIENTED_EDGE ( 'NONE', *, *, #2762, .F. ) ;
#20178=ORIENTED_EDGE ( 'NONE', *, *, #422, .T. ) ;
#20181=ORIENTED_EDGE ( 'NONE', *, *, #16240, .T. ) ;
#20187=CYLINDRICAL_SURFACE ( 'NONE', #403, 31.10000000000000142 ) ;
#20192=AXIS2_PLACEMENT_3D ( 'NONE', #21126, #23215, #5429 ) ;
#20193=LINE ( 'NONE', #3422, #13316 ) ;
#20198=FACE_OUTER_BOUND ( 'NONE', #17778, .T. ) ;
#20203=EDGE_LOOP ( 'NONE', ( #9444, #1733, #5973, #22771 ) ) ;
#20204=ORIENTED_EDGE ( 'NONE', *, *, #23591, .T. ) ;
#20206=MECHANICAL_DESIGN_GEOMETRIC_PRESENTATION_REPRESENTATION('',(#3510),#595);
#20208=CARTESIAN_POINT ( 'NONE',  ( 0.000000000000000000, 0.000000000000000000, -6.500000000000000000 ) ) ;
#20209=ORIENTED_EDGE ( 'NONE', *, *, #6190, .T. ) ;
#20210=VERTEX_POINT ( 'NONE', #15625 ) ;
#20211=EDGE_CURVE ( 'NONE', #10774, #6810, #21694, .T. ) ;
#20215=ADVANCED_FACE ( 'NONE', ( #17446 ), #23593, .T. ) ;
#20217=EDGE_CURVE ( 'NONE', #12173, #19269, #13918, .T. ) ;
#20221=CARTESIAN_POINT ( 'NONE',  ( 0.000000000000000000, 0.000000000000000000, 1.000000000000000000 ) ) ;
#20223=ADVANCED_FACE ( 'NONE', ( #6061 ), #19657, .F. ) ;
#20230=DIRECTION ( 'NONE',  ( -0.000000000000000000, -0.000000000000000000, 1.000000000000000000 ) ) ;
#20233=ORIENTED_EDGE ( 'NONE', *, *, #15211, .F. ) ;
#20243=VECTOR ( 'NONE', #7771, 1000.000000000000000 ) ;
#20245=ORIENTED_EDGE ( 'NONE', *, *, #11594, .T. ) ;
#20246=DIRECTION ( 'NONE',  ( 0.000000000000000000, -0.000000000000000000, 1.000000000000000000 ) ) ;
#20248=EDGE_CURVE ( 'NONE', #4968, #2690, #14599, .T. ) ;
#20249=DIRECTION ( 'NONE',  ( 0.000000000000000000, -0.000000000000000000, 1.000000000000000000 ) ) ;
#20254=EDGE_CURVE ( 'NONE', #18582, #25179, #9852, .T. ) ;
#20256=DIRECTION ( 'NONE',  ( 0.000000000000000000, 0.000000000000000000, 1.000000000000000000 ) ) ;
#20258=DIRECTION ( 'NONE',  ( 0.000000000000000000, 0.000000000000000000, 1.000000000000000000 ) ) ;
#20266=VERTEX_POINT ( 'NONE', #10349 ) ;
#20269=ORIENTED_EDGE ( 'NONE', *, *, #17042, .F. ) ;
#20271=ORIENTED_EDGE ( 'NONE', *, *, #10247, .T. ) ;
#20272=ORIENTED_EDGE ( 'NONE', *, *, #23591, .F. ) ;
#20274=ORIENTED_EDGE ( 'NONE', *, *, #1250, .F. ) ;
#20275=DIRECTION ( 'NONE',  ( 1.000000000000000000, 0.000000000000000000, 0.000000000000000000 ) ) ;
#20277=VERTEX_POINT ( 'NONE', #14316 ) ;
#20283=CARTESIAN_POINT ( 'NONE',  ( 0.000000000000000000, 0.000000000000000000, 1.000000000000000000 ) ) ;
#20290=DIRECTION ( 'NONE',  ( 0.000000000000000000, 0.000000000000000000, 1.000000000000000000 ) ) ;
#20294=DIRECTION ( 'NONE',  ( 0.000000000000000000, 0.000000000000000000, 1.000000000000000000 ) ) ;
#20295=DIRECTION ( 'NONE',  ( -0.000000000000000000, -0.000000000000000000, 1.000000000000000000 ) ) ;
#20302=CARTESIAN_POINT ( 'NONE',  ( 18.68225429291714690, -24.86329371854781201, -6.500000000000000000 ) ) ;
#20304=CARTESIAN_POINT ( 'NONE',  ( 23.64116323484238080, 20.20656826142275264, 1.000000000000000000 ) ) ;
#20305=ORIENTED_EDGE ( 'NONE', *, *, #21306, .F. ) ;
#20308=FACE_OUTER_BOUND ( 'NONE', #25083, .T. ) ;
#20313=EDGE_CURVE ( 'NONE', #4940, #10460, #7502, .T. ) ;
#20315=EDGE_CURVE ( 'NONE', #17398, #13890, #25463, .T. ) ;
#20320=DIRECTION ( 'NONE',  ( 0.000000000000000000, 0.000000000000000000, 1.000000000000000000 ) ) ;
#20321=AXIS2_PLACEMENT_3D ( 'NONE', #10002, #20320, #24510 ) ;
#20324=ORIENTED_EDGE ( 'NONE', *, *, #20821, .F. ) ;
#20329=EDGE_LOOP ( 'NONE', ( #17888, #21108, #13657, #8096 ) ) ;
#20330=CARTESIAN_POINT ( 'NONE',  ( -7.248980000273768098, 30.24338421796792176, -2.750000000000000000 ) ) ;
#20338=CARTESIAN_POINT ( 'NONE',  ( 0.000000000000000000, 0.000000000000000000, 1.000000000000000000 ) ) ;
#20339=EDGE_CURVE ( 'NONE', #25113, #10289, #2033, .T. ) ;
#20340=CARTESIAN_POINT ( 'NONE',  ( 7.734255490827002255, 30.12293631110042469, 1.000000000000000000 ) ) ;
#20342=CARTESIAN_POINT ( 'NONE',  ( 6.317933499823437771, 30.45149776762727356, -2.750000000000000000 ) ) ;
#20343=DIRECTION ( 'NONE',  ( 0.000000000000000000, 0.000000000000000000, 1.000000000000000000 ) ) ;
#20352=EDGE_CURVE ( 'NONE', #12237, #24819, #5779, .T. ) ;
#20356=CARTESIAN_POINT ( 'NONE',  ( 24.27856662945494293, -19.43607991388997291, -2.750000000000000000 ) ) ;
#20367=CARTESIAN_POINT ( 'NONE',  ( -31.03863125411927371, -1.952785157361310198, -6.500000000000000000 ) ) ;
#20370=CARTESIAN_POINT ( 'NONE',  ( -16.16421332384701515, -26.25859848311253941, 1.000000000000000000 ) ) ;
#20376=ADVANCED_FACE ( 'NONE', ( #16406 ), #12333, .F. ) ;
#20378=CARTESIAN_POINT ( 'NONE',  ( 0.000000000000000000, 0.000000000000000000, 1.000000000000000000 ) ) ;
#20383=EDGE_CURVE ( 'NONE', #7744, #11788, #22532, .T. ) ;
#20385=AXIS2_PLACEMENT_3D ( 'NONE', #15293, #923, #10838 ) ;
#20386=DIRECTION ( 'NONE',  ( 0.000000000000000000, 0.000000000000000000, 1.000000000000000000 ) ) ;
#20390=DIRECTION ( 'NONE',  ( 1.000000000000000000, 0.000000000000000000, 0.000000000000000000 ) ) ;
#20393=VECTOR ( 'NONE', #5341, 1000.000000000000000 ) ;
#20395=ORIENTED_EDGE ( 'NONE', *, *, #17247, .F. ) ;
#20396=ORIENTED_EDGE ( 'NONE', *, *, #25360, .T. ) ;
#20397=ORIENTED_EDGE ( 'NONE', *, *, #5478, .F. ) ;
#20398=CARTESIAN_POINT ( 'NONE',  ( -21.28941499438242246, -22.67092431280570963, 1.000000000000000000 ) ) ;
#20399=ORIENTED_EDGE ( 'NONE', *, *, #22417, .F. ) ;
#20404=AXIS2_PLACEMENT_3D ( 'NONE', #2705, #4670, #18657 ) ;
#20407=DIRECTION ( 'NONE',  ( 0.000000000000000000, 0.000000000000000000, 1.000000000000000000 ) ) ;
#20413=ADVANCED_FACE ( 'NONE', ( #22142 ), #4761, .F. ) ;
#20422=EDGE_CURVE ( 'NONE', #14523, #2078, #22496, .T. ) ;
#20424=DIRECTION ( 'NONE',  ( 0.000000000000000000, 0.000000000000000000, 1.000000000000000000 ) ) ;
#20425=ORIENTED_EDGE ( 'NONE', *, *, #7444, .T. ) ;
#20426=CARTESIAN_POINT ( 'NONE',  ( 0.000000000000000000, 0.000000000000000000, 1.000000000000000000 ) ) ;
#20429=AXIS2_PLACEMENT_3D ( 'NONE', #10215, #24083, #11804 ) ;
#20430=EDGE_CURVE ( 'NONE', #9082, #8835, #11207, .T. ) ;
#20431=CYLINDRICAL_SURFACE ( 'NONE', #16955, 0.5000000000000004441 ) ;
#20432=AXIS2_PLACEMENT_3D ( 'NONE', #20452, #20597, #8305 ) ;
#20434=CARTESIAN_POINT ( 'NONE',  ( 27.00874656207304980, 15.41874213889405176, -6.500000000000000000 ) ) ;
#20437=CARTESIAN_POINT ( 'NONE',  ( -25.75859848311282363, -16.66421332384654974, 1.000000000000000000 ) ) ;
#20439=CARTESIAN_POINT ( 'NONE',  ( 0.000000000000000000, 0.000000000000000000, 1.000000000000000000 ) ) ;
#20440=CARTESIAN_POINT ( 'NONE',  ( 0.000000000000000000, 0.000000000000000000, -6.500000000000000000 ) ) ;
#20443=CIRCLE ( 'NONE', #19191, 0.5000000000000011102 ) ;
#20444=AXIS2_PLACEMENT_3D ( 'NONE', #757, #14883, #9111 ) ;
#20447=DIRECTION ( 'NONE',  ( 0.000000000000000000, 0.000000000000000000, 1.000000000000000000 ) ) ;
#20451=EDGE_CURVE ( 'NONE', #4678, #4202, #23800, .T. ) ;
#20452=CARTESIAN_POINT ( 'NONE',  ( -3.897863563850083146, -30.85476721088024021, -6.500000000000000000 ) ) ;
#20453=AXIS2_PLACEMENT_3D ( 'NONE', #21380, #5796, #3704 ) ;
#20454=VERTEX_POINT ( 'NONE', #25007 ) ;
#20458=ORIENTED_EDGE ( 'NONE', *, *, #17316, .T. ) ;
#20461=AXIS2_PLACEMENT_3D ( 'NONE', #7461, #23286, #19755 ) ;
#20463=DIRECTION ( 'NONE',  ( 0.000000000000000000, 0.000000000000000000, 1.000000000000000000 ) ) ;
#20471=VECTOR ( 'NONE', #25129, 1000.000000000000000 ) ;
#20473=ADVANCED_FACE ( 'NONE', ( #1347 ), #3290, .F. ) ;
#20474=AXIS2_PLACEMENT_3D ( 'NONE', #14947, #17039, #7233 ) ;
#20478=AXIS2_PLACEMENT_3D ( 'NONE', #24568, #20658, #19074 ) ;
#20481=DIRECTION ( 'NONE',  ( 1.000000000000000000, 0.000000000000000000, 0.000000000000000000 ) ) ;
#20482=LINE ( 'NONE', #12778, #11205 ) ;
#20484=EDGE_CURVE ( 'NONE', #19902, #16230, #4946, .T. ) ;
#20486=VECTOR ( 'NONE', #19666, 1000.000000000000000 ) ;
#20488=CARTESIAN_POINT ( 'NONE',  ( -13.24173596767398742, -28.14012133169310559, -6.500000000000000000 ) ) ;
#20492=VERTEX_POINT ( 'NONE', #2782 ) ;
#20497=DIRECTION ( 'NONE',  ( -0.2486898871648449971, 0.9685831611286336296, 0.000000000000000000 ) ) ;
#20499=CARTESIAN_POINT ( 'NONE',  ( 21.28941499438225904, 22.67092431280586240, 1.000000000000000000 ) ) ;
#20500=VERTEX_POINT ( 'NONE', #19249 ) ;
#20503=AXIS2_PLACEMENT_3D ( 'NONE', #8170, #19532, #20712 ) ;
#20507=ORIENTED_EDGE ( 'NONE', *, *, #20030, .T. ) ;
#20508=EDGE_CURVE ( 'NONE', #7703, #25247, #4524, .T. ) ;
#20509=DIRECTION ( 'NONE',  ( 0.000000000000000000, 0.000000000000000000, 1.000000000000000000 ) ) ;
#20510=VECTOR ( 'NONE', #17091, 1000.000000000000000 ) ;
#20512=VECTOR ( 'NONE', #11353, 1000.000000000000000 ) ;
#20513=CARTESIAN_POINT ( 'NONE',  ( -17.78012134629613783, -25.16042852506070560, -6.500000000000000000 ) ) ;
#20515=AXIS2_PLACEMENT_3D ( 'NONE', #742, #10793, #4525 ) ;
#20518=CARTESIAN_POINT ( 'NONE',  ( 30.24338421796784004, 7.248980000274092284, -6.500000000000000000 ) ) ;
#20522=CARTESIAN_POINT ( 'NONE',  ( 0.000000000000000000, 0.000000000000000000, -6.500000000000000000 ) ) ;
#20526=CARTESIAN_POINT ( 'NONE',  ( -30.24338421796775123, 7.248980000274508839, 1.000000000000000000 ) ) ;
#20530=CARTESIAN_POINT ( 'NONE',  ( 20.20656826142283435, 23.64116323484230975, -2.750000000000000000 ) ) ;
#20537=ORIENTED_EDGE ( 'NONE', *, *, #17726, .T. ) ;
#20541=ORIENTED_EDGE ( 'NONE', *, *, #10839, .F. ) ;
#20542=ORIENTED_EDGE ( 'NONE', *, *, #1541, .T. ) ;
#20543=ORIENTED_EDGE ( 'NONE', *, *, #24716, .F. ) ;
#20545=CIRCLE ( 'NONE', #23455, 0.5000000000000011102 ) ;
#20547=EDGE_CURVE ( 'NONE', #20076, #24433, #7102, .T. ) ;
#20548=CARTESIAN_POINT ( 'NONE',  ( 16.66421332384664566, -26.25859848311276679, -6.500000000000000000 ) ) ;
#20550=CIRCLE ( 'NONE', #23894, 31.10000000000000142 ) ;
#20556=AXIS2_PLACEMENT_3D ( 'NONE', #4516, #10535, #7270 ) ;
#20561=DIRECTION ( 'NONE',  ( 0.000000000000000000, 0.000000000000000000, 1.000000000000000000 ) ) ;
#20564=CYLINDRICAL_SURFACE ( 'NONE', #9645, 0.5000000000000004441 ) ;
#20566=DIRECTION ( 'NONE',  ( 0.000000000000000000, 0.000000000000000000, 1.000000000000000000 ) ) ;
#20567=AXIS2_PLACEMENT_3D ( 'NONE', #9157, #19218, #17016 ) ;
#20568=ORIENTED_EDGE ( 'NONE', *, *, #4253, .F. ) ;
#20572=ORIENTED_EDGE ( 'NONE', *, *, #3464, .F. ) ;
#20573=DIRECTION ( 'NONE',  ( -0.1873813145857119722, 0.9822872507286911636, 0.000000000000000000 ) ) ;
#20576=VERTEX_POINT ( 'NONE', #3049 ) ;
#20578=CARTESIAN_POINT ( 'NONE',  ( 0.000000000000000000, 0.000000000000000000, 1.000000000000000000 ) ) ;
#20588=AXIS2_PLACEMENT_3D ( 'NONE', #17005, #1050, #17274 ) ;
#20590=EDGE_CURVE ( 'NONE', #8694, #16529, #22964, .T. ) ;
#20592=CIRCLE ( 'NONE', #20157, 31.10000000000000142 ) ;
#20595=CARTESIAN_POINT ( 'NONE',  ( 25.98730014090430274, -17.08421000182786997, -2.750000000000000000 ) ) ;
#20597=DIRECTION ( 'NONE',  ( 0.000000000000000000, 0.000000000000000000, 1.000000000000000000 ) ) ;
#20598=VERTEX_POINT ( 'NONE', #1203 ) ;
#20607=ORIENTED_EDGE ( 'NONE', *, *, #1178, .F. ) ;
#20612=VECTOR ( 'NONE', #25371, 1000.000000000000000 ) ;
#20615=AXIS2_PLACEMENT_3D ( 'NONE', #6910, #20904, #2993 ) ;
#20617=DIRECTION ( 'NONE',  ( 1.000000000000000000, 0.000000000000000000, 0.000000000000000000 ) ) ;
#20619=CARTESIAN_POINT ( 'NONE',  ( -30.53863125411927371, -1.952785157361310198, -6.500000000000000000 ) ) ;
#20621=CARTESIAN_POINT ( 'NONE',  ( 2.451530025009009961, 31.00322564728515218, 1.000000000000000000 ) ) ;
#20629=VERTEX_POINT ( 'NONE', #17936 ) ;
#20634=CARTESIAN_POINT ( 'NONE',  ( 19.43607991388988765, 24.27856662945500688, -6.500000000000000000 ) ) ;
#20639=DIRECTION ( 'NONE',  ( 0.000000000000000000, 0.000000000000000000, 1.000000000000000000 ) ) ;
#20640=ORIENTED_EDGE ( 'NONE', *, *, #5876, .T. ) ;
#20645=CARTESIAN_POINT ( 'NONE',  ( -7.248980000274416469, -30.24338421796776544, 1.000000000000000000 ) ) ;
#20647=CYLINDRICAL_SURFACE ( 'NONE', #6004, 0.5000000000000002220 ) ;
#20649=EDGE_CURVE ( 'NONE', #7097, #14349, #11625, .T. ) ;
#20658=DIRECTION ( 'NONE',  ( -0.000000000000000000, -0.000000000000000000, 1.000000000000000000 ) ) ;
#20659=DIRECTION ( 'NONE',  ( -0.000000000000000000, -0.000000000000000000, 1.000000000000000000 ) ) ;
#20661=EDGE_CURVE ( 'NONE', #8766, #6385, #19629, .T. ) ;
#20663=CYLINDRICAL_SURFACE ( 'NONE', #18601, 0.5000000000000004441 ) ;
#20665=CARTESIAN_POINT ( 'NONE',  ( 0.000000000000000000, 0.000000000000000000, 1.000000000000000000 ) ) ;
#20668=EDGE_CURVE ( 'NONE', #11918, #14407, #9123, .T. ) ;
#20671=ORIENTED_EDGE ( 'NONE', *, *, #19751, .F. ) ;
#20675=ORIENTED_EDGE ( 'NONE', *, *, #20254, .T. ) ;
#20676=CARTESIAN_POINT ( 'NONE',  ( -30.63887302793249034, -5.335677986744600254, 1.000000000000000000 ) ) ;
#20677=ORIENTED_EDGE ( 'NONE', *, *, #3735, .T. ) ;
#20678=FACE_OUTER_BOUND ( 'NONE', #2340, .T. ) ;
#20681=CARTESIAN_POINT ( 'NONE',  ( 3.401318489840878367, -30.91344420362549528, -2.750000000000000000 ) ) ;
#20684=DIRECTION ( 'NONE',  ( 0.000000000000000000, 0.000000000000000000, 1.000000000000000000 ) ) ;
#20685=AXIS2_PLACEMENT_3D ( 'NONE', #10836, #7432, #17269 ) ;
#20688=CARTESIAN_POINT ( 'NONE',  ( 13.24173596767378847, 28.14012133169319796, 1.000000000000000000 ) ) ;
#20691=DIRECTION ( 'NONE',  ( 1.000000000000000000, 0.000000000000000000, 0.000000000000000000 ) ) ;
#20694=DIRECTION ( 'NONE',  ( 0.000000000000000000, 0.000000000000000000, 1.000000000000000000 ) ) ;
#20696=EDGE_CURVE ( 'NONE', #14918, #22793, #13782, .T. ) ;
#20701=DIRECTION ( 'NONE',  ( 0.000000000000000000, 0.000000000000000000, 1.000000000000000000 ) ) ;
#20703=AXIS2_PLACEMENT_3D ( 'NONE', #7508, #25689, #17587 ) ;
#20707=ORIENTED_EDGE ( 'NONE', *, *, #18886, .F. ) ;
#20708=CIRCLE ( 'NONE', #14030, 31.10000000000000142 ) ;
#20709=DIRECTION ( 'NONE',  ( 0.000000000000000000, 0.000000000000000000, 1.000000000000000000 ) ) ;
#20712=DIRECTION ( 'NONE',  ( -0.3090169943749382919, 0.9510565162951566398, 0.000000000000000000 ) ) ;
#20715=VECTOR ( 'NONE', #1704, 1000.000000000000000 ) ;
#20718=CARTESIAN_POINT ( 'NONE',  ( -21.65113613650310143, 22.32573188046944068, 1.000000000000000000 ) ) ;
#20719=ADVANCED_FACE ( 'NONE', ( #21864 ), #17689, .T. ) ;
#20720=ORIENTED_EDGE ( 'NONE', *, *, #15130, .T. ) ;
#20726=ADVANCED_FACE ( 'NONE', ( #23684 ), #21480, .T. ) ;
#20727=CARTESIAN_POINT ( 'NONE',  ( -29.62293631110035363, 7.734255490827311341, -6.500000000000000000 ) ) ;
#20736=EDGE_CURVE ( 'NONE', #1055, #2880, #2438, .T. ) ;
#20746=DIRECTION ( 'NONE',  ( 0.000000000000000000, 0.000000000000000000, 1.000000000000000000 ) ) ;
#20747=DIRECTION ( 'NONE',  ( 1.000000000000000000, 0.000000000000000000, 0.000000000000000000 ) ) ;
#20749=DIRECTION ( 'NONE',  ( -0.000000000000000000, -0.000000000000000000, 1.000000000000000000 ) ) ;
#20753=EDGE_CURVE ( 'NONE', #9464, #161, #21729, .T. ) ;
#20754=CYLINDRICAL_SURFACE ( 'NONE', #19663, 0.5000000000000004441 ) ;
#20764=ORIENTED_EDGE ( 'NONE', *, *, #12864, .F. ) ;
#20768=ORIENTED_EDGE ( 'NONE', *, *, #13212, .T. ) ;
#20770=ORIENTED_EDGE ( 'NONE', *, *, #4364, .F. ) ;
#20772=CARTESIAN_POINT ( 'NONE',  ( 14.54246377227351061, -27.49048467073857793, 1.000000000000000000 ) ) ;
#20784=CARTESIAN_POINT ( 'NONE',  ( 31.10000000000000142, -1.085850696380214537E-13, 1.000000000000000000 ) ) ;
#20790=ORIENTED_EDGE ( 'NONE', *, *, #12495, .T. ) ;
#20791=DIRECTION ( 'NONE',  ( 0.000000000000000000, 0.000000000000000000, 1.000000000000000000 ) ) ;
#20793=ORIENTED_EDGE ( 'NONE', *, *, #17195, .F. ) ;
#20796=CIRCLE ( 'NONE', #802, 0.5000000000000002220 ) ;
#20797=VERTEX_POINT ( 'NONE', #10684 ) ;
#20799=ORIENTED_EDGE ( 'NONE', *, *, #2796, .F. ) ;
#20803=ORIENTED_EDGE ( 'NONE', *, *, #16538, .F. ) ;
#20811=AXIS2_PLACEMENT_3D ( 'NONE', #24093, #22134, #10487 ) ;
#20815=CARTESIAN_POINT ( 'NONE',  ( 0.000000000000000000, 0.000000000000000000, -6.500000000000000000 ) ) ;
#20821=EDGE_CURVE ( 'NONE', #13301, #20277, #14991, .T. ) ;
#20829=EDGE_LOOP ( 'NONE', ( #7299, #19284, #5676, #9878 ) ) ;
#20835=AXIS2_PLACEMENT_3D ( 'NONE', #5177, #21117, #17211 ) ;
#20846=AXIS2_PLACEMENT_3D ( 'NONE', #3215, #2973, #8719 ) ;
#20851=FACE_OUTER_BOUND ( 'NONE', #1207, .T. ) ;
#20855=ORIENTED_EDGE ( 'NONE', *, *, #23843, .T. ) ;
#20857=CARTESIAN_POINT ( 'NONE',  ( 0.000000000000000000, 0.000000000000000000, -6.500000000000000000 ) ) ;
#20859=CIRCLE ( 'NONE', #25445, 0.5000000000000005551 ) ;
#20860=ORIENTED_EDGE ( 'NONE', *, *, #21994, .F. ) ;
#20863=CARTESIAN_POINT ( 'NONE',  ( 0.000000000000000000, 0.000000000000000000, -6.500000000000000000 ) ) ;
#20864=CIRCLE ( 'NONE', #3739, 0.4999999999999999445 ) ;
#20866=DIRECTION ( 'NONE',  ( -0.000000000000000000, -0.000000000000000000, 1.000000000000000000 ) ) ;
#20868=ADVANCED_FACE ( 'NONE', ( #4061 ), #641, .F. ) ;
#20869=AXIS2_PLACEMENT_3D ( 'NONE', #11087, #1286, #1149 ) ;
#20871=AXIS2_PLACEMENT_3D ( 'NONE', #14581, #18518, #18759 ) ;
#20874=CYLINDRICAL_SURFACE ( 'NONE', #18775, 0.5000000000000004441 ) ;
#20875=EDGE_CURVE ( 'NONE', #3398, #2759, #18334, .T. ) ;
#20882=CARTESIAN_POINT ( 'NONE',  ( -21.28941499438242246, -22.67092431280570963, 1.000000000000000000 ) ) ;
#20885=CIRCLE ( 'NONE', #13372, 0.4999999999999993339 ) ;
#20886=DIRECTION ( 'NONE',  ( 1.000000000000000000, 0.000000000000000000, 0.000000000000000000 ) ) ;
#20889=ORIENTED_EDGE ( 'NONE', *, *, #17323, .F. ) ;
#20890=LINE ( 'NONE', #22601, #23040 ) ;
#20901=DIRECTION ( 'NONE',  ( 1.000000000000000000, 0.000000000000000000, 0.000000000000000000 ) ) ;
#20903=AXIS2_PLACEMENT_3D ( 'NONE', #15916, #25718, #15778 ) ;
#20904=DIRECTION ( 'NONE',  ( 0.000000000000000000, -0.000000000000000000, 1.000000000000000000 ) ) ;
#20905=EDGE_CURVE ( 'NONE', #1309, #23985, #4935, .T. ) ;
#20907=CIRCLE ( 'NONE', #12978, 31.10000000000000142 ) ;
#20910=CARTESIAN_POINT ( 'NONE',  ( 0.000000000000000000, 0.000000000000000000, 1.000000000000000000 ) ) ;
#20912=CIRCLE ( 'NONE', #16763, 0.5000000000000002220 ) ;
#20914=CARTESIAN_POINT ( 'NONE',  ( 0.000000000000000000, 0.000000000000000000, 1.000000000000000000 ) ) ;
#20919=CARTESIAN_POINT ( 'NONE',  ( -23.96296185032681336, 19.82388608118453632, -6.500000000000000000 ) ) ;
#20921=FACE_OUTER_BOUND ( 'NONE', #14628, .T. ) ;
#20925=DIRECTION ( 'NONE',  ( 0.000000000000000000, 0.000000000000000000, 1.000000000000000000 ) ) ;
#20926=EDGE_CURVE ( 'NONE', #19323, #9003, #8877, .T. ) ;
#20927=AXIS2_PLACEMENT_3D ( 'NONE', #956, #11130, #25137 ) ;
#20928=LINE ( 'NONE', #18965, #2894 ) ;
#20929=CARTESIAN_POINT ( 'NONE',  ( -7.234255490827218082, -30.12293631110037140, -6.500000000000000000 ) ) ;
#20930=VERTEX_POINT ( 'NONE', #18941 ) ;
#20932=FACE_OUTER_BOUND ( 'NONE', #13985, .T. ) ;
#20933=VERTEX_POINT ( 'NONE', #8999 ) ;
#20934=AXIS2_PLACEMENT_3D ( 'NONE', #10035, #6114, #8212 ) ;
#20938=ORIENTED_EDGE ( 'NONE', *, *, #10581, .F. ) ;
#20939=VERTEX_POINT ( 'NONE', #24434 ) ;
#20940=CARTESIAN_POINT ( 'NONE',  ( 31.06601413805602618, 1.453535542772499856, -2.750000000000000000 ) ) ;
#20941=CIRCLE ( 'NONE', #15098, 31.10000000000000142 ) ;
#20942=ORIENTED_EDGE ( 'NONE', *, *, #1314, .F. ) ;
#20956=DIRECTION ( 'NONE',  ( -0.5358267949789882190, 0.8443279255020205154, 0.000000000000000000 ) ) ;
#20958=DIRECTION ( 'NONE',  ( 0.06279051952932236669, 0.9980267284282710039, 0.000000000000000000 ) ) ;
#20959=LINE ( 'NONE', #16638, #25539 ) ;
#20964=ORIENTED_EDGE ( 'NONE', *, *, #2578, .F. ) ;
#20966=AXIS2_PLACEMENT_3D ( 'NONE', #21740, #20022, #19778 ) ;
#20967=ORIENTED_EDGE ( 'NONE', *, *, #22768, .T. ) ;
#20969=EDGE_LOOP ( 'NONE', ( #24589, #1227, #21919, #286 ) ) ;
#20973=CIRCLE ( 'NONE', #4245, 31.10000000000000142 ) ;
#20979=AXIS2_PLACEMENT_3D ( 'NONE', #13079, #19077, #16882 ) ;
#20984=CARTESIAN_POINT ( 'NONE',  ( 9.133673601486471227, 29.72853858738282185, -2.750000000000000000 ) ) ;
#20991=ORIENTED_EDGE ( 'NONE', *, *, #5772, .T. ) ;
#20995=DIRECTION ( 'NONE',  ( -0.000000000000000000, -0.000000000000000000, 1.000000000000000000 ) ) ;
#20997=LINE ( 'NONE', #24786, #23402 ) ;
#21000=ORIENTED_EDGE ( 'NONE', *, *, #8327, .T. ) ;
#21001=ORIENTED_EDGE ( 'NONE', *, *, #2302, .T. ) ;
#21002=DIRECTION ( 'NONE',  ( 0.000000000000000000, 0.000000000000000000, 1.000000000000000000 ) ) ;
#21009=AXIS2_PLACEMENT_3D ( 'NONE', #8939, #20065, #16155 ) ;
#21010=CARTESIAN_POINT ( 'NONE',  ( 27.00874656207294322, -15.41874213889423828, -6.500000000000000000 ) ) ;
#21014=PRODUCT_CONTEXT ( 'NONE', #3250, 'mechanical' ) ;
#21016=DIRECTION ( 'NONE',  ( 1.000000000000000000, 0.000000000000000000, 0.000000000000000000 ) ) ;
#21017=AXIS2_PLACEMENT_3D ( 'NONE', #14832, #8808, #3176 ) ;
#21024=DIRECTION ( 'NONE',  ( 1.000000000000000000, 0.000000000000000000, 0.000000000000000000 ) ) ;
#21026=LINE ( 'NONE', #10943, #6291 ) ;
#21031=EDGE_CURVE ( 'NONE', #18048, #9980, #14729, .T. ) ;
#21033=ORIENTED_EDGE ( 'NONE', *, *, #9213, .F. ) ;
#21036=AXIS2_PLACEMENT_3D ( 'NONE', #13353, #15703, #13223 ) ;
#21037=EDGE_LOOP ( 'NONE', ( #8383, #5356, #18004, #24460 ) ) ;
#21039=ORIENTED_EDGE ( 'NONE', *, *, #6317, .F. ) ;
#21040=VERTEX_POINT ( 'NONE', #2559 ) ;
#21047=DIRECTION ( 'NONE',  ( 0.000000000000000000, 0.000000000000000000, 1.000000000000000000 ) ) ;
#21054=CARTESIAN_POINT ( 'NONE',  ( 0.000000000000000000, 0.000000000000000000, -6.500000000000000000 ) ) ;
#21057=FACE_OUTER_BOUND ( 'NONE', #15302, .T. ) ;
#21058=CARTESIAN_POINT ( 'NONE',  ( -17.78012134629613783, -25.16042852506070560, -6.500000000000000000 ) ) ;
#21060=DIRECTION ( 'NONE',  ( 0.000000000000000000, -0.000000000000000000, 1.000000000000000000 ) ) ;
#21061=ORIENTED_EDGE ( 'NONE', *, *, #9720, .F. ) ;
#21064=ORIENTED_EDGE ( 'NONE', *, *, #21233, .F. ) ;
#21065=EDGE_CURVE ( 'NONE', #24237, #15562, #8837, .T. ) ;
#21068=ORIENTED_EDGE ( 'NONE', *, *, #431, .T. ) ;
#21069=VERTEX_POINT ( 'NONE', #18256 ) ;
#21070=CARTESIAN_POINT ( 'NONE',  ( 0.000000000000000000, 0.000000000000000000, -6.500000000000000000 ) ) ;
#21071=DIRECTION ( 'NONE',  ( 0.000000000000000000, 0.000000000000000000, 1.000000000000000000 ) ) ;
#21082=CARTESIAN_POINT ( 'NONE',  ( -24.86329371854747805, 18.68225429291759099, -2.750000000000000000 ) ) ;
#21083=CARTESIAN_POINT ( 'NONE',  ( -31.03863125411922752, 1.952785157361987878, -6.500000000000000000 ) ) ;
#21089=ORIENTED_EDGE ( 'NONE', *, *, #13478, .F. ) ;
#21091=DIRECTION ( 'NONE',  ( 0.000000000000000000, 0.000000000000000000, 1.000000000000000000 ) ) ;
#21094=ORIENTED_EDGE ( 'NONE', *, *, #5804, .T. ) ;
#21095=DIRECTION ( 'NONE',  ( 1.000000000000000000, 0.000000000000000000, 0.000000000000000000 ) ) ;
#21096=EDGE_CURVE ( 'NONE', #7582, #14460, #387, .T. ) ;
#21098=CARTESIAN_POINT ( 'NONE',  ( 29.09636799667075024, -10.98232076577232519, 1.000000000000000000 ) ) ;
#21102=DIRECTION ( 'NONE',  ( 1.000000000000000000, 0.000000000000000000, 0.000000000000000000 ) ) ;
#21108=ORIENTED_EDGE ( 'NONE', *, *, #6740, .T. ) ;
#21109=ORIENTED_EDGE ( 'NONE', *, *, #11951, .T. ) ;
#21112=CARTESIAN_POINT ( 'NONE',  ( -29.41953157733101065, -10.08469938919468945, 1.000000000000000000 ) ) ;
#21115=ORIENTED_EDGE ( 'NONE', *, *, #22155, .T. ) ;
#21117=DIRECTION ( 'NONE',  ( 0.000000000000000000, 0.000000000000000000, 1.000000000000000000 ) ) ;
#21118=EDGE_CURVE ( 'NONE', #7323, #24696, #12070, .T. ) ;
#21124=EDGE_CURVE ( 'NONE', #4507, #2220, #2306, .T. ) ;
#21126=CARTESIAN_POINT ( 'NONE',  ( 0.000000000000000000, 0.000000000000000000, -6.500000000000000000 ) ) ;
#21128=EDGE_CURVE ( 'NONE', #3228, #21953, #23756, .T. ) ;
#21134=CARTESIAN_POINT ( 'NONE',  ( -28.91604871112448549, 11.44867358849382910, 1.000000000000000000 ) ) ;
#21135=CARTESIAN_POINT ( 'NONE',  ( 0.000000000000000000, 0.000000000000000000, -6.500000000000000000 ) ) ;
#21145=DIRECTION ( 'NONE',  ( 0.000000000000000000, 0.000000000000000000, 1.000000000000000000 ) ) ;
#21146=ORIENTED_EDGE ( 'NONE', *, *, #10271, .T. ) ;
#21156=ORIENTED_EDGE ( 'NONE', *, *, #6419, .F. ) ;
#21161=EDGE_CURVE ( 'NONE', #16896, #11078, #16299, .T. ) ;
#21165=EDGE_CURVE ( 'NONE', #18175, #2848, #21669, .T. ) ;
#21167=CARTESIAN_POINT ( 'NONE',  ( -28.91604871112448549, 11.44867358849382910, -6.500000000000000000 ) ) ;
#21170=CARTESIAN_POINT ( 'NONE',  ( 27.10000000000000142, 3.318792825689327485E-15, 0.000000000000000000 ) ) ;
#21171=CARTESIAN_POINT ( 'NONE',  ( 5.827558883615830965, -30.54913349766226105, -6.500000000000000000 ) ) ;
#21178=VERTEX_POINT ( 'NONE', #1237 ) ;
#21180=DIRECTION ( 'NONE',  ( 1.000000000000000000, 0.000000000000000000, 0.000000000000000000 ) ) ;
#21181=DIRECTION ( 'NONE',  ( 0.000000000000000000, 0.000000000000000000, 1.000000000000000000 ) ) ;
#21187=DIRECTION ( 'NONE',  ( 0.000000000000000000, 0.000000000000000000, 1.000000000000000000 ) ) ;
#21188=CARTESIAN_POINT ( 'NONE',  ( 0.000000000000000000, 0.000000000000000000, 1.000000000000000000 ) ) ;
#21190=ADVANCED_FACE ( 'NONE', ( #25304 ), #21383, .T. ) ;
#21193=DIRECTION ( 'NONE',  ( 0.000000000000000000, -0.000000000000000000, -1.000000000000000000 ) ) ;
#21199=CARTESIAN_POINT ( 'NONE',  ( 0.000000000000000000, 0.000000000000000000, -6.500000000000000000 ) ) ;
#21200=CARTESIAN_POINT ( 'NONE',  ( 30.63887302793247969, 5.335677986744675749, -6.500000000000000000 ) ) ;
#21201=DIRECTION ( 'NONE',  ( -0.000000000000000000, -0.000000000000000000, 1.000000000000000000 ) ) ;
#21205=VECTOR ( 'NONE', #19334, 1000.000000000000000 ) ;
#21209=ORIENTED_EDGE ( 'NONE', *, *, #15739, .T. ) ;
#21210=ORIENTED_EDGE ( 'NONE', *, *, #12919, .F. ) ;
#21214=ORIENTED_EDGE ( 'NONE', *, *, #17830, .F. ) ;
#21215=DIRECTION ( 'NONE',  ( 0.000000000000000000, 0.000000000000000000, 1.000000000000000000 ) ) ;
#21216=ORIENTED_EDGE ( 'NONE', *, *, #23587, .T. ) ;
#21219=DIRECTION ( 'NONE',  ( 1.000000000000000000, 0.000000000000000000, 0.000000000000000000 ) ) ;
#21222=ADVANCED_FACE ( 'NONE', ( #7130 ), #2947, .F. ) ;
#21223=LINE ( 'NONE', #20984, #21324 ) ;
#21226=EDGE_CURVE ( 'NONE', #1345, #962, #22080, .T. ) ;
#21230=ORIENTED_EDGE ( 'NONE', *, *, #15482, .T. ) ;
#21232=DIRECTION ( 'NONE',  ( -0.000000000000000000, -0.000000000000000000, 1.000000000000000000 ) ) ;
#21233=EDGE_CURVE ( 'NONE', #5166, #23155, #1109, .T. ) ;
#21234=CIRCLE ( 'NONE', #10354, 31.10000000000000142 ) ;
#21235=EDGE_LOOP ( 'NONE', ( #15461, #10170, #250, #3362 ) ) ;
#21237=CIRCLE ( 'NONE', #7460, 31.10000000000000142 ) ;
#21239=CARTESIAN_POINT ( 'NONE',  ( -13.69242354489172797, -27.92360179968362743, -6.500000000000000000 ) ) ;
#21243=AXIS2_PLACEMENT_3D ( 'NONE', #17553, #25528, #25390 ) ;
#21245=AXIS2_PLACEMENT_3D ( 'NONE', #1043, #15033, #9016 ) ;
#21248=DIRECTION ( 'NONE',  ( -0.000000000000000000, 0.000000000000000000, 1.000000000000000000 ) ) ;
#21252=VECTOR ( 'NONE', #6765, 1000.000000000000000 ) ;
#21257=DIRECTION ( 'NONE',  ( -0.8443279255020122998, 0.5358267949790012086, 0.000000000000000000 ) ) ;
#21258=AXIS2_PLACEMENT_3D ( 'NONE', #21902, #8293, #6073 ) ;
#21259=FACE_OUTER_BOUND ( 'NONE', #15265, .T. ) ;
#21260=EDGE_CURVE ( 'NONE', #13647, #6542, #14156, .T. ) ;
#21267=CARTESIAN_POINT ( 'NONE',  ( 0.000000000000000000, 0.000000000000000000, -6.500000000000000000 ) ) ;
#21269=CARTESIAN_POINT ( 'NONE',  ( -17.87326343783906424, 25.45105997952945387, -6.500000000000000000 ) ) ;
#21270=EDGE_LOOP ( 'NONE', ( #13273, #16228, #15845, #22247 ) ) ;
#21276=VECTOR ( 'NONE', #6369, 1000.000000000000000 ) ;
#21277=CIRCLE ( 'NONE', #24208, 0.5000000000000001110 ) ;
#21282=DIRECTION ( 'NONE',  ( -0.9822872507286872779, 0.1873813145857327056, 0.000000000000000000 ) ) ;
#21284=AXIS2_PLACEMENT_3D ( 'NONE', #13639, #9718, #5274 ) ;
#21288=VECTOR ( 'NONE', #23429, 1000.000000000000000 ) ;
#21289=CARTESIAN_POINT ( 'NONE',  ( 0.000000000000000000, 0.000000000000000000, 1.000000000000000000 ) ) ;
#21291=EDGE_CURVE ( 'NONE', #23177, #2690, #24916, .T. ) ;
#21295=DIRECTION ( 'NONE',  ( 0.000000000000000000, 0.000000000000000000, 1.000000000000000000 ) ) ;
#21297=LINE ( 'NONE', #3377, #21205 ) ;
#21299=CYLINDRICAL_SURFACE ( 'NONE', #23738, 0.5000000000000004441 ) ;
#21301=CARTESIAN_POINT ( 'NONE',  ( -1.452785157361201396, 31.03863125411927371, 1.000000000000000000 ) ) ;
#21304=CIRCLE ( 'NONE', #6256, 0.4999999999999998890 ) ;
#21305=DIRECTION ( 'NONE',  ( 0.000000000000000000, 0.000000000000000000, 1.000000000000000000 ) ) ;
#21306=EDGE_CURVE ( 'NONE', #14582, #13859, #5800, .T. ) ;
#21307=DIRECTION ( 'NONE',  ( 0.000000000000000000, 0.000000000000000000, 1.000000000000000000 ) ) ;
#21308=CARTESIAN_POINT ( 'NONE',  ( -30.45149776762733751, -6.317933499823126908, -2.750000000000000000 ) ) ;
#21311=DIRECTION ( 'NONE',  ( 0.000000000000000000, 0.000000000000000000, 1.000000000000000000 ) ) ;
#21313=ORIENTED_EDGE ( 'NONE', *, *, #16545, .T. ) ;
#21314=ADVANCED_FACE ( 'NONE', ( #6993 ), #3196, .T. ) ;
#21316=VECTOR ( 'NONE', #18043, 1000.000000000000000 ) ;
#21317=ORIENTED_EDGE ( 'NONE', *, *, #2204, .F. ) ;
#21321=CARTESIAN_POINT ( 'NONE',  ( 0.000000000000000000, 0.000000000000000000, -6.500000000000000000 ) ) ;
#21322=VECTOR ( 'NONE', #4048, 1000.000000000000000 ) ;
#21324=VECTOR ( 'NONE', #3306, 1000.000000000000000 ) ;
#21326=CIRCLE ( 'NONE', #7953, 31.10000000000000142 ) ;
#21330=LINE ( 'NONE', #23283, #5860 ) ;
#21331=CIRCLE ( 'NONE', #10047, 31.10000000000000142 ) ;
#21333=DIRECTION ( 'NONE',  ( 1.000000000000000000, 0.000000000000000000, 0.000000000000000000 ) ) ;
#21339=LINE ( 'NONE', #3421, #21625 ) ;
#21343=CARTESIAN_POINT ( 'NONE',  ( -16.23990935651735867, -26.52310962334733446, 1.000000000000000000 ) ) ;
#21344=AXIS2_PLACEMENT_3D ( 'NONE', #12882, #23093, #16827 ) ;
#21345=ORIENTED_EDGE ( 'NONE', *, *, #12482, .T. ) ;
#21346=VECTOR ( 'NONE', #21546, 1000.000000000000000 ) ;
#21348=DIRECTION ( 'NONE',  ( -0.9297764858882532346, -0.3681245526846732008, 0.000000000000000000 ) ) ;
#21352=VERTEX_POINT ( 'NONE', #18908 ) ;
#21353=DIRECTION ( 'NONE',  ( -0.000000000000000000, -0.000000000000000000, 1.000000000000000000 ) ) ;
#21358=EDGE_CURVE ( 'NONE', #22500, #1051, #25850, .T. ) ;
#21359=DIRECTION ( 'NONE',  ( 1.000000000000000000, 0.000000000000000000, 0.000000000000000000 ) ) ;
#21361=VECTOR ( 'NONE', #23762, 1000.000000000000000 ) ;
#21363=DIRECTION ( 'NONE',  ( 0.000000000000000000, -0.000000000000000000, 1.000000000000000000 ) ) ;
#21366=CIRCLE ( 'NONE', #8838, 0.5000000000000011102 ) ;
#21367=DIRECTION ( 'NONE',  ( 0.1253332335643120576, 0.9921147013144768767, 0.000000000000000000 ) ) ;
#21368=EDGE_CURVE ( 'NONE', #18639, #2848, #3300, .T. ) ;
#21371=CYLINDRICAL_SURFACE ( 'NONE', #2054, 0.4999999999999970024 ) ;
#21372=AXIS2_PLACEMENT_3D ( 'NONE', #25715, #15534, #13568 ) ;
#21374=ORIENTED_EDGE ( 'NONE', *, *, #7539, .F. ) ;
#21377=ORIENTED_EDGE ( 'NONE', *, *, #4312, .T. ) ;
#21380=CARTESIAN_POINT ( 'NONE',  ( 0.000000000000000000, 0.000000000000000000, 1.000000000000000000 ) ) ;
#21381=VERTEX_POINT ( 'NONE', #6334 ) ;
#21382=ORIENTED_EDGE ( 'NONE', *, *, #2903, .F. ) ;
#21383=CYLINDRICAL_SURFACE ( 'NONE', #6206, 31.10000000000000142 ) ;
#21386=LINE ( 'NONE', #13272, #20243 ) ;
#21387=EDGE_LOOP ( 'NONE', ( #15949, #23537, #11435, #9152 ) ) ;
#21391=AXIS2_PLACEMENT_3D ( 'NONE', #937, #4852, #6547 ) ;
#21395=ADVANCED_FACE ( 'NONE', ( #2021 ), #23863, .F. ) ;
#21397=CIRCLE ( 'NONE', #5113, 0.5000000000000006661 ) ;
#21398=CARTESIAN_POINT ( 'NONE',  ( -30.85476721088022600, 3.897863563850190616, -6.500000000000000000 ) ) ;
#21403=CARTESIAN_POINT ( 'NONE',  ( -31.00322564728510955, 2.451530025009474034, -2.750000000000000000 ) ) ;
#21408=ORIENTED_EDGE ( 'NONE', *, *, #9923, .T. ) ;
#21419=ORIENTED_EDGE ( 'NONE', *, *, #12831, .F. ) ;
#21422=EDGE_CURVE ( 'NONE', #18350, #7360, #4162, .T. ) ;
#21423=CARTESIAN_POINT ( 'NONE',  ( -31.00322564728510955, 2.451530025009473590, -6.500000000000000000 ) ) ;
#21427=VECTOR ( 'NONE', #24970, 1000.000000000000000 ) ;
#21438=CARTESIAN_POINT ( 'NONE',  ( -20.78941499438192508, 22.67092431280617859, 1.000000000000000000 ) ) ;
#21439=AXIS2_PLACEMENT_3D ( 'NONE', #5392, #1744, #5655 ) ;
#21442=ORIENTED_EDGE ( 'NONE', *, *, #7481, .F. ) ;
#21445=CARTESIAN_POINT ( 'NONE',  ( 29.57785765677924061, -9.610428525060996208, 1.000000000000000000 ) ) ;
#21446=ORIENTED_EDGE ( 'NONE', *, *, #15787, .F. ) ;
#21447=AXIS2_PLACEMENT_3D ( 'NONE', #138, #19859, #1957 ) ;
#21448=ORIENTED_EDGE ( 'NONE', *, *, #12543, .T. ) ;
#21449=EDGE_LOOP ( 'NONE', ( #20269, #3081, #25846, #4454 ) ) ;
#21451=ORIENTED_EDGE ( 'NONE', *, *, #25751, .T. ) ;
#21452=DIRECTION ( 'NONE',  ( 1.000000000000000000, 0.000000000000000000, 0.000000000000000000 ) ) ;
#21455=ADVANCED_FACE ( 'NONE', ( #5948 ), #20187, .T. ) ;
#21456=DIRECTION ( 'NONE',  ( 0.9510565162951586382, 0.3090169943749320192, 0.000000000000000000 ) ) ;
#21458=ADVANCED_FACE ( 'NONE', ( #321 ), #2287, .T. ) ;
#21463=AXIS2_PLACEMENT_3D ( 'NONE', #14596, #16449, #22440 ) ;
#21464=CARTESIAN_POINT ( 'NONE',  ( -30.04913349766228592, -5.827558883615738594, -6.500000000000000000 ) ) ;
#21468=DIRECTION ( 'NONE',  ( 0.000000000000000000, 0.000000000000000000, -1.000000000000000000 ) ) ;
#21472=CARTESIAN_POINT ( 'NONE',  ( 0.000000000000000000, 0.000000000000000000, -6.500000000000000000 ) ) ;
#21473=DIRECTION ( 'NONE',  ( 1.000000000000000000, 0.000000000000000000, 0.000000000000000000 ) ) ;
#21475=DIRECTION ( 'NONE',  ( 1.000000000000000000, 0.000000000000000000, 0.000000000000000000 ) ) ;
#21477=CYLINDRICAL_SURFACE ( 'NONE', #12096, 31.10000000000000142 ) ;
#21479=ORIENTED_EDGE ( 'NONE', *, *, #4897, .T. ) ;
#21480=CYLINDRICAL_SURFACE ( 'NONE', #21645, 31.10000000000000142 ) ;
#21486=ORIENTED_EDGE ( 'NONE', *, *, #18524, .F. ) ;
#21491=CARTESIAN_POINT ( 'NONE',  ( -3.897863563849436552, 30.85476721088031482, -6.500000000000000000 ) ) ;
#21496=EDGE_CURVE ( 'NONE', #3018, #14914, #8432, .T. ) ;
#21498=ORIENTED_EDGE ( 'NONE', *, *, #8109, .T. ) ;
#21505=VERTEX_POINT ( 'NONE', #12467 ) ;
#21506=ORIENTED_EDGE ( 'NONE', *, *, #23952, .T. ) ;
#21508=ORIENTED_EDGE ( 'NONE', *, *, #17270, .T. ) ;
#21509=FACE_OUTER_BOUND ( 'NONE', #2495, .T. ) ;
#21514=CARTESIAN_POINT ( 'NONE',  ( -12.74173596767398742, -28.14012133169310559, -6.500000000000000000 ) ) ;
#21515=EDGE_CURVE ( 'NONE', #13703, #14349, #22933, .T. ) ;
#21522=LINE ( 'NONE', #13289, #472 ) ;
#21526=CARTESIAN_POINT ( 'NONE',  ( 24.86329371854761305, -18.68225429291740269, -2.750000000000000000 ) ) ;
#21528=CARTESIAN_POINT ( 'NONE',  ( -3.897863563850083146, -30.85476721088024021, -6.500000000000000000 ) ) ;
#21530=DIRECTION ( 'NONE',  ( 0.000000000000000000, 0.000000000000000000, 1.000000000000000000 ) ) ;
#21531=EDGE_LOOP ( 'NONE', ( #3494, #1099, #11849, #4258 ) ) ;
#21536=CIRCLE ( 'NONE', #10245, 31.10000000000000142 ) ;
#21538=ORIENTED_EDGE ( 'NONE', *, *, #23843, .F. ) ;
#21543=( NAMED_UNIT ( * ) SI_UNIT ( $, .STERADIAN. ) SOLID_ANGLE_UNIT ( ) );
#21546=DIRECTION ( 'NONE',  ( 0.000000000000000000, 0.000000000000000000, -1.000000000000000000 ) ) ;
#21547=FACE_OUTER_BOUND ( 'NONE', #9417, .T. ) ;
#21553=ORIENTED_EDGE ( 'NONE', *, *, #11089, .F. ) ;
#21557=ADVANCED_FACE ( 'NONE', ( #24628 ), #22686, .T. ) ;
#21560=ORIENTED_EDGE ( 'NONE', *, *, #13785, .T. ) ;
#21561=CARTESIAN_POINT ( 'NONE',  ( 0.000000000000000000, 0.000000000000000000, -6.500000000000000000 ) ) ;
#21562=CARTESIAN_POINT ( 'NONE',  ( -6.317933499823532806, -30.45149776762725580, 1.000000000000000000 ) ) ;
#21563=CARTESIAN_POINT ( 'NONE',  ( 28.72825533807133169, 11.91206721063041485, -6.500000000000000000 ) ) ;
#21567=VERTEX_POINT ( 'NONE', #2792 ) ;
#21570=LINE ( 'NONE', #3649, #9300 ) ;
#21572=CARTESIAN_POINT ( 'NONE',  ( 12.78762572734057024, 28.34936733434201273, -2.750000000000000000 ) ) ;
#21576=LINE ( 'NONE', #5500, #17694 ) ;
#21578=CARTESIAN_POINT ( 'NONE',  ( 0.000000000000000000, 0.000000000000000000, -6.500000000000000000 ) ) ;
#21579=CYLINDRICAL_SURFACE ( 'NONE', #9686, 0.5000000000000004441 ) ;
#21582=DIRECTION ( 'NONE',  ( 1.000000000000000000, 0.000000000000000000, 0.000000000000000000 ) ) ;
#21586=CIRCLE ( 'NONE', #20321, 31.10000000000000142 ) ;
#21587=CYLINDRICAL_SURFACE ( 'NONE', #19951, 31.10000000000000142 ) ;
#21590=LINE ( 'NONE', #17684, #19745 ) ;
#21593=VERTEX_POINT ( 'NONE', #11029 ) ;
#21596=DIRECTION ( 'NONE',  ( 0.3090169943749456194, -0.9510565162951541973, 0.000000000000000000 ) ) ;
#21597=VERTEX_POINT ( 'NONE', #8956 ) ;
#21606=CARTESIAN_POINT ( 'NONE',  ( 21.65113613650327196, -22.32573188046928436, 1.000000000000000000 ) ) ;
#21610=EDGE_CURVE ( 'NONE', #7673, #1524, #25021, .T. ) ;
#21613=LINE ( 'NONE', #13773, #497 ) ;
#21615=ORIENTED_EDGE ( 'NONE', *, *, #10760, .F. ) ;
#21617=ORIENTED_EDGE ( 'NONE', *, *, #1508, .F. ) ;
#21623=EDGE_CURVE ( 'NONE', #19911, #25487, #13133, .T. ) ;
#21625=VECTOR ( 'NONE', #5895, 1000.000000000000000 ) ;
#21628=EDGE_CURVE ( 'NONE', #18048, #161, #13356, .T. ) ;
#21629=CARTESIAN_POINT ( 'NONE',  ( -19.82388608118446527, -23.96296185032687376, -6.500000000000000000 ) ) ;
#21630=DIRECTION ( 'NONE',  ( -0.000000000000000000, -0.000000000000000000, 1.000000000000000000 ) ) ;
#21633=AXIS2_PLACEMENT_3D ( 'NONE', #2477, #20659, #6407 ) ;
#21637=CYLINDRICAL_SURFACE ( 'NONE', #15464, 0.5000000000000004441 ) ;
#21645=AXIS2_PLACEMENT_3D ( 'NONE', #19881, #5904, #5521 ) ;
#21649=VECTOR ( 'NONE', #3632, 1000.000000000000000 ) ;
#21650=ORIENTED_EDGE ( 'NONE', *, *, #22050, .T. ) ;
#21654=ORIENTED_EDGE ( 'NONE', *, *, #13200, .T. ) ;
#21656=CARTESIAN_POINT ( 'NONE',  ( 3.897863563849872204, 30.85476721088026508, 1.000000000000000000 ) ) ;
#21658=DIRECTION ( 'NONE',  ( 1.000000000000000000, 0.000000000000000000, 0.000000000000000000 ) ) ;
#21660=VERTEX_POINT ( 'NONE', #23448 ) ;
#21661=ADVANCED_FACE ( 'NONE', ( #23695 ), #5776, .F. ) ;
#21664=EDGE_CURVE ( 'NONE', #2083, #18610, #16693, .T. ) ;
#21669=CIRCLE ( 'NONE', #25018, 0.4999999999999986122 ) ;
#21670=AXIS2_PLACEMENT_3D ( 'NONE', #12948, #14518, #12417 ) ;
#21671=CARTESIAN_POINT ( 'NONE',  ( 3.401318489841097747, 30.91344420362547396, -6.500000000000000000 ) ) ;
#21672=DIRECTION ( 'NONE',  ( -0.000000000000000000, 0.000000000000000000, 1.000000000000000000 ) ) ;
#21673=CARTESIAN_POINT ( 'NONE',  ( 10.98232076577222038, 29.09636799667079288, 1.000000000000000000 ) ) ;
#21675=DIRECTION ( 'NONE',  ( 0.000000000000000000, 0.000000000000000000, 1.000000000000000000 ) ) ;
#21680=CARTESIAN_POINT ( 'NONE',  ( -9.610428525061097460, -29.57785765677920509, -6.500000000000000000 ) ) ;
#21684=VECTOR ( 'NONE', #9148, 1000.000000000000000 ) ;
#21687=ORIENTED_EDGE ( 'NONE', *, *, #24522, .T. ) ;
#21688=LINE ( 'NONE', #9793, #13853 ) ;
#21691=VERTEX_POINT ( 'NONE', #17565 ) ;
#21692=AXIS2_PLACEMENT_3D ( 'NONE', #14420, #4072, #4207 ) ;
#21694=CIRCLE ( 'NONE', #405, 0.5000000000000006661 ) ;
#21695=ORIENTED_EDGE ( 'NONE', *, *, #17500, .T. ) ;
#21697=ORIENTED_EDGE ( 'NONE', *, *, #19307, .T. ) ;
#21701=CIRCLE ( 'NONE', #9582, 0.4999999999999992784 ) ;
#21703=DIRECTION ( 'NONE',  ( 1.000000000000000000, 0.000000000000000000, 0.000000000000000000 ) ) ;
#21704=AXIS2_PLACEMENT_3D ( 'NONE', #3207, #3475, #5569 ) ;
#21705=AXIS2_PLACEMENT_3D ( 'NONE', #17100, #15008, #17243 ) ;
#21709=EDGE_CURVE ( 'NONE', #5387, #414, #23311, .T. ) ;
#21710=CARTESIAN_POINT ( 'NONE',  ( 0.000000000000000000, 0.000000000000000000, -6.500000000000000000 ) ) ;
#21711=DIRECTION ( 'NONE',  ( 0.5877852522924853496, 0.8090169943749385695, 0.000000000000000000 ) ) ;
#21712=VECTOR ( 'NONE', #7857, 1000.000000000000000 ) ;
#21716=CARTESIAN_POINT ( 'NONE',  ( -1.452785157361865531, -31.03863125411923463, -6.500000000000000000 ) ) ;
#21719=CARTESIAN_POINT ( 'NONE',  ( 30.54913349766219710, -5.827558883616158703, 1.000000000000000000 ) ) ;
#21720=AXIS2_PLACEMENT_3D ( 'NONE', #9669, #19589, #15807 ) ;
#21725=ORIENTED_EDGE ( 'NONE', *, *, #11499, .T. ) ;
#21729=LINE ( 'NONE', #3813, #9964 ) ;
#21732=VERTEX_POINT ( 'NONE', #11540 ) ;
#21739=EDGE_CURVE ( 'NONE', #16708, #14667, #15444, .T. ) ;
#21740=CARTESIAN_POINT ( 'NONE',  ( -30.85476721088022600, 3.897863563850190616, 1.000000000000000000 ) ) ;
#21741=DIRECTION ( 'NONE',  ( 0.4817536741017267032, 0.8763066800438573667, 0.000000000000000000 ) ) ;
#21743=AXIS2_PLACEMENT_3D ( 'NONE', #15032, #24844, #13076 ) ;
#21745=AXIS2_PLACEMENT_3D ( 'NONE', #19781, #1878, #9840 ) ;
#21750=VECTOR ( 'NONE', #2472, 1000.000000000000000 ) ;
#21754=VERTEX_POINT ( 'NONE', #1483 ) ;
#21755=ORIENTED_EDGE ( 'NONE', *, *, #24415, .F. ) ;
#21758=EDGE_LOOP ( 'NONE', ( #20305, #1495, #10458, #6502 ) ) ;
#21761=CARTESIAN_POINT ( 'NONE',  ( 0.000000000000000000, 0.000000000000000000, -6.500000000000000000 ) ) ;
#21763=ORIENTED_EDGE ( 'NONE', *, *, #16940, .T. ) ;
#21764=AXIS2_PLACEMENT_3D ( 'NONE', #6616, #18542, #22446 ) ;
#21765=FACE_OUTER_BOUND ( 'NONE', #22074, .T. ) ;
#21766=ORIENTED_EDGE ( 'NONE', *, *, #12325, .F. ) ;
#21770=AXIS2_PLACEMENT_3D ( 'NONE', #12900, #8591, #20747 ) ;
#21771=FACE_OUTER_BOUND ( 'NONE', #1311, .T. ) ;
#21773=EDGE_CURVE ( 'NONE', #7744, #15159, #15855, .T. ) ;
#21775=EDGE_CURVE ( 'NONE', #246, #161, #4135, .T. ) ;
#21777=AXIS2_PLACEMENT_3D ( 'NONE', #4251, #327, #22167 ) ;
#21778=AXIS2_PLACEMENT_3D ( 'NONE', #6440, #8406, #14814 ) ;
#21780=CARTESIAN_POINT ( 'NONE',  ( 0.000000000000000000, 0.000000000000000000, 1.000000000000000000 ) ) ;
#21784=EDGE_CURVE ( 'NONE', #17935, #20933, #11146, .T. ) ;
#21795=VERTEX_POINT ( 'NONE', #15222 ) ;
#21797=AXIS2_PLACEMENT_3D ( 'NONE', #21656, #23501, #11969 ) ;
#21798=FACE_OUTER_BOUND ( 'NONE', #22135, .T. ) ;
#21799=VERTEX_POINT ( 'NONE', #1361 ) ;
#21800=DIRECTION ( 'NONE',  ( -0.000000000000000000, 0.000000000000000000, 1.000000000000000000 ) ) ;
#21801=ORIENTED_EDGE ( 'NONE', *, *, #20668, .F. ) ;
#21803=CARTESIAN_POINT ( 'NONE',  ( -10.98232076577242644, -29.09636799667071116, -2.750000000000000000 ) ) ;
#21805=AXIS2_PLACEMENT_3D ( 'NONE', #17541, #151, #17921 ) ;
#21807=VECTOR ( 'NONE', #21630, 1000.000000000000000 ) ;
#21812=AXIS2_PLACEMENT_3D ( 'NONE', #675, #10852, #22372 ) ;
#21814=CARTESIAN_POINT ( 'NONE',  ( -24.86329371854747805, 18.68225429291759099, -6.500000000000000000 ) ) ;
#21817=DIRECTION ( 'NONE',  ( 1.000000000000000000, 0.000000000000000000, 0.000000000000000000 ) ) ;
#21819=ORIENTED_EDGE ( 'NONE', *, *, #19234, .T. ) ;
#21825=CYLINDRICAL_SURFACE ( 'NONE', #14969, 0.5000000000000004441 ) ;
#21827=DIRECTION ( 'NONE',  ( 0.000000000000000000, 0.000000000000000000, 1.000000000000000000 ) ) ;
#21828=ORIENTED_EDGE ( 'NONE', *, *, #19003, .F. ) ;
#21833=ORIENTED_EDGE ( 'NONE', *, *, #25853, .F. ) ;
#21835=ORIENTED_EDGE ( 'NONE', *, *, #8635, .T. ) ;
#21840=VECTOR ( 'NONE', #7194, 1000.000000000000000 ) ;
#21846=CIRCLE ( 'NONE', #25193, 31.10000000000000142 ) ;
#21851=CARTESIAN_POINT ( 'NONE',  ( 0.000000000000000000, 0.000000000000000000, -6.500000000000000000 ) ) ;
#21854=EDGE_CURVE ( 'NONE', #24465, #5387, #1639, .T. ) ;
#21855=FACE_OUTER_BOUND ( 'NONE', #4820, .T. ) ;
#21857=DIRECTION ( 'NONE',  ( 0.000000000000000000, 0.000000000000000000, 1.000000000000000000 ) ) ;
#21863=ORIENTED_EDGE ( 'NONE', *, *, #21291, .F. ) ;
#21864=FACE_OUTER_BOUND ( 'NONE', #12030, .T. ) ;
#21865=VERTEX_POINT ( 'NONE', #22121 ) ;
#21869=EDGE_CURVE ( 'NONE', #18350, #8164, #22945, .T. ) ;
#21873=AXIS2_PLACEMENT_3D ( 'NONE', #8111, #17908, #3534 ) ;
#21875=DIRECTION ( 'NONE',  ( 0.000000000000000000, 0.000000000000000000, -1.000000000000000000 ) ) ;
#21882=FACE_OUTER_BOUND ( 'NONE', #510, .T. ) ;
#21889=DIRECTION ( 'NONE',  ( 0.000000000000000000, 0.000000000000000000, -1.000000000000000000 ) ) ;
#21894=EDGE_CURVE ( 'NONE', #6294, #7204, #3718, .T. ) ;
#21896=EDGE_LOOP ( 'NONE', ( #3837, #16649, #443, #20204 ) ) ;
#21900=VECTOR ( 'NONE', #21889, 1000.000000000000000 ) ;
#21902=CARTESIAN_POINT ( 'NONE',  ( 0.000000000000000000, 0.000000000000000000, -6.500000000000000000 ) ) ;
#21905=DIRECTION ( 'NONE',  ( 0.000000000000000000, 0.000000000000000000, 1.000000000000000000 ) ) ;
#21906=CIRCLE ( 'NONE', #7303, 31.10000000000000142 ) ;
#21912=CYLINDRICAL_SURFACE ( 'NONE', #13733, 0.5000000000000004441 ) ;
#21913=EDGE_CURVE ( 'NONE', #24200, #2002, #19184, .T. ) ;
#21919=ORIENTED_EDGE ( 'NONE', *, *, #4132, .T. ) ;
#21921=EDGE_CURVE ( 'NONE', #1666, #20500, #16120, .T. ) ;
#21922=DIRECTION ( 'NONE',  ( 0.7705132427757873659, -0.6374239897486919659, 0.000000000000000000 ) ) ;
#21923=CARTESIAN_POINT ( 'NONE',  ( 0.4999838450259764255, 31.09598070739550124, -6.500000000000000000 ) ) ;
#21926=VERTEX_POINT ( 'NONE', #25785 ) ;
#21927=EDGE_CURVE ( 'NONE', #9386, #13117, #13759, .T. ) ;
#21931=EDGE_CURVE ( 'NONE', #2220, #5530, #23780, .T. ) ;
#21938=LINE ( 'NONE', #2201, #18330 ) ;
#21942=ORIENTED_EDGE ( 'NONE', *, *, #21931, .F. ) ;
#21948=CARTESIAN_POINT ( 'NONE',  ( -29.99470236596021167, 8.217531866531519569, -6.500000000000000000 ) ) ;
#21949=EDGE_LOOP ( 'NONE', ( #10899, #23238, #21064, #16923 ) ) ;
#21950=DIRECTION ( 'NONE',  ( 1.000000000000000000, 0.000000000000000000, 0.000000000000000000 ) ) ;
#21953=VERTEX_POINT ( 'NONE', #20159 ) ;
#21954=VERTEX_POINT ( 'NONE', #18213 ) ;
#21955=VERTEX_POINT ( 'NONE', #14295 ) ;
#21959=DIRECTION ( 'NONE',  ( 0.000000000000000000, 0.000000000000000000, 1.000000000000000000 ) ) ;
#21965=CIRCLE ( 'NONE', #3576, 0.5000000000000003331 ) ;
#21969=DIRECTION ( 'NONE',  ( 0.000000000000000000, 0.000000000000000000, 1.000000000000000000 ) ) ;
#21971=CARTESIAN_POINT ( 'NONE',  ( -25.16042852506064165, 18.28012134629622309, 1.000000000000000000 ) ) ;
#21973=APPLICATION_CONTEXT ( 'automotive_design' ) ;
#21975=DIRECTION ( 'NONE',  ( 0.000000000000000000, 0.000000000000000000, 1.000000000000000000 ) ) ;
#21981=EDGE_LOOP ( 'NONE', ( #519, #24342, #164, #24044 ) ) ;
#21983=DIRECTION ( 'NONE',  ( 0.000000000000000000, 0.000000000000000000, 1.000000000000000000 ) ) ;
#21984=ORIENTED_EDGE ( 'NONE', *, *, #17042, .T. ) ;
#21988=ORIENTED_EDGE ( 'NONE', *, *, #19522, .F. ) ;
#21989=ORIENTED_EDGE ( 'NONE', *, *, #21921, .F. ) ;
#21991=ORIENTED_EDGE ( 'NONE', *, *, #8746, .T. ) ;
#21992=DIRECTION ( 'NONE',  ( 0.000000000000000000, 0.000000000000000000, 1.000000000000000000 ) ) ;
#21994=EDGE_CURVE ( 'NONE', #19514, #18149, #17131, .T. ) ;
#21996=DIRECTION ( 'NONE',  ( 1.000000000000000000, 0.000000000000000000, 0.000000000000000000 ) ) ;
#22000=CARTESIAN_POINT ( 'NONE',  ( -30.35476721088022600, 3.897863563850190616, 1.000000000000000000 ) ) ;
#22005=CARTESIAN_POINT ( 'NONE',  ( -22.67092431280609688, -21.28941499438201745, 1.000000000000000000 ) ) ;
#22006=ORIENTED_EDGE ( 'NONE', *, *, #21515, .F. ) ;
#22007=ORIENTED_EDGE ( 'NONE', *, *, #13804, .T. ) ;
#22012=CARTESIAN_POINT ( 'NONE',  ( 0.000000000000000000, 0.000000000000000000, -6.500000000000000000 ) ) ;
#22014=ORIENTED_EDGE ( 'NONE', *, *, #10821, .F. ) ;
#22016=VERTEX_POINT ( 'NONE', #22780 ) ;
#22020=CARTESIAN_POINT ( 'NONE',  ( -2.451530025009351910, -31.00322564728512020, -6.500000000000000000 ) ) ;
#22021=EDGE_CURVE ( 'NONE', #2564, #24580, #16718, .T. ) ;
#22027=DIRECTION ( 'NONE',  ( 0.000000000000000000, 0.000000000000000000, 1.000000000000000000 ) ) ;
#22028=DIRECTION ( 'NONE',  ( 0.000000000000000000, 0.000000000000000000, 1.000000000000000000 ) ) ;
#22031=DIRECTION ( 'NONE',  ( 0.4257792915650852050, 0.9048270524660135816, 0.000000000000000000 ) ) ;
#22033=AXIS2_PLACEMENT_3D ( 'NONE', #18897, #19266, #1369 ) ;
#22035=ORIENTED_EDGE ( 'NONE', *, *, #24365, .F. ) ;
#22043=ORIENTED_EDGE ( 'NONE', *, *, #20508, .T. ) ;
#22044=ORIENTED_EDGE ( 'NONE', *, *, #23989, .F. ) ;
#22045=LINE ( 'NONE', #21803, #6371 ) ;
#22047=DIRECTION ( 'NONE',  ( 0.2486898871648653975, 0.9685831611286285225, 0.000000000000000000 ) ) ;
#22049=AXIS2_PLACEMENT_3D ( 'NONE', #11905, #19873, #7468 ) ;
#22050=EDGE_CURVE ( 'NONE', #7760, #22793, #24739, .T. ) ;
#22053=FACE_OUTER_BOUND ( 'NONE', #19978, .T. ) ;
#22056=AXIS2_PLACEMENT_3D ( 'NONE', #17161, #25262, #17414 ) ;
#22060=ORIENTED_EDGE ( 'NONE', *, *, #13506, .T. ) ;
#22067=VERTEX_POINT ( 'NONE', #10473 ) ;
#22068=FACE_OUTER_BOUND ( 'NONE', #23494, .T. ) ;
#22070=CYLINDRICAL_SURFACE ( 'NONE', #6263, 31.10000000000000142 ) ;
#22073=AXIS2_PLACEMENT_3D ( 'NONE', #20105, #4535, #14099 ) ;
#22074=EDGE_LOOP ( 'NONE', ( #10950, #15242, #16043, #10256 ) ) ;
#22076=AXIS2_PLACEMENT_3D ( 'NONE', #3989, #9997, #17991 ) ;
#22078=DIRECTION ( 'NONE',  ( 0.9921147013144794302, 0.1253332335642911299, 0.000000000000000000 ) ) ;
#22080=CIRCLE ( 'NONE', #10792, 31.10000000000000142 ) ;
#22084=DIRECTION ( 'NONE',  ( 0.9822872507286911636, 0.1873813145857119722, 0.000000000000000000 ) ) ;
#22092=CARTESIAN_POINT ( 'NONE',  ( 30.85476721088025442, -3.897863563849982782, 1.000000000000000000 ) ) ;
#22093=CARTESIAN_POINT ( 'NONE',  ( 0.000000000000000000, 0.000000000000000000, -6.500000000000000000 ) ) ;
#22094=EDGE_CURVE ( 'NONE', #2636, #21178, #21304, .T. ) ;
#22098=CIRCLE ( 'NONE', #12479, 0.5000000000000002220 ) ;
#22100=DIRECTION ( 'NONE',  ( 0.000000000000000000, 0.000000000000000000, -1.000000000000000000 ) ) ;
#22102=EDGE_CURVE ( 'NONE', #19667, #10774, #6949, .T. ) ;
#22107=VECTOR ( 'NONE', #2681, 1000.000000000000000 ) ;
#22112=CIRCLE ( 'NONE', #7093, 0.5000000000000006661 ) ;
#22113=AXIS2_PLACEMENT_3D ( 'NONE', #12820, #3142, #17139 ) ;
#22114=ORIENTED_EDGE ( 'NONE', *, *, #25110, .F. ) ;
#22118=AXIS2_PLACEMENT_3D ( 'NONE', #2660, #20424, #18493 ) ;
#22121=CARTESIAN_POINT ( 'NONE',  ( -27.92360179968386547, -13.69242354489123770, 1.000000000000000000 ) ) ;
#22134=DIRECTION ( 'NONE',  ( 0.000000000000000000, 0.000000000000000000, 1.000000000000000000 ) ) ;
#22135=EDGE_LOOP ( 'NONE', ( #6298, #8315, #16503, #2310 ) ) ;
#22137=ORIENTED_EDGE ( 'NONE', *, *, #17800, .T. ) ;
#22141=ORIENTED_EDGE ( 'NONE', *, *, #12112, .F. ) ;
#22142=FACE_OUTER_BOUND ( 'NONE', #7712, .T. ) ;
#22145=ORIENTED_EDGE ( 'NONE', *, *, #2909, .T. ) ;
#22146=ADVANCED_FACE ( 'NONE', ( #3236 ), #3120, .T. ) ;
#22147=CYLINDRICAL_SURFACE ( 'NONE', #2738, 0.5000000000000000000 ) ;
#22148=AXIS2_PLACEMENT_3D ( 'NONE', #21761, #23850, #25559 ) ;
#22152=DIRECTION ( 'NONE',  ( 0.000000000000000000, 0.000000000000000000, 1.000000000000000000 ) ) ;
#22153=AXIS2_PLACEMENT_3D ( 'NONE', #8508, #16489, #10311 ) ;
#22154=VECTOR ( 'NONE', #5825, 1000.000000000000000 ) ;
#22155=EDGE_CURVE ( 'NONE', #3259, #12818, #19189, .T. ) ;
#22157=DIRECTION ( 'NONE',  ( -0.000000000000000000, -0.000000000000000000, 1.000000000000000000 ) ) ;
#22162=AXIS2_PLACEMENT_3D ( 'NONE', #7929, #13685, #21658 ) ;
#22163=EDGE_CURVE ( 'NONE', #11427, #13061, #10421, .T. ) ;
#22164=CARTESIAN_POINT ( 'NONE',  ( -30.45149776762720961, 6.317933499823766397, -6.500000000000000000 ) ) ;
#22165=PRODUCT_DEFINITION_SHAPE ( 'NONE', 'NONE',  #10273 ) ;
#22167=DIRECTION ( 'NONE',  ( 1.000000000000000000, 0.000000000000000000, 0.000000000000000000 ) ) ;
#22177=ORIENTED_EDGE ( 'NONE', *, *, #24202, .F. ) ;
#22178=VECTOR ( 'NONE', #13023, 1000.000000000000000 ) ;
#22180=AXIS2_PLACEMENT_3D ( 'NONE', #9396, #11598, #17378 ) ;
#22183=ORIENTED_EDGE ( 'NONE', *, *, #22021, .F. ) ;
#22191=CIRCLE ( 'NONE', #12161, 0.4999999999999997224 ) ;
#22201=VERTEX_POINT ( 'NONE', #21671 ) ;
#22203=CARTESIAN_POINT ( 'NONE',  ( -28.14012133169306296, 13.24173596767408867, -6.500000000000000000 ) ) ;
#22207=CIRCLE ( 'NONE', #13865, 31.10000000000000142 ) ;
#22208=DIRECTION ( 'NONE',  ( 0.000000000000000000, 0.000000000000000000, 1.000000000000000000 ) ) ;
#22210=ORIENTED_EDGE ( 'NONE', *, *, #12498, .F. ) ;
#22217=ORIENTED_EDGE ( 'NONE', *, *, #4434, .F. ) ;
#22219=VERTEX_POINT ( 'NONE', #13963 ) ;
#22220=CARTESIAN_POINT ( 'NONE',  ( 12.78762572734057024, 28.34936733434201273, -6.500000000000000000 ) ) ;
#22221=CIRCLE ( 'NONE', #7176, 31.10000000000000142 ) ;
#22224=AXIS2_PLACEMENT_3D ( 'NONE', #14413, #24588, #2497 ) ;
#22229=AXIS2_PLACEMENT_3D ( 'NONE', #22629, #20135, #14128 ) ;
#22230=DIRECTION ( 'NONE',  ( 0.000000000000000000, 0.000000000000000000, 1.000000000000000000 ) ) ;
#22231=CYLINDRICAL_SURFACE ( 'NONE', #23063, 31.10000000000000142 ) ;
#22233=DIRECTION ( 'NONE',  ( 1.000000000000000000, 0.000000000000000000, 0.000000000000000000 ) ) ;
#22234=CARTESIAN_POINT ( 'NONE',  ( 0.000000000000000000, -31.10000000000000142, -6.500000000000000000 ) ) ;
#22237=CARTESIAN_POINT ( 'NONE',  ( 10.08469938919477649, -29.41953157733097868, -6.500000000000000000 ) ) ;
#22243=CYLINDRICAL_SURFACE ( 'NONE', #25868, 0.5000000000000004441 ) ;
#22244=ORIENTED_EDGE ( 'NONE', *, *, #6913, .F. ) ;
#22245=AXIS2_PLACEMENT_3D ( 'NONE', #13719, #24172, #7969 ) ;
#22246=EDGE_CURVE ( 'NONE', #18764, #6939, #11978, .T. ) ;
#22247=ORIENTED_EDGE ( 'NONE', *, *, #24156, .F. ) ;
#22248=ORIENTED_EDGE ( 'NONE', *, *, #20430, .T. ) ;
#22251=EDGE_LOOP ( 'NONE', ( #25040, #17975, #19089, #8339 ) ) ;
#22252=AXIS2_PLACEMENT_3D ( 'NONE', #14820, #22792, #21475 ) ;
#22255=EDGE_CURVE ( 'NONE', #25532, #9390, #12526, .T. ) ;
#22256=DIRECTION ( 'NONE',  ( 1.000000000000000000, 0.000000000000000000, 0.000000000000000000 ) ) ;
#22264=AXIS2_PLACEMENT_3D ( 'NONE', #16800, #2923, #1706 ) ;
#22265=CARTESIAN_POINT ( 'NONE',  ( -20.20656826142249685, 23.64116323484259752, -6.500000000000000000 ) ) ;
#22267=CARTESIAN_POINT ( 'NONE',  ( -28.91604871112473418, -11.44867358849319849, -6.500000000000000000 ) ) ;
#22273=VERTEX_POINT ( 'NONE', #19710 ) ;
#22279=DIRECTION ( 'NONE',  ( 1.000000000000000000, 0.000000000000000000, 0.000000000000000000 ) ) ;
#22281=ADVANCED_FACE ( 'NONE', ( #14084 ), #23899, .F. ) ;
#22282=DIRECTION ( 'NONE',  ( 0.000000000000000000, 0.000000000000000000, 1.000000000000000000 ) ) ;
#22285=CARTESIAN_POINT ( 'NONE',  ( 0.000000000000000000, 0.000000000000000000, -6.500000000000000000 ) ) ;
#22288=DIRECTION ( 'NONE',  ( 0.000000000000000000, 0.000000000000000000, 1.000000000000000000 ) ) ;
#22292=ADVANCED_FACE ( 'NONE', ( #9647 ), #7939, .F. ) ;
#22297=CARTESIAN_POINT ( 'NONE',  ( -5.335677986745010593, -30.63887302793242284, -2.750000000000000000 ) ) ;
#22300=DIRECTION ( 'NONE',  ( 0.000000000000000000, 0.000000000000000000, 1.000000000000000000 ) ) ;
#22306=ORIENTED_EDGE ( 'NONE', *, *, #16401, .T. ) ;
#22309=DIRECTION ( 'NONE',  ( -0.06279051952931542779, -0.9980267284282714479, 0.000000000000000000 ) ) ;
#22312=VERTEX_POINT ( 'NONE', #4011 ) ;
#22319=DIRECTION ( 'NONE',  ( 0.000000000000000000, 0.000000000000000000, 1.000000000000000000 ) ) ;
#22321=DIRECTION ( 'NONE',  ( 0.000000000000000000, -0.000000000000000000, -1.000000000000000000 ) ) ;
#22331=ORIENTED_EDGE ( 'NONE', *, *, #5915, .F. ) ;
#22334=ORIENTED_EDGE ( 'NONE', *, *, #3063, .T. ) ;
#22351=CARTESIAN_POINT ( 'NONE',  ( -20.92219106202066925, -23.01025686871623321, 1.000000000000000000 ) ) ;
#22354=CARTESIAN_POINT ( 'NONE',  ( 16.66421332384664566, -26.25859848311276679, 1.000000000000000000 ) ) ;
#22361=DIRECTION ( 'NONE',  ( 0.000000000000000000, 0.000000000000000000, 1.000000000000000000 ) ) ;
#22364=LINE ( 'NONE', #547, #10848 ) ;
#22365=CARTESIAN_POINT ( 'NONE',  ( -5.335677986745010593, -30.63887302793242284, 1.000000000000000000 ) ) ;
#22367=ORIENTED_EDGE ( 'NONE', *, *, #15274, .F. ) ;
#22368=ORIENTED_EDGE ( 'NONE', *, *, #14009, .F. ) ;
#22371=VERTEX_POINT ( 'NONE', #22441 ) ;
#22372=DIRECTION ( 'NONE',  ( 1.000000000000000000, 0.000000000000000000, 0.000000000000000000 ) ) ;
#22374=CIRCLE ( 'NONE', #14452, 0.4999999999999998335 ) ;
#22386=DIRECTION ( 'NONE',  ( -0.3681245526846659843, 0.9297764858882561212, 0.000000000000000000 ) ) ;
#22391=DIRECTION ( 'NONE',  ( 1.000000000000000000, 0.000000000000000000, 0.000000000000000000 ) ) ;
#22394=ORIENTED_EDGE ( 'NONE', *, *, #19318, .T. ) ;
#22397=ORIENTED_EDGE ( 'NONE', *, *, #25329, .F. ) ;
#22398=DIRECTION ( 'NONE',  ( 0.000000000000000000, -0.000000000000000000, 1.000000000000000000 ) ) ;
#22400=DIRECTION ( 'NONE',  ( 0.000000000000000000, 0.000000000000000000, 1.000000000000000000 ) ) ;
#22401=ADVANCED_FACE ( 'NONE', ( #18782 ), #18539, .F. ) ;
#22403=CARTESIAN_POINT ( 'NONE',  ( 26.25859848311259981, -16.66421332384692278, 1.000000000000000000 ) ) ;
#22405=ORIENTED_EDGE ( 'NONE', *, *, #4843, .T. ) ;
#22409=CARTESIAN_POINT ( 'NONE',  ( -14.54246377227319442, 27.49048467073874491, -6.500000000000000000 ) ) ;
#22410=CARTESIAN_POINT ( 'NONE',  ( 0.000000000000000000, 0.000000000000000000, -6.500000000000000000 ) ) ;
#22412=DIRECTION ( 'NONE',  ( 0.000000000000000000, 0.000000000000000000, 1.000000000000000000 ) ) ;
#22415=CARTESIAN_POINT ( 'NONE',  ( 13.24173596767359662, -28.14012133169329388, -6.500000000000000000 ) ) ;
#22417=EDGE_CURVE ( 'NONE', #7673, #17013, #15471, .T. ) ;
#22418=FACE_OUTER_BOUND ( 'NONE', #20203, .T. ) ;
#22422=EDGE_LOOP ( 'NONE', ( #4871, #17771, #14431, #25808 ) ) ;
#22425=EDGE_CURVE ( 'NONE', #9975, #5761, #9591, .T. ) ;
#22427=ORIENTED_EDGE ( 'NONE', *, *, #576, .T. ) ;
#22430=CARTESIAN_POINT ( 'NONE',  ( -26.52310962334728828, 16.23990935651745460, -2.750000000000000000 ) ) ;
#22431=EDGE_CURVE ( 'NONE', #25550, #2880, #8350, .T. ) ;
#22432=CARTESIAN_POINT ( 'NONE',  ( 30.45149776762729488, 6.317933499823327637, -6.500000000000000000 ) ) ;
#22435=ORIENTED_EDGE ( 'NONE', *, *, #4394, .F. ) ;
#22439=CARTESIAN_POINT ( 'NONE',  ( -30.53863125411922752, 1.952785157361987878, 1.000000000000000000 ) ) ;
#22440=DIRECTION ( 'NONE',  ( 0.1873813145857330109, 0.9822872507286871668, 0.000000000000000000 ) ) ;
#22441=CARTESIAN_POINT ( 'NONE',  ( -5.335677986744341794, 30.63887302793254364, -6.500000000000000000 ) ) ;
#22444=DIRECTION ( 'NONE',  ( 0.000000000000000000, 0.000000000000000000, 1.000000000000000000 ) ) ;
#22446=DIRECTION ( 'NONE',  ( 0.9921147013144794302, 0.1253332335642911299, 0.000000000000000000 ) ) ;
#22447=CARTESIAN_POINT ( 'NONE',  ( -5.827558883616271501, -30.54913349766217934, 1.000000000000000000 ) ) ;
#22455=CARTESIAN_POINT ( 'NONE',  ( 0.000000000000000000, 0.000000000000000000, -6.500000000000000000 ) ) ;
#22462=DIRECTION ( 'NONE',  ( 0.000000000000000000, 0.000000000000000000, 1.000000000000000000 ) ) ;
#22466=ORIENTED_EDGE ( 'NONE', *, *, #14614, .T. ) ;
#22468=ORIENTED_EDGE ( 'NONE', *, *, #22094, .F. ) ;
#22471=EDGE_CURVE ( 'NONE', #24696, #4508, #22840, .T. ) ;
#22476=VECTOR ( 'NONE', #21468, 1000.000000000000000 ) ;
#22483=DIRECTION ( 'NONE',  ( 0.000000000000000000, -0.000000000000000000, 1.000000000000000000 ) ) ;
#22484=CYLINDRICAL_SURFACE ( 'NONE', #2441, 31.10000000000000142 ) ;
#22489=AXIS2_PLACEMENT_3D ( 'NONE', #6116, #8338, #16327 ) ;
#22490=LINE ( 'NONE', #9021, #23347 ) ;
#22493=DIRECTION ( 'NONE',  ( -0.1873813145857119722, 0.9822872507286911636, 0.000000000000000000 ) ) ;
#22494=DIRECTION ( 'NONE',  ( -0.000000000000000000, -0.000000000000000000, 1.000000000000000000 ) ) ;
#22496=CIRCLE ( 'NONE', #10423, 0.5000000000000001110 ) ;
#22497=ADVANCED_FACE ( 'NONE', ( #10928 ), #7142, .F. ) ;
#22499=VECTOR ( 'NONE', #19336, 1000.000000000000000 ) ;
#22500=VERTEX_POINT ( 'NONE', #13035 ) ;
#22505=ORIENTED_EDGE ( 'NONE', *, *, #7737, .T. ) ;
#22506=DIRECTION ( 'NONE',  ( 1.000000000000000000, 0.000000000000000000, 0.000000000000000000 ) ) ;
#22509=AXIS2_PLACEMENT_3D ( 'NONE', #19169, #7154, #25067 ) ;
#22512=CIRCLE ( 'NONE', #2826, 31.10000000000000142 ) ;
#22513=CARTESIAN_POINT ( 'NONE',  ( -3.897863563850083146, -30.85476721088024021, 1.000000000000000000 ) ) ;
#22518=DIRECTION ( 'NONE',  ( 1.000000000000000000, 0.000000000000000000, 0.000000000000000000 ) ) ;
#22519=CIRCLE ( 'NONE', #12928, 0.5000000000000005551 ) ;
#22528=EDGE_LOOP ( 'NONE', ( #6219, #3945, #23298, #13957 ) ) ;
#22530=CIRCLE ( 'NONE', #13755, 0.4999999999999996114 ) ;
#22531=ORIENTED_EDGE ( 'NONE', *, *, #846, .T. ) ;
#22532=LINE ( 'NONE', #6181, #19545 ) ;
#22533=ORIENTED_EDGE ( 'NONE', *, *, #17300, .T. ) ;
#22535=ORIENTED_EDGE ( 'NONE', *, *, #17469, .F. ) ;
#22537=AXIS2_PLACEMENT_3D ( 'NONE', #20440, #17982, #72 ) ;
#22541=ADVANCED_FACE ( 'NONE', ( #3336 ), #9841, .F. ) ;
#22542=FACE_OUTER_BOUND ( 'NONE', #18647, .T. ) ;
#22549=EDGE_CURVE ( 'NONE', #17200, #23624, #11669, .T. ) ;
#22550=AXIS2_PLACEMENT_3D ( 'NONE', #21134, #25313, #7143 ) ;
#22551=AXIS2_PLACEMENT_3D ( 'NONE', #1656, #21530, #9497 ) ;
#22568=ORIENTED_EDGE ( 'NONE', *, *, #7623, .T. ) ;
#22571=AXIS2_PLACEMENT_3D ( 'NONE', #13253, #977, #22935 ) ;
#22587=CARTESIAN_POINT ( 'NONE',  ( -29.41953157733080104, 10.08469938919530406, -6.500000000000000000 ) ) ;
#22595=AXIS2_PLACEMENT_3D ( 'NONE', #10062, #6272, #23934 ) ;
#22596=LINE ( 'NONE', #19046, #21252 ) ;
#22599=DIRECTION ( 'NONE',  ( -0.000000000000000000, -0.000000000000000000, 1.000000000000000000 ) ) ;
#22600=ORIENTED_EDGE ( 'NONE', *, *, #25661, .T. ) ;
#22601=CARTESIAN_POINT ( 'NONE',  ( 11.91206721063030649, -28.72825533807137433, -2.750000000000000000 ) ) ;
#22604=DIRECTION ( 'NONE',  ( 0.000000000000000000, 0.000000000000000000, 1.000000000000000000 ) ) ;
#22605=VERTEX_POINT ( 'NONE', #22000 ) ;
#22610=ORIENTED_EDGE ( 'NONE', *, *, #19449, .T. ) ;
#22611=ORIENTED_EDGE ( 'NONE', *, *, #7684, .F. ) ;
#22612=CARTESIAN_POINT ( 'NONE',  ( -16.66421332384701515, -26.25859848311253941, -6.500000000000000000 ) ) ;
#22620=FACE_OUTER_BOUND ( 'NONE', #25292, .T. ) ;
#22624=AXIS2_PLACEMENT_3D ( 'NONE', #25540, #13520, #2125 ) ;
#22625=DIRECTION ( 'NONE',  ( 1.000000000000000000, 0.000000000000000000, 0.000000000000000000 ) ) ;
#22629=CARTESIAN_POINT ( 'NONE',  ( 22.67092431280578779, -21.28941499438234786, 1.000000000000000000 ) ) ;
#22631=AXIS2_PLACEMENT_3D ( 'NONE', #7526, #15522, #23490 ) ;
#22633=AXIS2_PLACEMENT_3D ( 'NONE', #23047, #7463, #15203 ) ;
#22635=DIRECTION ( 'NONE',  ( 1.000000000000000000, 0.000000000000000000, 0.000000000000000000 ) ) ;
#22638=CARTESIAN_POINT ( 'NONE',  ( -2.451530025008687996, 31.00322564728517349, 1.000000000000000000 ) ) ;
#22641=CIRCLE ( 'NONE', #9678, 0.4999999999999996669 ) ;
#22642=ORIENTED_EDGE ( 'NONE', *, *, #2161, .T. ) ;
#22643=ORIENTED_EDGE ( 'NONE', *, *, #21773, .F. ) ;
#22646=CARTESIAN_POINT ( 'NONE',  ( -17.08421000182795879, -25.98730014090424234, -2.750000000000000000 ) ) ;
#22648=DIRECTION ( 'NONE',  ( 1.000000000000000000, 0.000000000000000000, 0.000000000000000000 ) ) ;
#22651=ADVANCED_FACE ( 'NONE', ( #12191 ), #8146, .F. ) ;
#22654=DIRECTION ( 'NONE',  ( -0.000000000000000000, -0.000000000000000000, -1.000000000000000000 ) ) ;
#22655=AXIS2_PLACEMENT_3D ( 'NONE', #2429, #24017, #24525 ) ;
#22661=DIRECTION ( 'NONE',  ( 1.000000000000000000, 0.000000000000000000, 0.000000000000000000 ) ) ;
#22664=DIRECTION ( 'NONE',  ( 0.000000000000000000, 0.000000000000000000, 1.000000000000000000 ) ) ;
#22666=CARTESIAN_POINT ( 'NONE',  ( 0.000000000000000000, 0.000000000000000000, -6.500000000000000000 ) ) ;
#22667=CIRCLE ( 'NONE', #8886, 0.4999999999999992784 ) ;
#22668=CARTESIAN_POINT ( 'NONE',  ( 0.000000000000000000, 0.000000000000000000, 1.000000000000000000 ) ) ;
#22669=ORIENTED_EDGE ( 'NONE', *, *, #2160, .F. ) ;
#22670=ADVANCED_FACE ( 'NONE', ( #2263 ), #23833, .F. ) ;
#22671=ORIENTED_EDGE ( 'NONE', *, *, #3970, .F. ) ;
#22673=AXIS2_PLACEMENT_3D ( 'NONE', #10250, #8661, #8795 ) ;
#22674=EDGE_CURVE ( 'NONE', #7996, #24829, #25078, .T. ) ;
#22675=ORIENTED_EDGE ( 'NONE', *, *, #16969, .T. ) ;
#22677=ORIENTED_EDGE ( 'NONE', *, *, #23832, .F. ) ;
#22679=EDGE_LOOP ( 'NONE', ( #444, #309, #20181, #21000 ) ) ;
#22681=VERTEX_POINT ( 'NONE', #22265 ) ;
#22682=FACE_OUTER_BOUND ( 'NONE', #22825, .T. ) ;
#22685=CARTESIAN_POINT ( 'NONE',  ( 0.000000000000000000, 0.000000000000000000, -6.500000000000000000 ) ) ;
#22686=CYLINDRICAL_SURFACE ( 'NONE', #8322, 31.10000000000000142 ) ;
#22688=EDGE_CURVE ( 'NONE', #585, #6457, #19634, .T. ) ;
#22689=AXIS2_PLACEMENT_3D ( 'NONE', #1827, #9791, #1946 ) ;
#22694=AXIS2_PLACEMENT_3D ( 'NONE', #18127, #464, #16543 ) ;
#22697=CYLINDRICAL_SURFACE ( 'NONE', #14183, 0.5000000000000002220 ) ;
#22700=DIRECTION ( 'NONE',  ( 1.000000000000000000, 0.000000000000000000, 0.000000000000000000 ) ) ;
#22701=EDGE_LOOP ( 'NONE', ( #12425, #20458, #23592, #21508 ) ) ;
#22709=ORIENTED_EDGE ( 'NONE', *, *, #3230, .F. ) ;
#22716=AXIS2_PLACEMENT_3D ( 'NONE', #11025, #6972, #4882 ) ;
#22717=CARTESIAN_POINT ( 'NONE',  ( -9.610428525060479288, 29.57785765677940404, 1.000000000000000000 ) ) ;
#22722=DIRECTION ( 'NONE',  ( 1.000000000000000000, 0.000000000000000000, 0.000000000000000000 ) ) ;
#22729=CARTESIAN_POINT ( 'NONE',  ( 27.92360179968377309, 13.69242354489143665, -6.500000000000000000 ) ) ;
#22737=CARTESIAN_POINT ( 'NONE',  ( 11.44867358849329619, -28.91604871112469510, -6.500000000000000000 ) ) ;
#22740=VERTEX_POINT ( 'NONE', #18714 ) ;
#22742=ORIENTED_EDGE ( 'NONE', *, *, #18605, .T. ) ;
#22743=EDGE_CURVE ( 'NONE', #3260, #7134, #13798, .T. ) ;
#22745=DIRECTION ( 'NONE',  ( 1.000000000000000000, 0.000000000000000000, 0.000000000000000000 ) ) ;
#22751=CARTESIAN_POINT ( 'NONE',  ( 0.000000000000000000, 0.000000000000000000, 1.000000000000000000 ) ) ;
#22753=DIRECTION ( 'NONE',  ( -0.000000000000000000, -0.000000000000000000, 1.000000000000000000 ) ) ;
#22758=CYLINDRICAL_SURFACE ( 'NONE', #7618, 0.5000000000000004441 ) ;
#22762=CARTESIAN_POINT ( 'NONE',  ( -30.54913349766228592, -5.827558883615738594, -6.500000000000000000 ) ) ;
#22764=EDGE_LOOP ( 'NONE', ( #20764, #7636, #19350, #14443 ) ) ;
#22765=DIRECTION ( 'NONE',  ( 1.000000000000000000, 0.000000000000000000, 0.000000000000000000 ) ) ;
#22766=LINE ( 'NONE', #24974, #21684 ) ;
#22767=ORIENTED_EDGE ( 'NONE', *, *, #19790, .F. ) ;
#22768=EDGE_CURVE ( 'NONE', #14948, #24264, #4611, .T. ) ;
#22769=ORIENTED_EDGE ( 'NONE', *, *, #19234, .F. ) ;
#22771=ORIENTED_EDGE ( 'NONE', *, *, #8496, .T. ) ;
#22772=ADVANCED_FACE ( 'NONE', ( #24479 ), #24601, .F. ) ;
#22776=ORIENTED_EDGE ( 'NONE', *, *, #1724, .F. ) ;
#22777=CARTESIAN_POINT ( 'NONE',  ( 26.52310962334750855, 16.23990935651707801, -6.500000000000000000 ) ) ;
#22780=CARTESIAN_POINT ( 'NONE',  ( -28.41604871112448549, 11.44867358849382910, 1.000000000000000000 ) ) ;
#22788=LINE ( 'NONE', #2514, #10089 ) ;
#22792=DIRECTION ( 'NONE',  ( 0.000000000000000000, 0.000000000000000000, 1.000000000000000000 ) ) ;
#22793=VERTEX_POINT ( 'NONE', #1069 ) ;
#22796=ORIENTED_EDGE ( 'NONE', *, *, #1133, .F. ) ;
#22798=EDGE_LOOP ( 'NONE', ( #515, #24167, #18644, #3681 ) ) ;
#22802=CARTESIAN_POINT ( 'NONE',  ( 20.92219106202050583, 23.01025686871638598, -2.750000000000000000 ) ) ;
#22803=EDGE_CURVE ( 'NONE', #15051, #383, #16736, .T. ) ;
#22807=EDGE_CURVE ( 'NONE', #14523, #4678, #5747, .T. ) ;
#22813=CARTESIAN_POINT ( 'NONE',  ( -27.00874656207289348, 15.41874213889432887, 1.000000000000000000 ) ) ;
#22817=VERTEX_POINT ( 'NONE', #11247 ) ;
#22819=DIRECTION ( 'NONE',  ( 1.000000000000000000, 0.000000000000000000, 0.000000000000000000 ) ) ;
#22821=DIRECTION ( 'NONE',  ( 0.000000000000000000, 0.000000000000000000, 1.000000000000000000 ) ) ;
#22825=EDGE_LOOP ( 'NONE', ( #14380, #14728, #10596, #11972 ) ) ;
#22826=ADVANCED_FACE ( 'NONE', ( #15315 ), #7214, .T. ) ;
#22827=ORIENTED_EDGE ( 'NONE', *, *, #25723, .F. ) ;
#22830=EDGE_CURVE ( 'NONE', #8878, #4940, #21330, .T. ) ;
#22831=DIRECTION ( 'NONE',  ( -0.000000000000000000, 0.000000000000000000, 1.000000000000000000 ) ) ;
#22834=DIRECTION ( 'NONE',  ( 0.9685831611286301879, -0.2486898871648584586, 0.000000000000000000 ) ) ;
#22836=DIRECTION ( 'NONE',  ( -0.7705132427757840352, 0.6374239897486960738, 0.000000000000000000 ) ) ;
#22838=ADVANCED_FACE ( 'NONE', ( #11773 ), #3794, .T. ) ;
#22840=LINE ( 'NONE', #9093, #11268 ) ;
#22843=CYLINDRICAL_SURFACE ( 'NONE', #21770, 0.5000000000000004441 ) ;
#22849=DIRECTION ( 'NONE',  ( 0.000000000000000000, -0.000000000000000000, 1.000000000000000000 ) ) ;
#22851=CARTESIAN_POINT ( 'NONE',  ( 0.4999838450259764255, -31.09598070739550124, 1.000000000000000000 ) ) ;
#22853=DIRECTION ( 'NONE',  ( 0.000000000000000000, 0.000000000000000000, 1.000000000000000000 ) ) ;
#22858=DIRECTION ( 'NONE',  ( 0.8090169943749474513, -0.5877852522924730261, 0.000000000000000000 ) ) ;
#22859=ORIENTED_EDGE ( 'NONE', *, *, #3740, .T. ) ;
#22861=ORIENTED_EDGE ( 'NONE', *, *, #20313, .T. ) ;
#22863=ORIENTED_EDGE ( 'NONE', *, *, #6317, .T. ) ;
#22866=EDGE_CURVE ( 'NONE', #17279, #7474, #1687, .T. ) ;
#22870=DIRECTION ( 'NONE',  ( 0.1873813145857330109, 0.9822872507286871668, 0.000000000000000000 ) ) ;
#22873=DIRECTION ( 'NONE',  ( 0.000000000000000000, 0.000000000000000000, 1.000000000000000000 ) ) ;
#22876=DIRECTION ( 'NONE',  ( 0.000000000000000000, 0.000000000000000000, -1.000000000000000000 ) ) ;
#22882=DIRECTION ( 'NONE',  ( 1.000000000000000000, 0.000000000000000000, 0.000000000000000000 ) ) ;
#22887=ORIENTED_EDGE ( 'NONE', *, *, #7037, .T. ) ;
#22889=CIRCLE ( 'NONE', #7445, 0.4999999999999997224 ) ;
#22890=ORIENTED_EDGE ( 'NONE', *, *, #6520, .F. ) ;
#22893=LINE ( 'NONE', #20940, #10529 ) ;
#22894=AXIS2_PLACEMENT_3D ( 'NONE', #24787, #13018, #18905 ) ;
#22897=CYLINDRICAL_SURFACE ( 'NONE', #24777, 31.10000000000000142 ) ;
#22905=CIRCLE ( 'NONE', #17061, 0.5000000000000002220 ) ;
#22907=FACE_OUTER_BOUND ( 'NONE', #9026, .T. ) ;
#22910=CYLINDRICAL_SURFACE ( 'NONE', #15951, 31.10000000000000142 ) ;
#22913=AXIS2_PLACEMENT_3D ( 'NONE', #15081, #20701, #17308 ) ;
#22914=DIRECTION ( 'NONE',  ( 1.000000000000000000, 0.000000000000000000, 0.000000000000000000 ) ) ;
#22915=CIRCLE ( 'NONE', #25422, 31.10000000000000142 ) ;
#22916=CARTESIAN_POINT ( 'NONE',  ( -10.94867358849371541, -28.91604871112453168, -6.500000000000000000 ) ) ;
#22918=ORIENTED_EDGE ( 'NONE', *, *, #8020, .F. ) ;
#22919=ORIENTED_EDGE ( 'NONE', *, *, #10822, .T. ) ;
#22922=CARTESIAN_POINT ( 'NONE',  ( -17.08421000182784866, -25.98730014090430984, 1.000000000000000000 ) ) ;
#22923=EDGE_LOOP ( 'NONE', ( #18254, #15633, #193, #22742 ) ) ;
#22924=CARTESIAN_POINT ( 'NONE',  ( -16.66421332384646448, 26.25859848311288403, -6.500000000000000000 ) ) ;
#22929=CARTESIAN_POINT ( 'NONE',  ( -29.72853858738272592, 9.133673601486785643, 1.000000000000000000 ) ) ;
#22932=CYLINDRICAL_SURFACE ( 'NONE', #8415, 0.5000000000000004441 ) ;
#22933=LINE ( 'NONE', #6715, #14175 ) ;
#22935=DIRECTION ( 'NONE',  ( 1.000000000000000000, 0.000000000000000000, 0.000000000000000000 ) ) ;
#22938=EDGE_CURVE ( 'NONE', #18492, #6156, #21326, .T. ) ;
#22945=CIRCLE ( 'NONE', #11662, 0.4999999999999998335 ) ;
#22947=DIRECTION ( 'NONE',  ( 1.000000000000000000, 0.000000000000000000, 0.000000000000000000 ) ) ;
#22953=VERTEX_POINT ( 'NONE', #3272 ) ;
#22954=DIRECTION ( 'NONE',  ( 1.000000000000000000, 0.000000000000000000, 0.000000000000000000 ) ) ;
#22956=ORIENTED_EDGE ( 'NONE', *, *, #9041, .F. ) ;
#22958=DIRECTION ( 'NONE',  ( 0.4257792915650852050, 0.9048270524660135816, 0.000000000000000000 ) ) ;
#22959=CARTESIAN_POINT ( 'NONE',  ( 0.000000000000000000, 0.000000000000000000, -6.500000000000000000 ) ) ;
#22964=CIRCLE ( 'NONE', #25054, 31.10000000000000142 ) ;
#22965=ADVANCED_FACE ( 'NONE', ( #1330 ), #17291, .F. ) ;
#22969=DIRECTION ( 'NONE',  ( 0.000000000000000000, 0.000000000000000000, 1.000000000000000000 ) ) ;
#22973=VECTOR ( 'NONE', #14725, 1000.000000000000000 ) ;
#22980=AXIS2_PLACEMENT_3D ( 'NONE', #17027, #2770, #10731 ) ;
#22981=CARTESIAN_POINT ( 'NONE',  ( 23.96296185032695192, -19.82388608118436935, 1.000000000000000000 ) ) ;
#22986=DIRECTION ( 'NONE',  ( -0.7289686274214034478, 0.6845471059286972748, 0.000000000000000000 ) ) ;
#22989=DIRECTION ( 'NONE',  ( -0.000000000000000000, 0.000000000000000000, 1.000000000000000000 ) ) ;
#22990=VERTEX_POINT ( 'NONE', #22351 ) ;
#22992=EDGE_CURVE ( 'NONE', #8478, #10323, #2231, .T. ) ;
#22993=ORIENTED_EDGE ( 'NONE', *, *, #5525, .F. ) ;
#22995=EDGE_LOOP ( 'NONE', ( #2757, #1551, #5473, #5928 ) ) ;
#23001=CIRCLE ( 'NONE', #17167, 31.10000000000000142 ) ;
#23004=CARTESIAN_POINT ( 'NONE',  ( -29.07785765677936851, -9.610428525060582317, -6.500000000000000000 ) ) ;
#23013=CARTESIAN_POINT ( 'NONE',  ( 0.000000000000000000, 0.000000000000000000, -6.500000000000000000 ) ) ;
#23014=DIRECTION ( 'NONE',  ( 0.000000000000000000, -0.000000000000000000, 1.000000000000000000 ) ) ;
#23020=VECTOR ( 'NONE', #15992, 1000.000000000000000 ) ;
#23021=CARTESIAN_POINT ( 'NONE',  ( 5.335677986744567391, -30.63887302793249745, -2.750000000000000000 ) ) ;
#23023=ORIENTED_EDGE ( 'NONE', *, *, #9968, .F. ) ;
#23025=DIRECTION ( 'NONE',  ( 0.000000000000000000, 0.000000000000000000, 1.000000000000000000 ) ) ;
#23026=ORIENTED_EDGE ( 'NONE', *, *, #4246, .F. ) ;
#23027=CIRCLE ( 'NONE', #13829, 0.4999999999999993339 ) ;
#23030=VERTEX_POINT ( 'NONE', #394 ) ;
#23034=DIRECTION ( 'NONE',  ( 1.000000000000000000, 0.000000000000000000, 0.000000000000000000 ) ) ;
#23036=CIRCLE ( 'NONE', #15104, 0.5000000000000002220 ) ;
#23040=VECTOR ( 'NONE', #24820, 1000.000000000000000 ) ;
#23042=AXIS2_PLACEMENT_3D ( 'NONE', #14869, #6495, #12379 ) ;
#23046=CARTESIAN_POINT ( 'NONE',  ( -26.52310962334728828, 16.23990935651745460, -6.500000000000000000 ) ) ;
#23047=CARTESIAN_POINT ( 'NONE',  ( 30.85476721088027929, 3.897863563849760737, -6.500000000000000000 ) ) ;
#23048=DIRECTION ( 'NONE',  ( 0.000000000000000000, -0.000000000000000000, -1.000000000000000000 ) ) ;
#23056=ORIENTED_EDGE ( 'NONE', *, *, #15178, .T. ) ;
#23058=EDGE_LOOP ( 'NONE', ( #22677, #25412, #12390, #23319 ) ) ;
#23059=FACE_OUTER_BOUND ( 'NONE', #12589, .T. ) ;
#23060=EDGE_CURVE ( 'NONE', #15870, #23630, #9229, .T. ) ;
#23061=ORIENTED_EDGE ( 'NONE', *, *, #17070, .F. ) ;
#23062=FACE_OUTER_BOUND ( 'NONE', #21449, .T. ) ;
#23063=AXIS2_PLACEMENT_3D ( 'NONE', #11774, #12014, #2096 ) ;
#23064=AXIS2_PLACEMENT_3D ( 'NONE', #812, #12583, #571 ) ;
#23066=EDGE_CURVE ( 'NONE', #17442, #4475, #23432, .T. ) ;
#23067=DIRECTION ( 'NONE',  ( -0.000000000000000000, -0.000000000000000000, 1.000000000000000000 ) ) ;
#23070=AXIS2_PLACEMENT_3D ( 'NONE', #14054, #22152, #14563 ) ;
#23071=DIRECTION ( 'NONE',  ( 0.000000000000000000, -0.000000000000000000, 1.000000000000000000 ) ) ;
#23077=AXIS2_PLACEMENT_3D ( 'NONE', #23556, #13739, #8122 ) ;
#23080=VERTEX_POINT ( 'NONE', #15825 ) ;
#23084=EDGE_CURVE ( 'NONE', #8796, #16116, #20912, .T. ) ;
#23087=CARTESIAN_POINT ( 'NONE',  ( -17.87326343783906424, 25.45105997952945387, -2.750000000000000000 ) ) ;
#23088=ORIENTED_EDGE ( 'NONE', *, *, #20248, .T. ) ;
#23091=DIRECTION ( 'NONE',  ( 1.000000000000000000, 0.000000000000000000, 0.000000000000000000 ) ) ;
#23093=DIRECTION ( 'NONE',  ( 0.000000000000000000, 0.000000000000000000, 1.000000000000000000 ) ) ;
#23094=VERTEX_POINT ( 'NONE', #23798 ) ;
#23095=EDGE_CURVE ( 'NONE', #23505, #19518, #7138, .T. ) ;
#23097=DIRECTION ( 'NONE',  ( 1.000000000000000000, 0.000000000000000000, 0.000000000000000000 ) ) ;
#23100=AXIS2_PLACEMENT_3D ( 'NONE', #207, #2293, #18245 ) ;
#23101=DIRECTION ( 'NONE',  ( 0.9048270524660195768, -0.4257792915650726040, 0.000000000000000000 ) ) ;
#23105=CARTESIAN_POINT ( 'NONE',  ( 29.72853858738278987, -9.133673601486577809, -6.500000000000000000 ) ) ;
#23113=CYLINDRICAL_SURFACE ( 'NONE', #22509, 0.5000000000000004441 ) ;
#23120=LINE ( 'NONE', #10682, #18365 ) ;
#23124=EDGE_CURVE ( 'NONE', #6672, #1492, #11309, .T. ) ;
#23128=DIRECTION ( 'NONE',  ( 0.000000000000000000, 0.000000000000000000, 1.000000000000000000 ) ) ;
#23130=EDGE_CURVE ( 'NONE', #7738, #20939, #7981, .T. ) ;
#23131=CIRCLE ( 'NONE', #21447, 0.4999999999999999445 ) ;
#23141=CARTESIAN_POINT ( 'NONE',  ( -13.69242354489114177, 27.92360179968391165, -2.750000000000000000 ) ) ;
#23142=CARTESIAN_POINT ( 'NONE',  ( 0.000000000000000000, 0.000000000000000000, 1.000000000000000000 ) ) ;
#23150=DIRECTION ( 'NONE',  ( 1.000000000000000000, 0.000000000000000000, 0.000000000000000000 ) ) ;
#23153=EDGE_LOOP ( 'NONE', ( #20671, #23522, #7496, #16198 ) ) ;
#23154=ORIENTED_EDGE ( 'NONE', *, *, #8020, .T. ) ;
#23155=VERTEX_POINT ( 'NONE', #19989 ) ;
#23156=ORIENTED_EDGE ( 'NONE', *, *, #16714, .T. ) ;
#23160=CARTESIAN_POINT ( 'NONE',  ( 0.000000000000000000, 0.000000000000000000, -6.500000000000000000 ) ) ;
#23166=EDGE_CURVE ( 'NONE', #11885, #13215, #2858, .T. ) ;
#23169=DIRECTION ( 'NONE',  ( -0.6374239897486843054, 0.7705132427757935831, 0.000000000000000000 ) ) ;
#23176=ORIENTED_EDGE ( 'NONE', *, *, #9394, .T. ) ;
#23177=VERTEX_POINT ( 'NONE', #12805 ) ;
#23180=ORIENTED_EDGE ( 'NONE', *, *, #10022, .F. ) ;
#23181=DIRECTION ( 'NONE',  ( 0.000000000000000000, 0.000000000000000000, 1.000000000000000000 ) ) ;
#23182=ORIENTED_EDGE ( 'NONE', *, *, #20091, .F. ) ;
#23186=DIRECTION ( 'NONE',  ( 0.000000000000000000, 0.000000000000000000, 1.000000000000000000 ) ) ;
#23187=EDGE_CURVE ( 'NONE', #15991, #20076, #655, .T. ) ;
#23188=CYLINDRICAL_SURFACE ( 'NONE', #18014, 0.5000000000000004441 ) ;
#23192=EDGE_CURVE ( 'NONE', #17006, #13301, #14778, .T. ) ;
#23195=CARTESIAN_POINT ( 'NONE',  ( -4.393401135980685268, 30.78811501957149588, -2.750000000000000000 ) ) ;
#23197=ORIENTED_EDGE ( 'NONE', *, *, #6435, .T. ) ;
#23199=SHAPE_REPRESENTATION ( 'bezel', ( #21036 ), #23570 ) ;
#23201=EDGE_LOOP ( 'NONE', ( #4734, #2626, #20607, #17105 ) ) ;
#23202=FACE_OUTER_BOUND ( 'NONE', #24204, .T. ) ;
#23204=CARTESIAN_POINT ( 'NONE',  ( -31.09598070739550835, -0.4999838450256507416, 1.000000000000000000 ) ) ;
#23205=ORIENTED_EDGE ( 'NONE', *, *, #15211, .T. ) ;
#23206=ORIENTED_EDGE ( 'NONE', *, *, #1215, .F. ) ;
#23208=CARTESIAN_POINT ( 'NONE',  ( 20.20656826142273843, 23.64116323484239146, 1.000000000000000000 ) ) ;
#23209=VERTEX_POINT ( 'NONE', #18685 ) ;
#23214=CIRCLE ( 'NONE', #11932, 0.5000000000000005551 ) ;
#23215=DIRECTION ( 'NONE',  ( 0.000000000000000000, 0.000000000000000000, 1.000000000000000000 ) ) ;
#23217=ADVANCED_FACE ( 'NONE', ( #16876 ), #9012, .T. ) ;
#23221=DIRECTION ( 'NONE',  ( 0.000000000000000000, 0.000000000000000000, -1.000000000000000000 ) ) ;
#23222=DIRECTION ( 'NONE',  ( 0.000000000000000000, 0.000000000000000000, 1.000000000000000000 ) ) ;
#23227=EDGE_CURVE ( 'NONE', #8694, #15051, #15913, .T. ) ;
#23233=VERTEX_POINT ( 'NONE', #24564 ) ;
#23234=CYLINDRICAL_SURFACE ( 'NONE', #25553, 0.5000000000000000000 ) ;
#23238=ORIENTED_EDGE ( 'NONE', *, *, #25751, .F. ) ;
#23240=ORIENTED_EDGE ( 'NONE', *, *, #1697, .F. ) ;
#23242=ORIENTED_EDGE ( 'NONE', *, *, #20926, .F. ) ;
#23251=DIRECTION ( 'NONE',  ( -0.000000000000000000, 0.000000000000000000, 1.000000000000000000 ) ) ;
#23253=CARTESIAN_POINT ( 'NONE',  ( 14.98253926456337837, 27.25313774936414291, 1.000000000000000000 ) ) ;
#23259=CARTESIAN_POINT ( 'NONE',  ( 0.000000000000000000, 0.000000000000000000, 1.000000000000000000 ) ) ;
#23263=CARTESIAN_POINT ( 'NONE',  ( -2.451530025008687996, 31.00322564728517349, -6.500000000000000000 ) ) ;
#23264=ORIENTED_EDGE ( 'NONE', *, *, #7267, .F. ) ;
#23266=CARTESIAN_POINT ( 'NONE',  ( 0.000000000000000000, 0.000000000000000000, -6.500000000000000000 ) ) ;
#23269=EDGE_CURVE ( 'NONE', #24827, #21865, #4952, .T. ) ;
#23270=ORIENTED_EDGE ( 'NONE', *, *, #14865, .F. ) ;
#23271=EDGE_CURVE ( 'NONE', #21953, #3228, #7558, .T. ) ;
#23273=ORIENTED_EDGE ( 'NONE', *, *, #15842, .F. ) ;
#23275=DIRECTION ( 'NONE',  ( 0.000000000000000000, 0.000000000000000000, 1.000000000000000000 ) ) ;
#23277=DIRECTION ( 'NONE',  ( 1.000000000000000000, 0.000000000000000000, 0.000000000000000000 ) ) ;
#23278=DIRECTION ( 'NONE',  ( 1.000000000000000000, 0.000000000000000000, 0.000000000000000000 ) ) ;
#23283=CARTESIAN_POINT ( 'NONE',  ( 1.453535542772610212, 31.06601413805602263, -2.750000000000000000 ) ) ;
#23286=DIRECTION ( 'NONE',  ( -0.000000000000000000, -0.000000000000000000, 1.000000000000000000 ) ) ;
#23288=CYLINDRICAL_SURFACE ( 'NONE', #24717, 31.10000000000000142 ) ;
#23292=DIRECTION ( 'NONE',  ( 0.000000000000000000, 0.000000000000000000, 1.000000000000000000 ) ) ;
#23293=AXIS2_PLACEMENT_3D ( 'NONE', #5667, #1884, #9846 ) ;
#23294=CARTESIAN_POINT ( 'NONE',  ( 5.827558883616049457, 30.54913349766221842, 1.000000000000000000 ) ) ;
#23296=VERTEX_POINT ( 'NONE', #4560 ) ;
#23298=ORIENTED_EDGE ( 'NONE', *, *, #2160, .T. ) ;
#23301=ORIENTED_EDGE ( 'NONE', *, *, #21226, .T. ) ;
#23308=DIRECTION ( 'NONE',  ( 0.000000000000000000, 0.000000000000000000, 1.000000000000000000 ) ) ;
#23309=VECTOR ( 'NONE', #3937, 1000.000000000000000 ) ;
#23310=LINE ( 'NONE', #11415, #15511 ) ;
#23311=LINE ( 'NONE', #19127, #5412 ) ;
#23313=CARTESIAN_POINT ( 'NONE',  ( 14.54246377227358877, 27.49048467073853175, -6.500000000000000000 ) ) ;
#23317=CARTESIAN_POINT ( 'NONE',  ( 31.03863125411924173, -1.952785157361756951, -6.500000000000000000 ) ) ;
#23319=ORIENTED_EDGE ( 'NONE', *, *, #7863, .T. ) ;
#23323=ORIENTED_EDGE ( 'NONE', *, *, #5924, .F. ) ;
#23326=CIRCLE ( 'NONE', #12044, 31.10000000000000142 ) ;
#23332=LINE ( 'NONE', #13656, #6469 ) ;
#23336=CARTESIAN_POINT ( 'NONE',  ( 25.45105997952913057, -17.87326343783952254, -2.750000000000000000 ) ) ;
#23338=CARTESIAN_POINT ( 'NONE',  ( 13.24173596767378847, 28.14012133169319796, -6.500000000000000000 ) ) ;
#23340=AXIS2_PLACEMENT_3D ( 'NONE', #24815, #4925, #20886 ) ;
#23344=VECTOR ( 'NONE', #18382, 1000.000000000000000 ) ;
#23345=DIRECTION ( 'NONE',  ( 0.000000000000000000, 0.000000000000000000, 1.000000000000000000 ) ) ;
#23347=VECTOR ( 'NONE', #9524, 1000.000000000000000 ) ;
#23351=DIRECTION ( 'NONE',  ( 0.000000000000000000, 0.000000000000000000, -1.000000000000000000 ) ) ;
#23354=EDGE_CURVE ( 'NONE', #22067, #17688, #14256, .T. ) ;
#23357=VERTEX_POINT ( 'NONE', #13460 ) ;
#23362=CARTESIAN_POINT ( 'NONE',  ( 24.27856662945499266, 19.43607991388990186, 1.000000000000000000 ) ) ;
#23363=ORIENTED_EDGE ( 'NONE', *, *, #24006, .T. ) ;
#23365=CIRCLE ( 'NONE', #17527, 0.4999999999999983902 ) ;
#23366=EDGE_CURVE ( 'NONE', #23357, #7134, #13194, .T. ) ;
#23367=CIRCLE ( 'NONE', #12083, 0.5000000000000017764 ) ;
#23370=EDGE_LOOP ( 'NONE', ( #12557, #10987, #9861, #11933 ) ) ;
#23372=EDGE_CURVE ( 'NONE', #12921, #12737, #47, .T. ) ;
#23373=CARTESIAN_POINT ( 'NONE',  ( 0.000000000000000000, 0.000000000000000000, -6.500000000000000000 ) ) ;
#23380=DIRECTION ( 'NONE',  ( 1.000000000000000000, 0.000000000000000000, 0.000000000000000000 ) ) ;
#23387=CYLINDRICAL_SURFACE ( 'NONE', #12902, 31.10000000000000142 ) ;
#23396=VERTEX_POINT ( 'NONE', #11093 ) ;
#23400=EDGE_LOOP ( 'NONE', ( #13484, #24260, #16950, #18700 ) ) ;
#23401=ORIENTED_EDGE ( 'NONE', *, *, #16311, .F. ) ;
#23402=VECTOR ( 'NONE', #3075, 1000.000000000000000 ) ;
#23403=ORIENTED_EDGE ( 'NONE', *, *, #18173, .F. ) ;
#23404=ORIENTED_EDGE ( 'NONE', *, *, #14434, .T. ) ;
#23405=ORIENTED_EDGE ( 'NONE', *, *, #12831, .T. ) ;
#23406=CARTESIAN_POINT ( 'NONE',  ( 25.16042852506090810, 18.28012134629586072, -6.500000000000000000 ) ) ;
#23409=AXIS2_PLACEMENT_3D ( 'NONE', #10892, #1222, #21367 ) ;
#23411=CARTESIAN_POINT ( 'NONE',  ( -9.610428525060479288, 29.57785765677940404, -6.500000000000000000 ) ) ;
#23418=AXIS2_PLACEMENT_3D ( 'NONE', #20426, #8160, #10495 ) ;
#23421=DIRECTION ( 'NONE',  ( 1.000000000000000000, 0.000000000000000000, 0.000000000000000000 ) ) ;
#23422=CYLINDRICAL_SURFACE ( 'NONE', #18062, 31.10000000000000142 ) ;
#23424=VECTOR ( 'NONE', #3160, 1000.000000000000000 ) ;
#23428=ORIENTED_EDGE ( 'NONE', *, *, #10821, .T. ) ;
#23429=DIRECTION ( 'NONE',  ( 0.000000000000000000, -0.000000000000000000, -1.000000000000000000 ) ) ;
#23430=VECTOR ( 'NONE', #14978, 1000.000000000000000 ) ;
#23432=CIRCLE ( 'NONE', #22595, 31.10000000000000142 ) ;
#23434=DIRECTION ( 'NONE',  ( 1.000000000000000000, 0.000000000000000000, 0.000000000000000000 ) ) ;
#23435=ORIENTED_EDGE ( 'NONE', *, *, #21165, .F. ) ;
#23437=ORIENTED_EDGE ( 'NONE', *, *, #10643, .T. ) ;
#23439=VECTOR ( 'NONE', #974, 1000.000000000000000 ) ;
#23445=EDGE_CURVE ( 'NONE', #14404, #24819, #6719, .T. ) ;
#23448=CARTESIAN_POINT ( 'NONE',  ( -18.68225429291740269, -24.86329371854762016, 1.000000000000000000 ) ) ;
#23450=VECTOR ( 'NONE', #14604, 1000.000000000000000 ) ;
#23455=AXIS2_PLACEMENT_3D ( 'NONE', #22403, #18008, #8422 ) ;
#23456=ORIENTED_EDGE ( 'NONE', *, *, #23130, .T. ) ;
#23457=ORIENTED_EDGE ( 'NONE', *, *, #19124, .T. ) ;
#23462=ORIENTED_EDGE ( 'NONE', *, *, #10386, .F. ) ;
#23468=AXIS2_PLACEMENT_3D ( 'NONE', #3133, #11100, #1158 ) ;
#23472=EDGE_CURVE ( 'NONE', #7696, #1446, #15283, .T. ) ;
#23475=CIRCLE ( 'NONE', #8867, 0.4999999999999991673 ) ;
#23483=VECTOR ( 'NONE', #6762, 1000.000000000000000 ) ;
#23484=EDGE_CURVE ( 'NONE', #8412, #4038, #17571, .T. ) ;
#23485=FACE_OUTER_BOUND ( 'NONE', #9710, .T. ) ;
#23487=DIRECTION ( 'NONE',  ( 0.000000000000000000, 0.000000000000000000, 1.000000000000000000 ) ) ;
#23490=DIRECTION ( 'NONE',  ( -0.1253332335642912687, 0.9921147013144795412, 0.000000000000000000 ) ) ;
#23494=EDGE_LOOP ( 'NONE', ( #13341, #6736, #450, #22887 ) ) ;
#23498=ORIENTED_EDGE ( 'NONE', *, *, #20736, .F. ) ;
#23501=DIRECTION ( 'NONE',  ( 0.000000000000000000, 0.000000000000000000, 1.000000000000000000 ) ) ;
#23504=ORIENTED_EDGE ( 'NONE', *, *, #25617, .T. ) ;
#23505=VERTEX_POINT ( 'NONE', #5850 ) ;
#23506=CARTESIAN_POINT ( 'NONE',  ( -17.08421000182742233, 25.98730014090460472, -6.500000000000000000 ) ) ;
#23508=AXIS2_PLACEMENT_3D ( 'NONE', #8429, #6461, #4367 ) ;
#23509=DIRECTION ( 'NONE',  ( -0.000000000000000000, 0.000000000000000000, 1.000000000000000000 ) ) ;
#23510=CIRCLE ( 'NONE', #17682, 0.4999999999999993339 ) ;
#23511=ADVANCED_FACE ( 'NONE', ( #13967 ), #6105, .T. ) ;
#23513=SHAPE_REPRESENTATION_RELATIONSHIP ( 'NONE' , 'NONE' ,  #23199, #16592 ) ;
#23519=CARTESIAN_POINT ( 'NONE',  ( -1.952785157361865753, -31.03863125411923463, 1.000000000000000000 ) ) ;
#23520=CARTESIAN_POINT ( 'NONE',  ( -26.75313774936397948, 14.98253926456367502, -6.500000000000000000 ) ) ;
#23522=ORIENTED_EDGE ( 'NONE', *, *, #1314, .T. ) ;
#23524=DIRECTION ( 'NONE',  ( 0.000000000000000000, 0.000000000000000000, 1.000000000000000000 ) ) ;
#23528=CARTESIAN_POINT ( 'NONE',  ( 0.000000000000000000, 0.000000000000000000, 1.000000000000000000 ) ) ;
#23533=DIRECTION ( 'NONE',  ( -0.3090169943749528914, -0.9510565162951518658, 0.000000000000000000 ) ) ;
#23535=AXIS2_PLACEMENT_3D ( 'NONE', #20338, #4910, #24413 ) ;
#23537=ORIENTED_EDGE ( 'NONE', *, *, #1844, .F. ) ;
#23538=EDGE_LOOP ( 'NONE', ( #8802, #17281, #8156, #12058 ) ) ;
#23542=CARTESIAN_POINT ( 'NONE',  ( 30.63887302793245482, 5.335677986744801871, 1.000000000000000000 ) ) ;
#23547=CARTESIAN_POINT ( 'NONE',  ( -30.78811501957138930, 4.393401135981437555, -2.750000000000000000 ) ) ;
#23548=CIRCLE ( 'NONE', #6040, 31.10000000000000142 ) ;
#23550=CIRCLE ( 'NONE', #12274, 31.10000000000000142 ) ;
#23554=CARTESIAN_POINT ( 'NONE',  ( 5.335677986744568280, -30.63887302793249745, -6.500000000000000000 ) ) ;
#23555=CYLINDRICAL_SURFACE ( 'NONE', #22056, 31.10000000000000142 ) ;
#23556=CARTESIAN_POINT ( 'NONE',  ( 0.000000000000000000, 0.000000000000000000, -6.500000000000000000 ) ) ;
#23557=EDGE_CURVE ( 'NONE', #583, #1666, #8818, .T. ) ;
#23560=DIRECTION ( 'NONE',  ( 0.000000000000000000, 0.000000000000000000, 1.000000000000000000 ) ) ;
#23561=DIRECTION ( 'NONE',  ( -0.000000000000000000, 0.000000000000000000, -1.000000000000000000 ) ) ;
#23563=ORIENTED_EDGE ( 'NONE', *, *, #5551, .T. ) ;
#23565=DIRECTION ( 'NONE',  ( 0.8443279255020154084, -0.5358267949789962126, 0.000000000000000000 ) ) ;
#23566=ORIENTED_EDGE ( 'NONE', *, *, #19677, .T. ) ;
#23568=VERTEX_POINT ( 'NONE', #12254 ) ;
#23570=( GEOMETRIC_REPRESENTATION_CONTEXT ( 3 ) GLOBAL_UNCERTAINTY_ASSIGNED_CONTEXT ( ( #18824 ) ) GLOBAL_UNIT_ASSIGNED_CONTEXT ( ( #9270, #1812, #21543 ) ) REPRESENTATION_CONTEXT ( 'NONE', 'WORKASPACE' ) );
#23577=CARTESIAN_POINT ( 'NONE',  ( -24.86329371854788661, -18.68225429291705098, -2.750000000000000000 ) ) ;
#23578=FACE_OUTER_BOUND ( 'NONE', #17517, .T. ) ;
#23586=ORIENTED_EDGE ( 'NONE', *, *, #20696, .T. ) ;
#23587=EDGE_CURVE ( 'NONE', #24730, #24433, #19649, .T. ) ;
#23591=EDGE_CURVE ( 'NONE', #5929, #6393, #8326, .T. ) ;
#23592=ORIENTED_EDGE ( 'NONE', *, *, #12007, .T. ) ;
#23593=CYLINDRICAL_SURFACE ( 'NONE', #17112, 31.10000000000000142 ) ;
#23595=CARTESIAN_POINT ( 'NONE',  ( 9.610428525060671134, -29.57785765677934009, 1.000000000000000000 ) ) ;
#23597=ORIENTED_EDGE ( 'NONE', *, *, #7734, .T. ) ;
#23600=VERTEX_POINT ( 'NONE', #8204 ) ;
#23609=AXIS2_PLACEMENT_3D ( 'NONE', #20138, #6803, #14785 ) ;
#23618=DIRECTION ( 'NONE',  ( 0.000000000000000000, 0.000000000000000000, 1.000000000000000000 ) ) ;
#23624=VERTEX_POINT ( 'NONE', #21673 ) ;
#23626=FACE_BOUND ( 'NONE', #16145, .T. ) ;
#23627=ORIENTED_EDGE ( 'NONE', *, *, #13384, .T. ) ;
#23629=CIRCLE ( 'NONE', #8173, 0.4999999999999999445 ) ;
#23630=VERTEX_POINT ( 'NONE', #14224 ) ;
#23632=CARTESIAN_POINT ( 'NONE',  ( 3.401318489841097747, 30.91344420362547396, -2.750000000000000000 ) ) ;
#23641=DIRECTION ( 'NONE',  ( 1.000000000000000000, 0.000000000000000000, 0.000000000000000000 ) ) ;
#23642=LINE ( 'NONE', #25609, #18397 ) ;
#23647=DIRECTION ( 'NONE',  ( -0.9822872507286872779, 0.1873813145857327056, 0.000000000000000000 ) ) ;
#23650=DIRECTION ( 'NONE',  ( 0.000000000000000000, 0.000000000000000000, 1.000000000000000000 ) ) ;
#23652=ORIENTED_EDGE ( 'NONE', *, *, #19386, .F. ) ;
#23654=DIRECTION ( 'NONE',  ( -0.000000000000000000, 0.000000000000000000, -1.000000000000000000 ) ) ;
#23656=VERTEX_POINT ( 'NONE', #4916 ) ;
#23659=ORIENTED_EDGE ( 'NONE', *, *, #21306, .T. ) ;
#23660=EDGE_CURVE ( 'NONE', #13603, #25184, #18433, .T. ) ;
#23661=EDGE_LOOP ( 'NONE', ( #5766, #5421, #6415, #10744 ) ) ;
#23670=DIRECTION ( 'NONE',  ( 0.000000000000000000, 0.000000000000000000, 1.000000000000000000 ) ) ;
#23671=DIRECTION ( 'NONE',  ( 0.000000000000000000, -0.000000000000000000, -1.000000000000000000 ) ) ;
#23683=ORIENTED_EDGE ( 'NONE', *, *, #2804, .F. ) ;
#23684=FACE_OUTER_BOUND ( 'NONE', #17514, .T. ) ;
#23689=EDGE_CURVE ( 'NONE', #22273, #5799, #24702, .T. ) ;
#23690=ORIENTED_EDGE ( 'NONE', *, *, #10022, .T. ) ;
#23691=ADVANCED_FACE ( 'NONE', ( #14868 ), #22843, .F. ) ;
#23693=LINE ( 'NONE', #7867, #9735 ) ;
#23695=FACE_OUTER_BOUND ( 'NONE', #14165, .T. ) ;
#23704=EDGE_LOOP ( 'NONE', ( #8663, #5357, #21345, #6042 ) ) ;
#23705=EDGE_LOOP ( 'NONE', ( #10847, #7931, #3884, #9028 ) ) ;
#23708=DIRECTION ( 'NONE',  ( 0.000000000000000000, 0.000000000000000000, 1.000000000000000000 ) ) ;
#23710=DIRECTION ( 'NONE',  ( 0.000000000000000000, 0.000000000000000000, 1.000000000000000000 ) ) ;
#23712=VERTEX_POINT ( 'NONE', #14478 ) ;
#23713=CIRCLE ( 'NONE', #9097, 0.4999999999999998890 ) ;
#23714=DIRECTION ( 'NONE',  ( 0.000000000000000000, 0.000000000000000000, 1.000000000000000000 ) ) ;
#23716=CARTESIAN_POINT ( 'NONE',  ( 1.453535542772610212, 31.06601413805602263, 1.000000000000000000 ) ) ;
#23719=AXIS2_PLACEMENT_3D ( 'NONE', #273, #21975, #1719 ) ;
#23720=DIRECTION ( 'NONE',  ( 0.000000000000000000, 0.000000000000000000, 1.000000000000000000 ) ) ;
#23722=ADVANCED_FACE ( 'NONE', ( #2825 ), #2703, .F. ) ;
#23723=EDGE_CURVE ( 'NONE', #9415, #10323, #483, .T. ) ;
#23725=CARTESIAN_POINT ( 'NONE',  ( 16.23990935651717393, 26.52310962334745170, 1.000000000000000000 ) ) ;
#23728=AXIS2_PLACEMENT_3D ( 'NONE', #15519, #23487, #15897 ) ;
#23729=CARTESIAN_POINT ( 'NONE',  ( 0.000000000000000000, 0.000000000000000000, 1.000000000000000000 ) ) ;
#23736=DIRECTION ( 'NONE',  ( -0.000000000000000000, 0.000000000000000000, -1.000000000000000000 ) ) ;
#23738=AXIS2_PLACEMENT_3D ( 'NONE', #15288, #9517, #11356 ) ;
#23748=ORIENTED_EDGE ( 'NONE', *, *, #23084, .T. ) ;
#23749=ORIENTED_EDGE ( 'NONE', *, *, #8496, .F. ) ;
#23750=DIRECTION ( 'NONE',  ( 0.000000000000000000, -0.000000000000000000, 1.000000000000000000 ) ) ;
#23752=VECTOR ( 'NONE', #18584, 1000.000000000000000 ) ;
#23753=EDGE_CURVE ( 'NONE', #22016, #17650, #1317, .T. ) ;
#23754=AXIS2_PLACEMENT_3D ( 'NONE', #23253, #1678, #7424 ) ;
#23756=CIRCLE ( 'NONE', #20000, 30.10000000000000142 ) ;
#23760=DIRECTION ( 'NONE',  ( -0.2486898871648449971, 0.9685831611286336296, 0.000000000000000000 ) ) ;
#23762=DIRECTION ( 'NONE',  ( -0.000000000000000000, 0.000000000000000000, 1.000000000000000000 ) ) ;
#23766=DIRECTION ( 'NONE',  ( 0.000000000000000000, 0.000000000000000000, 1.000000000000000000 ) ) ;
#23767=ORIENTED_EDGE ( 'NONE', *, *, #9443, .T. ) ;
#23768=DIRECTION ( 'NONE',  ( 1.000000000000000000, 0.000000000000000000, 0.000000000000000000 ) ) ;
#23771=DIRECTION ( 'NONE',  ( -0.000000000000000000, -0.000000000000000000, 1.000000000000000000 ) ) ;
#23773=CARTESIAN_POINT ( 'NONE',  ( -21.65113613650350288, -22.32573188046905344, 1.000000000000000000 ) ) ;
#23774=DIRECTION ( 'NONE',  ( -0.000000000000000000, -0.000000000000000000, 1.000000000000000000 ) ) ;
#23780=CIRCLE ( 'NONE', #7101, 0.5000000000000011102 ) ;
#23781=VERTEX_POINT ( 'NONE', #4800 ) ;
#23782=AXIS2_PLACEMENT_3D ( 'NONE', #3995, #19933, #22700 ) ;
#23784=EDGE_LOOP ( 'NONE', ( #10175, #6451, #11261, #13747 ) ) ;
#23785=ORIENTED_EDGE ( 'NONE', *, *, #2510, .F. ) ;
#23786=CARTESIAN_POINT ( 'NONE',  ( 2.451530025008918923, -31.00322564728515928, 1.000000000000000000 ) ) ;
#23787=CARTESIAN_POINT ( 'NONE',  ( 28.72825533807133169, 11.91206721063041485, -2.750000000000000000 ) ) ;
#23792=AXIS2_PLACEMENT_3D ( 'NONE', #22737, #22989, #18671 ) ;
#23796=VECTOR ( 'NONE', #4741, 1000.000000000000000 ) ;
#23798=CARTESIAN_POINT ( 'NONE',  ( -30.35476721088022600, 3.897863563850190616, -6.500000000000000000 ) ) ;
#23799=CARTESIAN_POINT ( 'NONE',  ( -19.82388608118446527, -23.96296185032687376, -6.500000000000000000 ) ) ;
#23800=CIRCLE ( 'NONE', #1195, 0.5000000000000001110 ) ;
#23802=CARTESIAN_POINT ( 'NONE',  ( 31.09598070739550479, 0.4999838450258677902, -6.500000000000000000 ) ) ;
#23821=ORIENTED_EDGE ( 'NONE', *, *, #24350, .T. ) ;
#23822=FACE_OUTER_BOUND ( 'NONE', #25363, .T. ) ;
#23830=CIRCLE ( 'NONE', #14659, 0.4999999999999986122 ) ;
#23831=CYLINDRICAL_SURFACE ( 'NONE', #13809, 31.10000000000000142 ) ;
#23832=EDGE_CURVE ( 'NONE', #4688, #22740, #8856, .T. ) ;
#23833=CYLINDRICAL_SURFACE ( 'NONE', #9612, 0.5000000000000004441 ) ;
#23835=AXIS2_PLACEMENT_3D ( 'NONE', #14347, #8069, #18147 ) ;
#23838=ADVANCED_FACE ( 'NONE', ( #624 ), #2439, .T. ) ;
#23840=CARTESIAN_POINT ( 'NONE',  ( -28.91604871112448549, 11.44867358849382910, -6.500000000000000000 ) ) ;
#23843=EDGE_CURVE ( 'NONE', #21381, #24200, #24530, .T. ) ;
#23845=CIRCLE ( 'NONE', #9664, 31.10000000000000142 ) ;
#23850=DIRECTION ( 'NONE',  ( 0.000000000000000000, 0.000000000000000000, 1.000000000000000000 ) ) ;
#23852=ORIENTED_EDGE ( 'NONE', *, *, #4493, .F. ) ;
#23854=VECTOR ( 'NONE', #11573, 1000.000000000000000 ) ;
#23857=EDGE_LOOP ( 'NONE', ( #554, #7635, #18084, #23597 ) ) ;
#23859=DIRECTION ( 'NONE',  ( -0.000000000000000000, 0.000000000000000000, -1.000000000000000000 ) ) ;
#23861=VECTOR ( 'NONE', #3340, 1000.000000000000000 ) ;
#23863=CYLINDRICAL_SURFACE ( 'NONE', #12499, 0.5000000000000004441 ) ;
#23865=CIRCLE ( 'NONE', #9682, 0.4999999999999991118 ) ;
#23867=AXIS2_PLACEMENT_3D ( 'NONE', #2214, #16192, #7959 ) ;
#23868=CIRCLE ( 'NONE', #922, 31.10000000000000142 ) ;
#23870=CARTESIAN_POINT ( 'NONE',  ( -26.75313774936430633, -14.98253926456308172, -6.500000000000000000 ) ) ;
#23872=AXIS2_PLACEMENT_3D ( 'NONE', #14026, #4337, #4069 ) ;
#23875=CARTESIAN_POINT ( 'NONE',  ( 31.09598070739550479, 0.4999838450258677902, 1.000000000000000000 ) ) ;
#23877=CARTESIAN_POINT ( 'NONE',  ( -30.53863125411922752, 1.952785157361987878, -6.500000000000000000 ) ) ;
#23879=ORIENTED_EDGE ( 'NONE', *, *, #22102, .T. ) ;
#23886=ADVANCED_FACE ( 'NONE', ( #21259 ), #7147, .T. ) ;
#23887=DIRECTION ( 'NONE',  ( 1.000000000000000000, 0.000000000000000000, -0.000000000000000000 ) ) ;
#23888=AXIS2_PLACEMENT_3D ( 'NONE', #16410, #24378, #23887 ) ;
#23890=DIRECTION ( 'NONE',  ( 1.387778780781445044E-14, 1.000000000000000000, 0.000000000000000000 ) ) ;
#23894=AXIS2_PLACEMENT_3D ( 'NONE', #20910, #6523, #24704 ) ;
#23897=AXIS2_PLACEMENT_3D ( 'NONE', #4167, #648, #16596 ) ;
#23898=AXIS2_PLACEMENT_3D ( 'NONE', #17979, #22288, #4488 ) ;
#23899=CYLINDRICAL_SURFACE ( 'NONE', #18779, 0.5000000000000004441 ) ;
#23904=DIRECTION ( 'NONE',  ( -0.000000000000000000, -0.000000000000000000, 1.000000000000000000 ) ) ;
#23905=DIRECTION ( 'NONE',  ( 0.000000000000000000, 0.000000000000000000, 1.000000000000000000 ) ) ;
#23916=FACE_OUTER_BOUND ( 'NONE', #4328, .T. ) ;
#23919=DIRECTION ( 'NONE',  ( 0.000000000000000000, 0.000000000000000000, 1.000000000000000000 ) ) ;
#23922=ORIENTED_EDGE ( 'NONE', *, *, #17341, .T. ) ;
#23923=VERTEX_POINT ( 'NONE', #15516 ) ;
#23924=VERTEX_POINT ( 'NONE', #19162 ) ;
#23925=CARTESIAN_POINT ( 'NONE',  ( -9.110428525061097460, -29.57785765677920509, -6.500000000000000000 ) ) ;
#23926=DIRECTION ( 'NONE',  ( 1.000000000000000000, 0.000000000000000000, 0.000000000000000000 ) ) ;
#23934=DIRECTION ( 'NONE',  ( 1.000000000000000000, 0.000000000000000000, 0.000000000000000000 ) ) ;
#23936=CIRCLE ( 'NONE', #12670, 0.5000000000000002220 ) ;
#23939=DIRECTION ( 'NONE',  ( 1.000000000000000000, 0.000000000000000000, 0.000000000000000000 ) ) ;
#23940=FACE_OUTER_BOUND ( 'NONE', #20829, .T. ) ;
#23943=CYLINDRICAL_SURFACE ( 'NONE', #16633, 0.5000000000000004441 ) ;
#23945=CARTESIAN_POINT ( 'NONE',  ( 0.000000000000000000, 0.000000000000000000, -6.500000000000000000 ) ) ;
#23947=ORIENTED_EDGE ( 'NONE', *, *, #5268, .F. ) ;
#23951=ADVANCED_FACE ( 'NONE', ( #19297 ), #13551, .F. ) ;
#23952=EDGE_CURVE ( 'NONE', #9729, #24341, #1121, .T. ) ;
#23955=ORIENTED_EDGE ( 'NONE', *, *, #23372, .F. ) ;
#23956=ORIENTED_EDGE ( 'NONE', *, *, #13095, .T. ) ;
#23960=EDGE_LOOP ( 'NONE', ( #15629, #1592, #20507, #22796 ) ) ;
#23963=ADVANCED_FACE ( 'NONE', ( #9239 ), #7006, .T. ) ;
#23976=ORIENTED_EDGE ( 'NONE', *, *, #23130, .F. ) ;
#23979=ORIENTED_EDGE ( 'NONE', *, *, #16566, .F. ) ;
#23985=VERTEX_POINT ( 'NONE', #25435 ) ;
#23986=CARTESIAN_POINT ( 'NONE',  ( 0.000000000000000000, 0.000000000000000000, -6.500000000000000000 ) ) ;
#23989=EDGE_CURVE ( 'NONE', #10388, #4038, #21576, .T. ) ;
#23990=CARTESIAN_POINT ( 'NONE',  ( 6.317933499823220167, -30.45149776762731975, -6.500000000000000000 ) ) ;
#23999=LINE ( 'NONE', #6078, #9726 ) ;
#24002=CARTESIAN_POINT ( 'NONE',  ( 24.86329371854774806, 18.68225429291723216, -2.750000000000000000 ) ) ;
#24004=ORIENTED_EDGE ( 'NONE', *, *, #1479, .T. ) ;
#24006=EDGE_CURVE ( 'NONE', #17747, #14371, #18024, .T. ) ;
#24009=EDGE_LOOP ( 'NONE', ( #20272, #11018, #11819, #2656 ) ) ;
#24011=CARTESIAN_POINT ( 'NONE',  ( -7.734255490827218971, -30.12293631110037140, -6.500000000000000000 ) ) ;
#24013=ORIENTED_EDGE ( 'NONE', *, *, #8865, .F. ) ;
#24014=ORIENTED_EDGE ( 'NONE', *, *, #460, .F. ) ;
#24017=DIRECTION ( 'NONE',  ( 0.000000000000000000, 0.000000000000000000, 1.000000000000000000 ) ) ;
#24020=EDGE_CURVE ( 'NONE', #23923, #22016, #5059, .T. ) ;
#24022=DIRECTION ( 'NONE',  ( 1.000000000000000000, 0.000000000000000000, 0.000000000000000000 ) ) ;
#24023=ADVANCED_FACE ( 'NONE', ( #23485 ), #17350, .F. ) ;
#24027=CARTESIAN_POINT ( 'NONE',  ( 7.248980000274197977, 30.24338421796781518, -2.750000000000000000 ) ) ;
#24028=LINE ( 'NONE', #23520, #21649 ) ;
#24036=DIRECTION ( 'NONE',  ( 0.9297764858882504591, -0.3681245526846803617, 0.000000000000000000 ) ) ;
#24037=AXIS2_PLACEMENT_3D ( 'NONE', #1239, #17973, #4233 ) ;
#24038=ORIENTED_EDGE ( 'NONE', *, *, #12740, .T. ) ;
#24041=DIRECTION ( 'NONE',  ( 0.000000000000000000, 0.000000000000000000, 1.000000000000000000 ) ) ;
#24043=ORIENTED_EDGE ( 'NONE', *, *, #16100, .F. ) ;
#24044=ORIENTED_EDGE ( 'NONE', *, *, #19807, .T. ) ;
#24045=VERTEX_POINT ( 'NONE', #23105 ) ;
#24046=EDGE_LOOP ( 'NONE', ( #4785, #21061, #15050, #4230 ) ) ;
#24047=CARTESIAN_POINT ( 'NONE',  ( 30.12293631110045311, 7.734255490826897450, 1.000000000000000000 ) ) ;
#24050=AXIS2_PLACEMENT_3D ( 'NONE', #19476, #17523, #23926 ) ;
#24053=ADVANCED_FACE ( 'NONE', ( #13426 ), #14992, .F. ) ;
#24055=EDGE_CURVE ( 'NONE', #7738, #6126, #20941, .T. ) ;
#24056=CARTESIAN_POINT ( 'NONE',  ( -28.14012133169333651, -13.24173596767349359, -6.500000000000000000 ) ) ;
#24057=DIRECTION ( 'NONE',  ( -0.000000000000000000, 0.000000000000000000, 1.000000000000000000 ) ) ;
#24067=DIRECTION ( 'NONE',  ( 0.000000000000000000, -0.000000000000000000, 1.000000000000000000 ) ) ;
#24072=EDGE_LOOP ( 'NONE', ( #22767, #18281, #15218, #17284 ) ) ;
#24074=ORIENTED_EDGE ( 'NONE', *, *, #1842, .T. ) ;
#24075=EDGE_LOOP ( 'NONE', ( #23979, #4485, #17036, #818 ) ) ;
#24077=CARTESIAN_POINT ( 'NONE',  ( -21.28941499438192864, 22.67092431280617859, 1.000000000000000000 ) ) ;
#24081=ADVANCED_FACE ( 'NONE', ( #16153 ), #1908, .T. ) ;
#24083=DIRECTION ( 'NONE',  ( 0.000000000000000000, 0.000000000000000000, 1.000000000000000000 ) ) ;
#24087=CARTESIAN_POINT ( 'NONE',  ( -18.28012134629613783, -25.16042852506070560, -6.500000000000000000 ) ) ;
#24093=CARTESIAN_POINT ( 'NONE',  ( 0.000000000000000000, 0.000000000000000000, -6.500000000000000000 ) ) ;
#24094=ORIENTED_EDGE ( 'NONE', *, *, #11594, .F. ) ;
#24095=EDGE_LOOP ( 'NONE', ( #14211, #23498, #1501, #4821 ) ) ;
#24098=ORIENTED_EDGE ( 'NONE', *, *, #18524, .T. ) ;
#24099=DIRECTION ( 'NONE',  ( 0.000000000000000000, 0.000000000000000000, 1.000000000000000000 ) ) ;
#24104=CARTESIAN_POINT ( 'NONE',  ( 0.000000000000000000, 0.000000000000000000, -6.500000000000000000 ) ) ;
#24117=DIRECTION ( 'NONE',  ( -0.000000000000000000, -0.000000000000000000, 1.000000000000000000 ) ) ;
#24124=ORIENTED_EDGE ( 'NONE', *, *, #18638, .F. ) ;
#24128=ORIENTED_EDGE ( 'NONE', *, *, #12866, .T. ) ;
#24131=DIRECTION ( 'NONE',  ( -0.000000000000000000, -0.000000000000000000, 1.000000000000000000 ) ) ;
#24132=CIRCLE ( 'NONE', #1179, 0.5000000000000004441 ) ;
#24137=CYLINDRICAL_SURFACE ( 'NONE', #13879, 0.5000000000000004441 ) ;
#24140=DIRECTION ( 'NONE',  ( 0.1253332335642980688, -0.9921147013144785420, 0.000000000000000000 ) ) ;
#24143=EDGE_CURVE ( 'NONE', #9505, #19523, #14685, .T. ) ;
#24144=DIRECTION ( 'NONE',  ( 1.000000000000000000, 0.000000000000000000, 0.000000000000000000 ) ) ;
#24150=ORIENTED_EDGE ( 'NONE', *, *, #25224, .F. ) ;
#24151=CYLINDRICAL_SURFACE ( 'NONE', #7200, 31.10000000000000142 ) ;
#24156=EDGE_CURVE ( 'NONE', #10563, #11374, #21366, .T. ) ;
#24157=CARTESIAN_POINT ( 'NONE',  ( -28.72825533807142051, -11.91206721063020701, 1.000000000000000000 ) ) ;
#24164=ORIENTED_EDGE ( 'NONE', *, *, #19318, .F. ) ;
#24167=ORIENTED_EDGE ( 'NONE', *, *, #25293, .F. ) ;
#24168=VERTEX_POINT ( 'NONE', #13668 ) ;
#24172=DIRECTION ( 'NONE',  ( 0.000000000000000000, 0.000000000000000000, 1.000000000000000000 ) ) ;
#24174=VECTOR ( 'NONE', #12918, 1000.000000000000000 ) ;
#24183=VECTOR ( 'NONE', #21232, 1000.000000000000000 ) ;
#24184=DIRECTION ( 'NONE',  ( 0.000000000000000000, -0.000000000000000000, 1.000000000000000000 ) ) ;
#24186=CARTESIAN_POINT ( 'NONE',  ( -27.49048467073869517, -14.54246377227329212, -6.500000000000000000 ) ) ;
#24187=DIRECTION ( 'NONE',  ( -0.1253332335643051187, -0.9921147013144777649, 0.000000000000000000 ) ) ;
#24190=CARTESIAN_POINT ( 'NONE',  ( -23.01025686871661335, -20.92219106202025714, -6.500000000000000000 ) ) ;
#24192=ADVANCED_FACE ( 'NONE', ( #25824 ), #3719, .T. ) ;
#24193=AXIS2_PLACEMENT_3D ( 'NONE', #19082, #25352, #9409 ) ;
#24194=CARTESIAN_POINT ( 'NONE',  ( -9.610428525060479288, 29.57785765677940404, -6.500000000000000000 ) ) ;
#24195=CARTESIAN_POINT ( 'NONE',  ( 0.000000000000000000, 0.000000000000000000, -6.500000000000000000 ) ) ;
#24200=VERTEX_POINT ( 'NONE', #13938 ) ;
#24202=EDGE_CURVE ( 'NONE', #5409, #7760, #24726, .T. ) ;
#24204=EDGE_LOOP ( 'NONE', ( #13650, #13598, #5117, #16052 ) ) ;
#24205=CYLINDRICAL_SURFACE ( 'NONE', #9705, 31.10000000000000142 ) ;
#24207=EDGE_CURVE ( 'NONE', #17608, #14723, #22221, .T. ) ;
#24208=AXIS2_PLACEMENT_3D ( 'NONE', #13336, #1167, #10845 ) ;
#24209=ORIENTED_EDGE ( 'NONE', *, *, #21854, .F. ) ;
#24210=DIRECTION ( 'NONE',  ( 0.1873813145857189666, -0.9822872507286897203, 0.000000000000000000 ) ) ;
#24213=VECTOR ( 'NONE', #19140, 1000.000000000000000 ) ;
#24218=DIRECTION ( 'NONE',  ( 0.7705132427757999114, 0.6374239897486768669, 0.000000000000000000 ) ) ;
#24219=VECTOR ( 'NONE', #23654, 1000.000000000000000 ) ;
#24223=AXIS2_PLACEMENT_3D ( 'NONE', #24604, #14680, #4749 ) ;
#24232=EDGE_LOOP ( 'NONE', ( #11621, #480, #11856, #24381 ) ) ;
#24236=DIRECTION ( 'NONE',  ( 0.000000000000000000, 0.000000000000000000, 1.000000000000000000 ) ) ;
#24237=VERTEX_POINT ( 'NONE', #18368 ) ;
#24239=DIRECTION ( 'NONE',  ( 0.000000000000000000, 0.000000000000000000, 1.000000000000000000 ) ) ;
#24243=CARTESIAN_POINT ( 'NONE',  ( -5.827558883616271501, -30.54913349766217934, -6.500000000000000000 ) ) ;
#24244=AXIS2_PLACEMENT_3D ( 'NONE', #23519, #11483, #9656 ) ;
#24246=CARTESIAN_POINT ( 'NONE',  ( -27.64012133169333651, -13.24173596767349359, 1.000000000000000000 ) ) ;
#24249=AXIS2_PLACEMENT_3D ( 'NONE', #7810, #25855, #15790 ) ;
#24251=CYLINDRICAL_SURFACE ( 'NONE', #11346, 0.5000000000000004441 ) ;
#24260=ORIENTED_EDGE ( 'NONE', *, *, #14610, .F. ) ;
#24264=VERTEX_POINT ( 'NONE', #2678 ) ;
#24265=EDGE_CURVE ( 'NONE', #7323, #17107, #4890, .T. ) ;
#24267=CARTESIAN_POINT ( 'NONE',  ( -14.48253926456356666, -27.25313774936403988, -6.500000000000000000 ) ) ;
#24268=AXIS2_PLACEMENT_3D ( 'NONE', #873, #20343, #498 ) ;
#24271=ORIENTED_EDGE ( 'NONE', *, *, #21368, .T. ) ;
#24272=ORIENTED_EDGE ( 'NONE', *, *, #11052, .F. ) ;
#24277=ADVANCED_FACE ( 'NONE', ( #16424 ), #24251, .F. ) ;
#24279=DIRECTION ( 'NONE',  ( 0.000000000000000000, 0.000000000000000000, 1.000000000000000000 ) ) ;
#24281=VECTOR ( 'NONE', #23251, 1000.000000000000000 ) ;
#24292=CARTESIAN_POINT ( 'NONE',  ( -27.92360179968386547, -13.69242354489123770, -6.500000000000000000 ) ) ;
#24296=EDGE_LOOP ( 'NONE', ( #1145, #17303, #157, #11112 ) ) ;
#24299=EDGE_LOOP ( 'NONE', ( #23683, #4193, #9887, #21725 ) ) ;
#24303=FACE_OUTER_BOUND ( 'NONE', #18291, .T. ) ;
#24305=CIRCLE ( 'NONE', #13868, 31.10000000000000142 ) ;
#24306=AXIS2_PLACEMENT_3D ( 'NONE', #12721, #16779, #299 ) ;
#24313=EDGE_CURVE ( 'NONE', #1345, #7996, #10093, .T. ) ;
#24316=CIRCLE ( 'NONE', #13889, 0.4999999999999997224 ) ;
#24322=AXIS2_PLACEMENT_3D ( 'NONE', #22093, #538, #8511 ) ;
#24323=DIRECTION ( 'NONE',  ( 0.000000000000000000, 0.000000000000000000, 1.000000000000000000 ) ) ;
#24324=FACE_OUTER_BOUND ( 'NONE', #1080, .T. ) ;
#24331=CARTESIAN_POINT ( 'NONE',  ( -22.67092431280563503, 21.28941499438250062, -6.500000000000000000 ) ) ;
#24333=CYLINDRICAL_SURFACE ( 'NONE', #1642, 31.10000000000000142 ) ;
#24334=LINE ( 'NONE', #8634, #15576 ) ;
#24335=ORIENTED_EDGE ( 'NONE', *, *, #2728, .T. ) ;
#24336=DIRECTION ( 'NONE',  ( 1.000000000000000000, 0.000000000000000000, 0.000000000000000000 ) ) ;
#24337=CARTESIAN_POINT ( 'NONE',  ( 16.23990935651717393, 26.52310962334745170, -6.500000000000000000 ) ) ;
#24338=ORIENTED_EDGE ( 'NONE', *, *, #16167, .F. ) ;
#24339=AXIS2_PLACEMENT_3D ( 'NONE', #24047, #8227, #134 ) ;
#24340=ORIENTED_EDGE ( 'NONE', *, *, #13667, .F. ) ;
#24341=VERTEX_POINT ( 'NONE', #24391 ) ;
#24342=ORIENTED_EDGE ( 'NONE', *, *, #10353, .F. ) ;
#24346=DIRECTION ( 'NONE',  ( -0.7289686274214034478, 0.6845471059286972748, 0.000000000000000000 ) ) ;
#24347=ORIENTED_EDGE ( 'NONE', *, *, #9292, .F. ) ;
#24350=EDGE_CURVE ( 'NONE', #18321, #9729, #20121, .T. ) ;
#24357=CYLINDRICAL_SURFACE ( 'NONE', #18841, 0.5000000000000004441 ) ;
#24363=CARTESIAN_POINT ( 'NONE',  ( 25.45105997952917676, 17.87326343783944083, 1.000000000000000000 ) ) ;
#24365=EDGE_CURVE ( 'NONE', #2838, #16618, #21613, .T. ) ;
#24369=VERTEX_POINT ( 'NONE', #49 ) ;
#24375=VERTEX_POINT ( 'NONE', #11930 ) ;
#24377=ORIENTED_EDGE ( 'NONE', *, *, #21628, .F. ) ;
#24378=DIRECTION ( 'NONE',  ( 0.000000000000000000, 0.000000000000000000, 1.000000000000000000 ) ) ;
#24379=VECTOR ( 'NONE', #23509, 1000.000000000000000 ) ;
#24380=DIRECTION ( 'NONE',  ( 0.000000000000000000, 0.000000000000000000, 1.000000000000000000 ) ) ;
#24381=ORIENTED_EDGE ( 'NONE', *, *, #24207, .T. ) ;
#24386=DIRECTION ( 'NONE',  ( -0.000000000000000000, -0.000000000000000000, 1.000000000000000000 ) ) ;
#24391=CARTESIAN_POINT ( 'NONE',  ( -1.453535542772161238, 31.06601413805604750, -6.500000000000000000 ) ) ;
#24394=ADVANCED_FACE ( 'NONE', ( #20921 ), #12941, .F. ) ;
#24398=ORIENTED_EDGE ( 'NONE', *, *, #6565, .T. ) ;
#24402=VERTEX_POINT ( 'NONE', #14428 ) ;
#24406=DIRECTION ( 'NONE',  ( 0.7705132427757873659, -0.6374239897486919659, 0.000000000000000000 ) ) ;
#24409=EDGE_LOOP ( 'NONE', ( #7252, #21109, #20860, #16331, #281, #550, #2272, #10629, #19854, #183, #9733, #21094, #9667, #5080, #9296, #22642, #21446, #4548, #15356, #2777, #11498, #16644, #4695, #23205, #4851, #2341, #610, #12456, #11828, #4846, #17383, #11973, #21442, #23156, #25678, #14344, #8915, #24618, #9210, #14794, #13790, #3700, #21828, #7881, #2526, #4084, #8881, #14286, #15277, #886, #24585, #23088, #14095, #10415, #575, #16559, #22993, #15498, #15606, #10686, #2843, #7232, #6634, #24948, #2911, #22675, #14879, #24487, #18290, #12984, #10045, #24883, #17937, #22405, #6125, #10296, #18422, #16012, #8226, #6157, #12989, #1212, #7800, #21001, #11650, #3166, #14024, #24098, #20274, #14437, #4427, #2558, #25393, #11024, #4056, #3670, #13443, #7669, #4156, #18381, #22043, #22141, #2633, #98, #9318, #7642, #15015, #260, #22248, #9418, #2179, #12166, #10199, #10764, #21654, #8135, #3873, #18081, #15181, #19764, #416, #3673, #11106, #17748, #23956, #9800, #2951, #11547, #3223, #8693, #25777, #24150, #2881, #730, #22643, #21498, #15392, #606, #1921, #7891, #6453, #17015, #257, #411, #9463, #24984, #14290, #24074, #23659, #25561, #18907, #5042, #18456, #17717, #11911, #24340, #21479, #9629, #6731, #14924, #8193, #19411, #12242, #18259, #17173, #13756, #9641, #2247, #10208, #25389, #24124, #5457, #24695, #7202, #6056, #3640, #24014, #23767, #16340, #22890, #25800, #19597, #20568, #10532, #13217, #23785, #19091, #21313, #5232, #726, #2669, #23323, #10105, #12759, #23401, #7573, #313, #24377, #2712, #19527, #8520, #14140, #6781, #1760, #14051, #11549, #14658, #7324, #5289, #4363, #14727, #21377, #14699, #8908, #12107, #13986, #19207, #25347, #4305, #11155, #14408, #19217, #15553, #18120, #11815, #3019, #6575, #8639, #7235, #507, #10715, #23457, #22600, #17011, #9973, #18945, #10566, #25744, #14490, #18739, #7890, #1868, #5081, #23748, #1107, #14013, #18228, #11471, #18996 ) ) ;
#24412=CARTESIAN_POINT ( 'NONE',  ( -9.610428525061097460, -29.57785765677920509, -6.500000000000000000 ) ) ;
#24413=DIRECTION ( 'NONE',  ( 1.000000000000000000, 0.000000000000000000, 0.000000000000000000 ) ) ;
#24415=EDGE_CURVE ( 'NONE', #20933, #15851, #12608, .T. ) ;
#24417=DIRECTION ( 'NONE',  ( 0.000000000000000000, 0.000000000000000000, 1.000000000000000000 ) ) ;
#24421=DIRECTION ( 'NONE',  ( 0.000000000000000000, -0.000000000000000000, 1.000000000000000000 ) ) ;
#24422=DIRECTION ( 'NONE',  ( 0.000000000000000000, 0.000000000000000000, 1.000000000000000000 ) ) ;
#24424=DIRECTION ( 'NONE',  ( 1.000000000000000000, 0.000000000000000000, 0.000000000000000000 ) ) ;
#24426=LINE ( 'NONE', #16465, #15836 ) ;
#24430=DIRECTION ( 'NONE',  ( -0.000000000000000000, -0.000000000000000000, 1.000000000000000000 ) ) ;
#24432=CYLINDRICAL_SURFACE ( 'NONE', #15850, 31.10000000000000142 ) ;
#24433=VERTEX_POINT ( 'NONE', #16255 ) ;
#24434=CARTESIAN_POINT ( 'NONE',  ( -27.00874656207317059, -15.41874213889385459, 1.000000000000000000 ) ) ;
#24436=EDGE_CURVE ( 'NONE', #12308, #5761, #86, .T. ) ;
#24441=LINE ( 'NONE', #10430, #3043 ) ;
#24448=DIRECTION ( 'NONE',  ( -0.000000000000000000, -0.000000000000000000, 1.000000000000000000 ) ) ;
#24455=DIRECTION ( 'NONE',  ( 1.000000000000000000, 0.000000000000000000, 0.000000000000000000 ) ) ;
#24456=DIRECTION ( 'NONE',  ( 0.000000000000000000, 0.000000000000000000, 1.000000000000000000 ) ) ;
#24457=CARTESIAN_POINT ( 'NONE',  ( 0.000000000000000000, 0.000000000000000000, -6.500000000000000000 ) ) ;
#24459=EDGE_CURVE ( 'NONE', #24369, #14282, #19282, .T. ) ;
#24460=ORIENTED_EDGE ( 'NONE', *, *, #853, .F. ) ;
#24463=DIRECTION ( 'NONE',  ( 0.000000000000000000, -0.000000000000000000, 1.000000000000000000 ) ) ;
#24464=ORIENTED_EDGE ( 'NONE', *, *, #25125, .T. ) ;
#24465=VERTEX_POINT ( 'NONE', #2388 ) ;
#24467=ORIENTED_EDGE ( 'NONE', *, *, #1570, .T. ) ;
#24473=CARTESIAN_POINT ( 'NONE',  ( -13.24173596767339767, 28.14012133169338270, 1.000000000000000000 ) ) ;
#24474=DIRECTION ( 'NONE',  ( 1.000000000000000000, 0.000000000000000000, 0.000000000000000000 ) ) ;
#24478=CARTESIAN_POINT ( 'NONE',  ( 0.000000000000000000, 0.000000000000000000, -6.500000000000000000 ) ) ;
#24479=FACE_OUTER_BOUND ( 'NONE', #21235, .T. ) ;
#24486=VERTEX_POINT ( 'NONE', #18343 ) ;
#24487=ORIENTED_EDGE ( 'NONE', *, *, #24156, .T. ) ;
#24490=VERTEX_POINT ( 'NONE', #3005 ) ;
#24491=DIRECTION ( 'NONE',  ( 0.000000000000000000, 0.000000000000000000, 1.000000000000000000 ) ) ;
#24492=ORIENTED_EDGE ( 'NONE', *, *, #2302, .F. ) ;
#24496=DIRECTION ( 'NONE',  ( 0.06279051952932236669, 0.9980267284282710039, 0.000000000000000000 ) ) ;
#24497=DIRECTION ( 'NONE',  ( -0.6845471059286901694, -0.7289686274214101092, 0.000000000000000000 ) ) ;
#24500=DIRECTION ( 'NONE',  ( 0.3090169943749591086, 0.9510565162951497564, 0.000000000000000000 ) ) ;
#24510=DIRECTION ( 'NONE',  ( 1.000000000000000000, 0.000000000000000000, 0.000000000000000000 ) ) ;
#24518=ORIENTED_EDGE ( 'NONE', *, *, #8746, .F. ) ;
#24519=CARTESIAN_POINT ( 'NONE',  ( 0.000000000000000000, 0.000000000000000000, 0.000000000000000000 ) ) ;
#24522=EDGE_CURVE ( 'NONE', #16527, #15624, #18221, .T. ) ;
#24525=DIRECTION ( 'NONE',  ( 1.000000000000000000, 0.000000000000000000, 0.000000000000000000 ) ) ;
#24526=EDGE_CURVE ( 'NONE', #1309, #5799, #8855, .T. ) ;
#24530=LINE ( 'NONE', #18399, #23450 ) ;
#24533=LINE ( 'NONE', #10796, #8707 ) ;
#24537=DIRECTION ( 'NONE',  ( -0.000000000000000000, 0.000000000000000000, 1.000000000000000000 ) ) ;
#24539=DIRECTION ( 'NONE',  ( -0.6374239897486919659, -0.7705132427757873659, 0.000000000000000000 ) ) ;
#24543=VERTEX_POINT ( 'NONE', #9017 ) ;
#24544=CARTESIAN_POINT ( 'NONE',  ( -6.317933499822993682, 30.45149776762736593, 1.000000000000000000 ) ) ;
#24547=CARTESIAN_POINT ( 'NONE',  ( 0.000000000000000000, 0.000000000000000000, -6.500000000000000000 ) ) ;
#24551=EDGE_CURVE ( 'NONE', #12308, #23924, #15543, .T. ) ;
#24554=ORIENTED_EDGE ( 'NONE', *, *, #23753, .F. ) ;
#24558=CARTESIAN_POINT ( 'NONE',  ( -1.952785157361201618, 31.03863125411927371, -6.500000000000000000 ) ) ;
#24561=CARTESIAN_POINT ( 'NONE',  ( -10.94867358849309547, 28.91604871112477326, 1.000000000000000000 ) ) ;
#24563=EDGE_CURVE ( 'NONE', #24543, #10325, #22641, .T. ) ;
#24564=CARTESIAN_POINT ( 'NONE',  ( -30.78811501957140706, 4.393401135981310546, 1.000000000000000000 ) ) ;
#24565=CARTESIAN_POINT ( 'NONE',  ( 0.000000000000000000, 0.000000000000000000, 1.000000000000000000 ) ) ;
#24568=CARTESIAN_POINT ( 'NONE',  ( 3.897863563849872204, 30.85476721088026508, -6.500000000000000000 ) ) ;
#24569=DIRECTION ( 'NONE',  ( 0.000000000000000000, 0.000000000000000000, 1.000000000000000000 ) ) ;
#24572=DIRECTION ( 'NONE',  ( 0.000000000000000000, -0.000000000000000000, 1.000000000000000000 ) ) ;
#24573=VECTOR ( 'NONE', #13205, 1000.000000000000000 ) ;
#24574=CARTESIAN_POINT ( 'NONE',  ( -18.28012134629613783, -25.16042852506070560, -6.500000000000000000 ) ) ;
#24576=AXIS2_PLACEMENT_3D ( 'NONE', #4285, #18402, #20098 ) ;
#24577=ORIENTED_EDGE ( 'NONE', *, *, #14336, .F. ) ;
#24578=CARTESIAN_POINT ( 'NONE',  ( 0.000000000000000000, 0.000000000000000000, -6.500000000000000000 ) ) ;
#24580=VERTEX_POINT ( 'NONE', #21301 ) ;
#24582=ORIENTED_EDGE ( 'NONE', *, *, #23192, .T. ) ;
#24583=VECTOR ( 'NONE', #4249, 1000.000000000000000 ) ;
#24585=ORIENTED_EDGE ( 'NONE', *, *, #5772, .F. ) ;
#24588=DIRECTION ( 'NONE',  ( 0.000000000000000000, 0.000000000000000000, 1.000000000000000000 ) ) ;
#24589=ORIENTED_EDGE ( 'NONE', *, *, #16990, .T. ) ;
#24590=DIRECTION ( 'NONE',  ( 0.000000000000000000, 0.000000000000000000, 1.000000000000000000 ) ) ;
#24593=VECTOR ( 'NONE', #788, 1000.000000000000000 ) ;
#24595=CIRCLE ( 'NONE', #19993, 0.5000000000000002220 ) ;
#24597=FACE_OUTER_BOUND ( 'NONE', #4580, .T. ) ;
#24598=DIRECTION ( 'NONE',  ( 0.000000000000000000, 0.000000000000000000, 1.000000000000000000 ) ) ;
#24599=VECTOR ( 'NONE', #2420, 1000.000000000000000 ) ;
#24601=CYLINDRICAL_SURFACE ( 'NONE', #10037, 0.5000000000000004441 ) ;
#24602=AXIS2_PLACEMENT_3D ( 'NONE', #24574, #12816, #12552 ) ;
#24604=CARTESIAN_POINT ( 'NONE',  ( -29.57785765677936851, -9.610428525060582317, -6.500000000000000000 ) ) ;
#24605=CARTESIAN_POINT ( 'NONE',  ( -18.28012134629558716, 25.16042852506110705, -6.500000000000000000 ) ) ;
#24606=DIRECTION ( 'NONE',  ( -0.000000000000000000, -0.000000000000000000, 1.000000000000000000 ) ) ;
#24607=DIRECTION ( 'NONE',  ( 1.000000000000000000, 0.000000000000000000, 0.000000000000000000 ) ) ;
#24614=VECTOR ( 'NONE', #8466, 1000.000000000000000 ) ;
#24618=ORIENTED_EDGE ( 'NONE', *, *, #20649, .T. ) ;
#24619=CARTESIAN_POINT ( 'NONE',  ( 0.000000000000000000, 0.000000000000000000, -6.500000000000000000 ) ) ;
#24621=AXIS2_PLACEMENT_3D ( 'NONE', #7501, #14045, #1889 ) ;
#24622=EDGE_LOOP ( 'NONE', ( #3845, #24759, #6962, #18995 ) ) ;
#24623=DIRECTION ( 'NONE',  ( 1.000000000000000000, 0.000000000000000000, 0.000000000000000000 ) ) ;
#24628=FACE_OUTER_BOUND ( 'NONE', #4164, .T. ) ;
#24631=EDGE_CURVE ( 'NONE', #3398, #4306, #931, .T. ) ;
#24642=CIRCLE ( 'NONE', #14199, 0.5000000000000003331 ) ;
#24646=CARTESIAN_POINT ( 'NONE',  ( -16.66421332384646448, 26.25859848311288403, 1.000000000000000000 ) ) ;
#24648=ORIENTED_EDGE ( 'NONE', *, *, #8373, .T. ) ;
#24655=EDGE_CURVE ( 'NONE', #15624, #21567, #3827, .T. ) ;
#24660=AXIS2_PLACEMENT_3D ( 'NONE', #3961, #12319, #12440 ) ;
#24679=AXIS2_PLACEMENT_3D ( 'NONE', #18156, #9778, #233 ) ;
#24682=ORIENTED_EDGE ( 'NONE', *, *, #7481, .T. ) ;
#24684=CARTESIAN_POINT ( 'NONE',  ( -26.25859848311282363, -16.66421332384654974, 1.000000000000000000 ) ) ;
#24685=ORIENTED_EDGE ( 'NONE', *, *, #14043, .F. ) ;
#24689=CARTESIAN_POINT ( 'NONE',  ( 23.96296185032708337, 19.82388608118420237, 1.000000000000000000 ) ) ;
#24690=ORIENTED_EDGE ( 'NONE', *, *, #15086, .F. ) ;
#24692=CIRCLE ( 'NONE', #5479, 0.4999999999999991673 ) ;
#24695=ORIENTED_EDGE ( 'NONE', *, *, #6590, .T. ) ;
#24696=VERTEX_POINT ( 'NONE', #19201 ) ;
#24697=FACE_OUTER_BOUND ( 'NONE', #24622, .T. ) ;
#24702=CIRCLE ( 'NONE', #13003, 0.5000000000000004441 ) ;
#24704=DIRECTION ( 'NONE',  ( 1.000000000000000000, 0.000000000000000000, 0.000000000000000000 ) ) ;
#24707=DIRECTION ( 'NONE',  ( 0.000000000000000000, 0.000000000000000000, 1.000000000000000000 ) ) ;
#24711=DIRECTION ( 'NONE',  ( 1.000000000000000000, 0.000000000000000000, 0.000000000000000000 ) ) ;
#24714=VECTOR ( 'NONE', #25579, 1000.000000000000000 ) ;
#24715=CARTESIAN_POINT ( 'NONE',  ( 0.000000000000000000, 0.000000000000000000, 1.000000000000000000 ) ) ;
#24716=EDGE_CURVE ( 'NONE', #24827, #15870, #19688, .T. ) ;
#24717=AXIS2_PLACEMENT_3D ( 'NONE', #15453, #25134, #24996 ) ;
#24719=LINE ( 'NONE', #4721, #6226 ) ;
#24722=CYLINDRICAL_SURFACE ( 'NONE', #15022, 31.10000000000000142 ) ;
#24723=DIRECTION ( 'NONE',  ( 0.000000000000000000, 0.000000000000000000, 1.000000000000000000 ) ) ;
#24725=EDGE_CURVE ( 'NONE', #5826, #23600, #8430, .T. ) ;
#24726=CIRCLE ( 'NONE', #5919, 0.5000000000000003331 ) ;
#24729=EDGE_LOOP ( 'NONE', ( #25145, #11500, #4881, #2781 ) ) ;
#24730=VERTEX_POINT ( 'NONE', #12383 ) ;
#24731=DIRECTION ( 'NONE',  ( 0.000000000000000000, 0.000000000000000000, -1.000000000000000000 ) ) ;
#24732=CIRCLE ( 'NONE', #12199, 31.10000000000000142 ) ;
#24733=ORIENTED_EDGE ( 'NONE', *, *, #23084, .F. ) ;
#24734=DIRECTION ( 'NONE',  ( 0.000000000000000000, 0.000000000000000000, 1.000000000000000000 ) ) ;
#24736=AXIS2_PLACEMENT_3D ( 'NONE', #1891, #17837, #25806 ) ;
#24737=AXIS2_PLACEMENT_3D ( 'NONE', #23142, #19076, #3243 ) ;
#24739=LINE ( 'NONE', #20681, #4176 ) ;
#24749=DIRECTION ( 'NONE',  ( 0.000000000000000000, 0.000000000000000000, -1.000000000000000000 ) ) ;
#24753=AXIS2_PLACEMENT_3D ( 'NONE', #18293, #20509, #2850 ) ;
#24756=ORIENTED_EDGE ( 'NONE', *, *, #4093, .T. ) ;
#24758=CIRCLE ( 'NONE', #23100, 0.4999999999999998890 ) ;
#24759=ORIENTED_EDGE ( 'NONE', *, *, #13059, .T. ) ;
#24761=VERTEX_POINT ( 'NONE', #10284 ) ;
#24766=ORIENTED_EDGE ( 'NONE', *, *, #11921, .F. ) ;
#24767=DIRECTION ( 'NONE',  ( -0.9980267284282710039, 0.06279051952932233893, 0.000000000000000000 ) ) ;
#24775=DIRECTION ( 'NONE',  ( 1.000000000000000000, 0.000000000000000000, 0.000000000000000000 ) ) ;
#24777=AXIS2_PLACEMENT_3D ( 'NONE', #12963, #7068, #24474 ) ;
#24782=AXIS2_PLACEMENT_3D ( 'NONE', #8321, #14475, #18536 ) ;
#24784=ADVANCED_FACE ( 'NONE', ( #20102 ), #5857, .F. ) ;
#24786=CARTESIAN_POINT ( 'NONE',  ( 13.69242354489134073, -27.92360179968382283, -2.750000000000000000 ) ) ;
#24787=CARTESIAN_POINT ( 'NONE',  ( 0.000000000000000000, 0.000000000000000000, 1.000000000000000000 ) ) ;
#24789=ORIENTED_EDGE ( 'NONE', *, *, #23372, .T. ) ;
#24790=DIRECTION ( 'NONE',  ( 0.000000000000000000, 0.000000000000000000, -1.000000000000000000 ) ) ;
#24791=CARTESIAN_POINT ( 'NONE',  ( 0.000000000000000000, 0.000000000000000000, -6.500000000000000000 ) ) ;
#24794=FACE_OUTER_BOUND ( 'NONE', #6214, .T. ) ;
#24796=VECTOR ( 'NONE', #21193, 1000.000000000000000 ) ;
#24799=CIRCLE ( 'NONE', #20192, 31.10000000000000142 ) ;
#24805=LINE ( 'NONE', #20619, #24614 ) ;
#24806=CARTESIAN_POINT ( 'NONE',  ( -14.98253926456298579, 27.25313774936435962, 1.000000000000000000 ) ) ;
#24808=DIRECTION ( 'NONE',  ( -0.9822872507286872779, 0.1873813145857327056, 0.000000000000000000 ) ) ;
#24815=CARTESIAN_POINT ( 'NONE',  ( 0.000000000000000000, 0.000000000000000000, -6.500000000000000000 ) ) ;
#24819=VERTEX_POINT ( 'NONE', #16323 ) ;
#24820=DIRECTION ( 'NONE',  ( -0.000000000000000000, 0.000000000000000000, 1.000000000000000000 ) ) ;
#24824=ORIENTED_EDGE ( 'NONE', *, *, #907, .F. ) ;
#24826=EDGE_CURVE ( 'NONE', #15121, #2787, #19296, .T. ) ;
#24827=VERTEX_POINT ( 'NONE', #24292 ) ;
#24829=VERTEX_POINT ( 'NONE', #14367 ) ;
#24830=EDGE_LOOP ( 'NONE', ( #22610, #11235, #6178, #8287 ) ) ;
#24831=ADVANCED_FACE ( 'NONE', ( #16185 ), #24151, .T. ) ;
#24832=DIRECTION ( 'NONE',  ( -0.8443279255020122998, 0.5358267949790012086, 0.000000000000000000 ) ) ;
#24834=FACE_OUTER_BOUND ( 'NONE', #8917, .T. ) ;
#24840=DIRECTION ( 'NONE',  ( 1.000000000000000000, 0.000000000000000000, 0.000000000000000000 ) ) ;
#24844=DIRECTION ( 'NONE',  ( 0.000000000000000000, 0.000000000000000000, 1.000000000000000000 ) ) ;
#24845=CARTESIAN_POINT ( 'NONE',  ( 0.000000000000000000, 0.000000000000000000, 1.000000000000000000 ) ) ;
#24846=FACE_OUTER_BOUND ( 'NONE', #22701, .T. ) ;
#24852=LINE ( 'NONE', #21308, #21840 ) ;
#24853=EDGE_LOOP ( 'NONE', ( #17012, #12597, #12459, #21835 ) ) ;
#24857=ORIENTED_EDGE ( 'NONE', *, *, #15739, .F. ) ;
#24860=VERTEX_POINT ( 'NONE', #5990 ) ;
#24864=DIRECTION ( 'NONE',  ( 0.000000000000000000, 0.000000000000000000, 1.000000000000000000 ) ) ;
#24873=CIRCLE ( 'NONE', #23609, 0.5000000000000004441 ) ;
#24878=CARTESIAN_POINT ( 'NONE',  ( -16.66421332384701515, -26.25859848311253941, -6.500000000000000000 ) ) ;
#24880=CARTESIAN_POINT ( 'NONE',  ( -28.14012133169333651, -13.24173596767349359, -6.500000000000000000 ) ) ;
#24881=EDGE_CURVE ( 'NONE', #10033, #23656, #16848, .T. ) ;
#24883=ORIENTED_EDGE ( 'NONE', *, *, #853, .T. ) ;
#24884=EDGE_LOOP ( 'NONE', ( #15745, #17894, #20770, #9419 ) ) ;
#24888=CIRCLE ( 'NONE', #19033, 0.4999999999999999445 ) ;
#24889=CARTESIAN_POINT ( 'NONE',  ( -22.67092431280563503, 21.28941499438250062, 1.000000000000000000 ) ) ;
#24891=CARTESIAN_POINT ( 'NONE',  ( -13.24173596767398742, -28.14012133169310559, -6.500000000000000000 ) ) ;
#24896=DIRECTION ( 'NONE',  ( 0.000000000000000000, 0.000000000000000000, 1.000000000000000000 ) ) ;
#24905=CYLINDRICAL_SURFACE ( 'NONE', #4076, 31.10000000000000142 ) ;
#24914=ORIENTED_EDGE ( 'NONE', *, *, #6019, .T. ) ;
#24916=LINE ( 'NONE', #14976, #17490 ) ;
#24922=CARTESIAN_POINT ( 'NONE',  ( 2.451530025009136970, 31.00322564728514152, -6.500000000000000000 ) ) ;
#24924=EDGE_CURVE ( 'NONE', #14667, #4479, #12906, .T. ) ;
#24927=DIRECTION ( 'NONE',  ( 0.8090169943749532244, 0.5877852522924652545, 0.000000000000000000 ) ) ;
#24942=CARTESIAN_POINT ( 'NONE',  ( -31.03863125411927371, -1.952785157361310198, -6.500000000000000000 ) ) ;
#24948=ORIENTED_EDGE ( 'NONE', *, *, #23689, .T. ) ;
#24953=EDGE_CURVE ( 'NONE', #21593, #19594, #13037, .T. ) ;
#24962=CARTESIAN_POINT ( 'NONE',  ( 0.000000000000000000, 0.000000000000000000, -6.500000000000000000 ) ) ;
#24965=DIRECTION ( 'NONE',  ( 0.000000000000000000, 0.000000000000000000, 1.000000000000000000 ) ) ;
#24970=DIRECTION ( 'NONE',  ( 0.000000000000000000, 0.000000000000000000, -1.000000000000000000 ) ) ;
#24973=DIRECTION ( 'NONE',  ( 0.4257792915650852050, 0.9048270524660135816, 0.000000000000000000 ) ) ;
#24974=CARTESIAN_POINT ( 'NONE',  ( -10.94867358849371541, -28.91604871112453168, -6.500000000000000000 ) ) ;
#24977=CIRCLE ( 'NONE', #17048, 31.10000000000000142 ) ;
#24978=ORIENTED_EDGE ( 'NONE', *, *, #16544, .F. ) ;
#24980=ORIENTED_EDGE ( 'NONE', *, *, #14571, .F. ) ;
#24981=DIRECTION ( 'NONE',  ( 0.5877852522924730261, -0.8090169943749474513, 0.000000000000000000 ) ) ;
#24983=CIRCLE ( 'NONE', #22894, 31.10000000000000142 ) ;
#24984=ORIENTED_EDGE ( 'NONE', *, *, #10657, .T. ) ;
#24996=DIRECTION ( 'NONE',  ( 1.000000000000000000, 0.000000000000000000, 0.000000000000000000 ) ) ;
#24997=CARTESIAN_POINT ( 'NONE',  ( -31.09598070739550835, -0.4999838450256507416, -6.500000000000000000 ) ) ;
#25000=AXIS2_PLACEMENT_3D ( 'NONE', #1295, #11484, #25232 ) ;
#25001=FACE_OUTER_BOUND ( 'NONE', #17972, .T. ) ;
#25003=EDGE_CURVE ( 'NONE', #16624, #13717, #10118, .T. ) ;
#25007=CARTESIAN_POINT ( 'NONE',  ( -30.10000000000000142, 3.686186865433532535E-15, -6.500000000000000000 ) ) ;
#25012=VECTOR ( 'NONE', #11157, 1000.000000000000000 ) ;
#25013=ORIENTED_EDGE ( 'NONE', *, *, #24631, .F. ) ;
#25014=AXIS2_PLACEMENT_3D ( 'NONE', #2828, #14607, #8470 ) ;
#25015=DIRECTION ( 'NONE',  ( 1.000000000000000000, 0.000000000000000000, 0.000000000000000000 ) ) ;
#25018=AXIS2_PLACEMENT_3D ( 'NONE', #17338, #13153, #8972 ) ;
#25021=LINE ( 'NONE', #7109, #2483 ) ;
#25026=DIRECTION ( 'NONE',  ( -0.000000000000000000, 0.000000000000000000, 1.000000000000000000 ) ) ;
#25032=VECTOR ( 'NONE', #21875, 1000.000000000000000 ) ;
#25034=ADVANCED_FACE ( 'NONE', ( #489 ), #24137, .F. ) ;
#25035=CARTESIAN_POINT ( 'NONE',  ( 17.08421000182759997, -25.98730014090448392, -6.500000000000000000 ) ) ;
#25036=CIRCLE ( 'NONE', #2919, 0.5000000000000000000 ) ;
#25040=ORIENTED_EDGE ( 'NONE', *, *, #998, .T. ) ;
#25044=VECTOR ( 'NONE', #1200, 1000.000000000000000 ) ;
#25049=CIRCLE ( 'NONE', #16689, 0.5000000000000001110 ) ;
#25050=CIRCLE ( 'NONE', #5834, 0.5000000000000003331 ) ;
#25054=AXIS2_PLACEMENT_3D ( 'NONE', #2912, #5145, #19114 ) ;
#25057=DIRECTION ( 'NONE',  ( -0.000000000000000000, -0.000000000000000000, 1.000000000000000000 ) ) ;
#25059=CIRCLE ( 'NONE', #9601, 0.5000000000000003331 ) ;
#25063=EDGE_CURVE ( 'NONE', #10717, #3169, #12494, .T. ) ;
#25066=CIRCLE ( 'NONE', #6675, 31.10000000000000142 ) ;
#25067=DIRECTION ( 'NONE',  ( 1.000000000000000000, 0.000000000000000000, 0.000000000000000000 ) ) ;
#25071=EDGE_LOOP ( 'NONE', ( #12031, #615, #10721, #10993 ) ) ;
#25078=CIRCLE ( 'NONE', #31, 0.5000000000000000000 ) ;
#25080=ORIENTED_EDGE ( 'NONE', *, *, #15873, .F. ) ;
#25083=EDGE_LOOP ( 'NONE', ( #14755, #2373, #6446, #8673 ) ) ;
#25086=ADVANCED_FACE ( 'NONE', ( #14214 ), #16307, .T. ) ;
#25087=CIRCLE ( 'NONE', #2531, 31.10000000000000142 ) ;
#25092=CARTESIAN_POINT ( 'NONE',  ( 11.91206721063039886, 28.72825533807133169, 1.000000000000000000 ) ) ;
#25093=VECTOR ( 'NONE', #22753, 1000.000000000000000 ) ;
#25098=CARTESIAN_POINT ( 'NONE',  ( 23.01025686871630782, -20.92219106202058754, -2.750000000000000000 ) ) ;
#25099=CARTESIAN_POINT ( 'NONE',  ( -19.32388608118395013, 23.96296185032730364, 1.000000000000000000 ) ) ;
#25104=DIRECTION ( 'NONE',  ( 0.000000000000000000, 0.000000000000000000, 1.000000000000000000 ) ) ;
#25105=CARTESIAN_POINT ( 'NONE',  ( -19.43607991388954304, 24.27856662945528399, -2.750000000000000000 ) ) ;
#25107=CARTESIAN_POINT ( 'NONE',  ( -28.14012133169306296, 13.24173596767408867, 1.000000000000000000 ) ) ;
#25110=EDGE_CURVE ( 'NONE', #7791, #10324, #21397, .T. ) ;
#25113=VERTEX_POINT ( 'NONE', #22439 ) ;
#25115=DIRECTION ( 'NONE',  ( 1.000000000000000000, 0.000000000000000000, 0.000000000000000000 ) ) ;
#25118=EDGE_CURVE ( 'NONE', #17279, #20930, #8442, .T. ) ;
#25125=EDGE_CURVE ( 'NONE', #21178, #6707, #106, .T. ) ;
#25128=VECTOR ( 'NONE', #24606, 1000.000000000000000 ) ;
#25129=DIRECTION ( 'NONE',  ( 0.000000000000000000, -0.000000000000000000, 1.000000000000000000 ) ) ;
#25130=CARTESIAN_POINT ( 'NONE',  ( 27.25313774936409317, -14.98253926456347074, -6.500000000000000000 ) ) ;
#25132=DIRECTION ( 'NONE',  ( 0.8443279255020205154, 0.5358267949789882190, 0.000000000000000000 ) ) ;
#25133=CARTESIAN_POINT ( 'NONE',  ( -30.85476721088022600, 3.897863563850190616, -6.500000000000000000 ) ) ;
#25134=DIRECTION ( 'NONE',  ( 0.000000000000000000, 0.000000000000000000, 1.000000000000000000 ) ) ;
#25136=AXIS2_PLACEMENT_3D ( 'NONE', #19580, #1684, #9660 ) ;
#25137=DIRECTION ( 'NONE',  ( 1.000000000000000000, 0.000000000000000000, 0.000000000000000000 ) ) ;
#25138=DIRECTION ( 'NONE',  ( 0.000000000000000000, -0.000000000000000000, -1.000000000000000000 ) ) ;
#25140=EDGE_CURVE ( 'NONE', #7323, #7998, #5940, .T. ) ;
#25143=ORIENTED_EDGE ( 'NONE', *, *, #2268, .T. ) ;
#25145=ORIENTED_EDGE ( 'NONE', *, *, #10822, .F. ) ;
#25148=LINE ( 'NONE', #17693, #7596 ) ;
#25150=AXIS2_PLACEMENT_3D ( 'NONE', #7047, #3380, #19337 ) ;
#25151=ADVANCED_FACE ( 'NONE', ( #17076 ), #8702, .T. ) ;
#25152=VERTEX_POINT ( 'NONE', #3085 ) ;
#25154=CIRCLE ( 'NONE', #13874, 31.10000000000000142 ) ;
#25159=AXIS2_PLACEMENT_3D ( 'NONE', #20863, #15248, #9089 ) ;
#25160=CARTESIAN_POINT ( 'NONE',  ( 17.08421000182777760, 25.98730014090436313, -2.750000000000000000 ) ) ;
#25161=CARTESIAN_POINT ( 'NONE',  ( -25.98730014090454432, -17.08421000182750760, -2.750000000000000000 ) ) ;
#25175=ORIENTED_EDGE ( 'NONE', *, *, #6913, .T. ) ;
#25178=LINE ( 'NONE', #6734, #22973 ) ;
#25179=VERTEX_POINT ( 'NONE', #20437 ) ;
#25182=CIRCLE ( 'NONE', #4282, 31.10000000000000142 ) ;
#25184=VERTEX_POINT ( 'NONE', #10359 ) ;
#25186=CYLINDRICAL_SURFACE ( 'NONE', #7196, 0.5000000000000004441 ) ;
#25188=AXIS2_PLACEMENT_3D ( 'NONE', #23528, #21827, #25620 ) ;
#25191=ADVANCED_FACE ( 'NONE', ( #14324 ), #10504, .F. ) ;
#25192=ADVANCED_FACE ( 'NONE', ( #19917 ), #6581, .T. ) ;
#25193=AXIS2_PLACEMENT_3D ( 'NONE', #3266, #13724, #23278 ) ;
#25196=CARTESIAN_POINT ( 'NONE',  ( 0.000000000000000000, 0.000000000000000000, -6.500000000000000000 ) ) ;
#25199=CIRCLE ( 'NONE', #565, 31.10000000000000142 ) ;
#25210=ORIENTED_EDGE ( 'NONE', *, *, #20422, .F. ) ;
#25213=DIRECTION ( 'NONE',  ( 0.000000000000000000, 0.000000000000000000, 1.000000000000000000 ) ) ;
#25216=ORIENTED_EDGE ( 'NONE', *, *, #16798, .F. ) ;
#25222=AXIS2_PLACEMENT_3D ( 'NONE', #7104, #10751, #14951 ) ;
#25224=EDGE_CURVE ( 'NONE', #10602, #15596, #5535, .T. ) ;
#25227=DIRECTION ( 'NONE',  ( 0.000000000000000000, -0.000000000000000000, -1.000000000000000000 ) ) ;
#25228=DIRECTION ( 'NONE',  ( 0.000000000000000000, 0.000000000000000000, 1.000000000000000000 ) ) ;
#25230=CYLINDRICAL_SURFACE ( 'NONE', #19931, 31.10000000000000142 ) ;
#25232=DIRECTION ( 'NONE',  ( -0.9510565162951561957, -0.3090169943749392911, 0.000000000000000000 ) ) ;
#25235=DIRECTION ( 'NONE',  ( 0.000000000000000000, 0.000000000000000000, 1.000000000000000000 ) ) ;
#25236=CYLINDRICAL_SURFACE ( 'NONE', #6200, 31.10000000000000142 ) ;
#25237=ADVANCED_FACE ( 'NONE', ( #20308 ), #9986, .T. ) ;
#25239=CARTESIAN_POINT ( 'NONE',  ( -16.16421332384701515, -26.25859848311253941, -6.500000000000000000 ) ) ;
#25242=DIRECTION ( 'NONE',  ( 0.9921147013144794302, 0.1253332335642911299, 0.000000000000000000 ) ) ;
#25243=DIRECTION ( 'NONE',  ( 0.000000000000000000, 0.000000000000000000, 1.000000000000000000 ) ) ;
#25245=ORIENTED_EDGE ( 'NONE', *, *, #1870, .T. ) ;
#25247=VERTEX_POINT ( 'NONE', #22020 ) ;
#25248=EDGE_LOOP ( 'NONE', ( #15532, #240, #20018, #16764 ) ) ;
#25249=DIRECTION ( 'NONE',  ( 0.4817536741017131585, -0.8763066800438648052, 0.000000000000000000 ) ) ;
#25250=DIRECTION ( 'NONE',  ( 0.000000000000000000, 0.000000000000000000, 1.000000000000000000 ) ) ;
#25255=DIRECTION ( 'NONE',  ( 0.000000000000000000, -0.000000000000000000, -1.000000000000000000 ) ) ;
#25257=DIRECTION ( 'NONE',  ( 0.000000000000000000, 0.000000000000000000, 1.000000000000000000 ) ) ;
#25260=EDGE_CURVE ( 'NONE', #8556, #2078, #5150, .T. ) ;
#25261=DIRECTION ( 'NONE',  ( 0.000000000000000000, 0.000000000000000000, 1.000000000000000000 ) ) ;
#25262=DIRECTION ( 'NONE',  ( 0.000000000000000000, 0.000000000000000000, 1.000000000000000000 ) ) ;
#25265=CARTESIAN_POINT ( 'NONE',  ( 7.248980000273979485, -30.24338421796786847, -2.750000000000000000 ) ) ;
#25267=CARTESIAN_POINT ( 'NONE',  ( 0.000000000000000000, 0.000000000000000000, -6.500000000000000000 ) ) ;
#25268=EDGE_LOOP ( 'NONE', ( #19473, #2752, #25143, #17483 ) ) ;
#25269=CARTESIAN_POINT ( 'NONE',  ( 0.000000000000000000, 0.000000000000000000, -6.500000000000000000 ) ) ;
#25271=EDGE_CURVE ( 'NONE', #12169, #10041, #968, .T. ) ;
#25279=ORIENTED_EDGE ( 'NONE', *, *, #24020, .T. ) ;
#25282=CARTESIAN_POINT ( 'NONE',  ( -26.25859848311282363, -16.66421332384654974, -6.500000000000000000 ) ) ;
#25283=CARTESIAN_POINT ( 'NONE',  ( -25.16042852506104666, -18.28012134629567598, -6.500000000000000000 ) ) ;
#25290=CARTESIAN_POINT ( 'NONE',  ( 0.000000000000000000, 0.000000000000000000, -6.500000000000000000 ) ) ;
#25291=VERTEX_POINT ( 'NONE', #22929 ) ;
#25292=EDGE_LOOP ( 'NONE', ( #12369, #10716, #10992, #18943 ) ) ;
#25293=EDGE_CURVE ( 'NONE', #6766, #11648, #16425, .T. ) ;
#25295=CARTESIAN_POINT ( 'NONE',  ( -28.91604871112473418, -11.44867358849319849, 1.000000000000000000 ) ) ;
#25296=VERTEX_POINT ( 'NONE', #18744 ) ;
#25297=CARTESIAN_POINT ( 'NONE',  ( -20.20656826142249685, 23.64116323484259752, -2.750000000000000000 ) ) ;
#25298=AXIS2_PLACEMENT_3D ( 'NONE', #16238, #21992, #24210 ) ;
#25304=FACE_OUTER_BOUND ( 'NONE', #21949, .T. ) ;
#25305=DIRECTION ( 'NONE',  ( 1.000000000000000000, 0.000000000000000000, 0.000000000000000000 ) ) ;
#25306=ORIENTED_EDGE ( 'NONE', *, *, #17018, .T. ) ;
#25307=CARTESIAN_POINT ( 'NONE',  ( -29.57785765677936851, -9.610428525060582317, -6.500000000000000000 ) ) ;
#25308=CARTESIAN_POINT ( 'NONE',  ( 0.000000000000000000, 0.000000000000000000, -6.500000000000000000 ) ) ;
#25310=DIRECTION ( 'NONE',  ( 0.000000000000000000, 0.000000000000000000, 1.000000000000000000 ) ) ;
#25313=DIRECTION ( 'NONE',  ( 0.000000000000000000, 0.000000000000000000, 1.000000000000000000 ) ) ;
#25314=CARTESIAN_POINT ( 'NONE',  ( -11.44867358849371541, -28.91604871112453168, -6.500000000000000000 ) ) ;
#25317=CARTESIAN_POINT ( 'NONE',  ( -11.91206721063060670, -28.72825533807125353, 1.000000000000000000 ) ) ;
#25320=DIRECTION ( 'NONE',  ( -0.000000000000000000, 0.000000000000000000, 1.000000000000000000 ) ) ;
#25326=FACE_OUTER_BOUND ( 'NONE', #22798, .T. ) ;
#25329=EDGE_CURVE ( 'NONE', #20576, #9975, #3054, .T. ) ;
#25336=ORIENTED_EDGE ( 'NONE', *, *, #18971, .T. ) ;
#25337=ORIENTED_EDGE ( 'NONE', *, *, #9146, .F. ) ;
#25338=FACE_OUTER_BOUND ( 'NONE', #13840, .T. ) ;
#25344=DIRECTION ( 'NONE',  ( 0.000000000000000000, 0.000000000000000000, 1.000000000000000000 ) ) ;
#25346=DIRECTION ( 'NONE',  ( 0.000000000000000000, 0.000000000000000000, 1.000000000000000000 ) ) ;
#25347=ORIENTED_EDGE ( 'NONE', *, *, #13029, .T. ) ;
#25352=DIRECTION ( 'NONE',  ( 0.000000000000000000, 0.000000000000000000, 1.000000000000000000 ) ) ;
#25357=DIRECTION ( 'NONE',  ( 0.06279051952930848890, -0.9980267284282718920, 0.000000000000000000 ) ) ;
#25358=DIRECTION ( 'NONE',  ( 0.000000000000000000, 0.000000000000000000, 1.000000000000000000 ) ) ;
#25359=VERTEX_POINT ( 'NONE', #16928 ) ;
#25360=EDGE_CURVE ( 'NONE', #7582, #822, #6821, .T. ) ;
#25361=ORIENTED_EDGE ( 'NONE', *, *, #6132, .F. ) ;
#25363=EDGE_LOOP ( 'NONE', ( #11502, #10944, #11530, #17612 ) ) ;
#25364=VERTEX_POINT ( 'NONE', #12741 ) ;
#25365=CARTESIAN_POINT ( 'NONE',  ( -21.28941499438192864, 22.67092431280617859, -6.500000000000000000 ) ) ;
#25368=ADVANCED_FACE ( 'NONE', ( #5016 ), #2672, .F. ) ;
#25371=DIRECTION ( 'NONE',  ( 0.000000000000000000, 0.000000000000000000, -1.000000000000000000 ) ) ;
#25377=CARTESIAN_POINT ( 'NONE',  ( 4.393401135981119587, 30.78811501957143193, -6.500000000000000000 ) ) ;
#25378=CARTESIAN_POINT ( 'NONE',  ( 25.98730014090437734, -17.08421000182775984, 1.000000000000000000 ) ) ;
#25382=AXIS2_PLACEMENT_3D ( 'NONE', #7692, #9515, #5718 ) ;
#25386=LINE ( 'NONE', #3426, #25044 ) ;
#25389=ORIENTED_EDGE ( 'NONE', *, *, #16029, .T. ) ;
#25390=DIRECTION ( 'NONE',  ( 1.000000000000000000, 0.000000000000000000, 0.000000000000000000 ) ) ;
#25391=ORIENTED_EDGE ( 'NONE', *, *, #7631, .T. ) ;
#25393=ORIENTED_EDGE ( 'NONE', *, *, #5551, .F. ) ;
#25394=FACE_OUTER_BOUND ( 'NONE', #14854, .T. ) ;
#25399=EDGE_CURVE ( 'NONE', #789, #21593, #23693, .T. ) ;
#25400=LINE ( 'NONE', #25160, #23439 ) ;
#25404=AXIS2_PLACEMENT_3D ( 'NONE', #24605, #18481, #12839 ) ;
#25407=DIRECTION ( 'NONE',  ( 1.000000000000000000, 0.000000000000000000, 0.000000000000000000 ) ) ;
#25408=ORIENTED_EDGE ( 'NONE', *, *, #24459, .T. ) ;
#25412=ORIENTED_EDGE ( 'NONE', *, *, #6680, .F. ) ;
#25414=CIRCLE ( 'NONE', #12461, 31.10000000000000142 ) ;
#25419=AXIS2_PLACEMENT_3D ( 'NONE', #13406, #7264, #15358 ) ;
#25421=CARTESIAN_POINT ( 'NONE',  ( 9.133673601486471227, 29.72853858738282185, -6.500000000000000000 ) ) ;
#25422=AXIS2_PLACEMENT_3D ( 'NONE', #1467, #17547, #25521 ) ;
#25423=VERTEX_POINT ( 'NONE', #19504 ) ;
#25427=ADVANCED_FACE ( 'NONE', ( #17562 ), #3821, .T. ) ;
#25430=AXIS2_PLACEMENT_3D ( 'NONE', #3103, #11068, #14615 ) ;
#25434=VECTOR ( 'NONE', #24386, 1000.000000000000000 ) ;
#25435=CARTESIAN_POINT ( 'NONE',  ( 26.52310962334739486, -16.23990935651726275, 1.000000000000000000 ) ) ;
#25437=VECTOR ( 'NONE', #4574, 1000.000000000000000 ) ;
#25445=AXIS2_PLACEMENT_3D ( 'NONE', #5517, #25524, #7350 ) ;
#25447=VERTEX_POINT ( 'NONE', #9574 ) ;
#25449=EDGE_CURVE ( 'NONE', #19514, #24761, #560, .T. ) ;
#25451=CARTESIAN_POINT ( 'NONE',  ( 1.952785157361432100, -31.03863125411925949, -6.500000000000000000 ) ) ;
#25452=VERTEX_POINT ( 'NONE', #25537 ) ;
#25456=AXIS2_PLACEMENT_3D ( 'NONE', #929, #3254, #5231 ) ;
#25463=CIRCLE ( 'NONE', #14192, 0.5000000000000001110 ) ;
#25464=CARTESIAN_POINT ( 'NONE',  ( 10.08469938919477649, -29.41953157733097868, -2.750000000000000000 ) ) ;
#25465=EDGE_CURVE ( 'NONE', #12169, #1343, #8488, .T. ) ;
#25466=AXIS2_PLACEMENT_3D ( 'NONE', #1052, #21311, #14916 ) ;
#25470=DIRECTION ( 'NONE',  ( -0.000000000000000000, 0.000000000000000000, 1.000000000000000000 ) ) ;
#25473=CARTESIAN_POINT ( 'NONE',  ( 23.96296185032695192, -19.82388608118436935, -6.500000000000000000 ) ) ;
#25477=DIRECTION ( 'NONE',  ( 1.000000000000000000, 0.000000000000000000, 0.000000000000000000 ) ) ;
#25478=DIRECTION ( 'NONE',  ( -0.6845471059286831750, 0.7289686274214168815, 0.000000000000000000 ) ) ;
#25479=ORIENTED_EDGE ( 'NONE', *, *, #15711, .F. ) ;
#25483=AXIS2_PLACEMENT_3D ( 'NONE', #11512, #7337, #19363 ) ;
#25484=DIRECTION ( 'NONE',  ( 1.000000000000000000, 0.000000000000000000, 0.000000000000000000 ) ) ;
#25487=VERTEX_POINT ( 'NONE', #21606 ) ;
#25496=ORIENTED_EDGE ( 'NONE', *, *, #539, .F. ) ;
#25502=VECTOR ( 'NONE', #25227, 1000.000000000000000 ) ;
#25505=EDGE_CURVE ( 'NONE', #16708, #15212, #11537, .T. ) ;
#25513=DIRECTION ( 'NONE',  ( 0.000000000000000000, -0.000000000000000000, 1.000000000000000000 ) ) ;
#25514=DIRECTION ( 'NONE',  ( 0.000000000000000000, 0.000000000000000000, 1.000000000000000000 ) ) ;
#25519=CIRCLE ( 'NONE', #7132, 0.4999999999999995004 ) ;
#25521=DIRECTION ( 'NONE',  ( 1.000000000000000000, 0.000000000000000000, 0.000000000000000000 ) ) ;
#25524=DIRECTION ( 'NONE',  ( 0.000000000000000000, 0.000000000000000000, 1.000000000000000000 ) ) ;
#25525=ORIENTED_EDGE ( 'NONE', *, *, #14100, .F. ) ;
#25528=DIRECTION ( 'NONE',  ( 0.000000000000000000, 0.000000000000000000, 1.000000000000000000 ) ) ;
#25532=VERTEX_POINT ( 'NONE', #11802 ) ;
#25537=CARTESIAN_POINT ( 'NONE',  ( -30.53863125411922752, 1.952785157361987878, -6.500000000000000000 ) ) ;
#25538=AXIS2_PLACEMENT_3D ( 'NONE', #2977, #4684, #10945 ) ;
#25539=VECTOR ( 'NONE', #6690, 1000.000000000000000 ) ;
#25540=CARTESIAN_POINT ( 'NONE',  ( 28.91604871112457076, -11.44867358849361416, 1.000000000000000000 ) ) ;
#25543=EDGE_CURVE ( 'NONE', #8796, #12340, #5977, .T. ) ;
#25544=DIRECTION ( 'NONE',  ( 0.000000000000000000, 0.000000000000000000, 1.000000000000000000 ) ) ;
#25545=EDGE_CURVE ( 'NONE', #13257, #9975, #17698, .T. ) ;
#25550=VERTEX_POINT ( 'NONE', #13249 ) ;
#25553=AXIS2_PLACEMENT_3D ( 'NONE', #21528, #13439, #17477 ) ;
#25554=AXIS2_PLACEMENT_3D ( 'NONE', #13125, #1601, #21095 ) ;
#25559=DIRECTION ( 'NONE',  ( 1.000000000000000000, 0.000000000000000000, 0.000000000000000000 ) ) ;
#25561=ORIENTED_EDGE ( 'NONE', *, *, #25604, .F. ) ;
#25562=VECTOR ( 'NONE', #18959, 1000.000000000000000 ) ;
#25563=LINE ( 'NONE', #5423, #20486 ) ;
#25564=VERTEX_POINT ( 'NONE', #7362 ) ;
#25566=DIRECTION ( 'NONE',  ( 0.000000000000000000, 0.000000000000000000, 1.000000000000000000 ) ) ;
#25568=AXIS2_PLACEMENT_3D ( 'NONE', #21321, #18180, #2222 ) ;
#25579=DIRECTION ( 'NONE',  ( 0.000000000000000000, 0.000000000000000000, -1.000000000000000000 ) ) ;
#25584=CARTESIAN_POINT ( 'NONE',  ( 0.000000000000000000, 0.000000000000000000, 1.000000000000000000 ) ) ;
#25589=ORIENTED_EDGE ( 'NONE', *, *, #21913, .F. ) ;
#25590=ADVANCED_FACE ( 'NONE', ( #14926 ), #22897, .T. ) ;
#25593=DIRECTION ( 'NONE',  ( 0.000000000000000000, 0.000000000000000000, 1.000000000000000000 ) ) ;
#25597=ORIENTED_EDGE ( 'NONE', *, *, #19247, .T. ) ;
#25603=( NAMED_UNIT ( * ) SI_UNIT ( $, .STERADIAN. ) SOLID_ANGLE_UNIT ( ) );
#25604=EDGE_CURVE ( 'NONE', #24827, #13859, #20592, .T. ) ;
#25607=LINE ( 'NONE', #15284, #24281 ) ;
#25609=CARTESIAN_POINT ( 'NONE',  ( 20.20656826142266738, -23.64116323484245541, -2.750000000000000000 ) ) ;
#25612=ORIENTED_EDGE ( 'NONE', *, *, #24459, .F. ) ;
#25616=LINE ( 'NONE', #1824, #1186 ) ;
#25617=EDGE_CURVE ( 'NONE', #18972, #16823, #11821, .T. ) ;
#25620=DIRECTION ( 'NONE',  ( 1.000000000000000000, 0.000000000000000000, 0.000000000000000000 ) ) ;
#25621=EDGE_LOOP ( 'NONE', ( #4584, #4536, #17963, #17214 ) ) ;
#25626=ADVANCED_FACE ( 'NONE', ( #5626 ), #19603, .F. ) ;
#25629=ORIENTED_EDGE ( 'NONE', *, *, #7759, .F. ) ;
#25630=ORIENTED_EDGE ( 'NONE', *, *, #2505, .T. ) ;
#25633=DIRECTION ( 'NONE',  ( 0.000000000000000000, 0.000000000000000000, 1.000000000000000000 ) ) ;
#25635=DIRECTION ( 'NONE',  ( 0.9048270524660262382, 0.4257792915650585042, 0.000000000000000000 ) ) ;
#25646=DIRECTION ( 'NONE',  ( -0.9685831611286283005, 0.2486898871648657861, 0.000000000000000000 ) ) ;
#25650=CARTESIAN_POINT ( 'NONE',  ( -19.82388608118395013, 23.96296185032730364, -6.500000000000000000 ) ) ;
#25651=CARTESIAN_POINT ( 'NONE',  ( -27.64012133169306296, 13.24173596767408867, 1.000000000000000000 ) ) ;
#25652=CARTESIAN_POINT ( 'NONE',  ( 18.28012134629577190, -25.16042852506097205, -6.500000000000000000 ) ) ;
#25653=ORIENTED_EDGE ( 'NONE', *, *, #13308, .T. ) ;
#25658=CARTESIAN_POINT ( 'NONE',  ( 0.000000000000000000, 0.000000000000000000, -6.500000000000000000 ) ) ;
#25661=EDGE_CURVE ( 'NONE', #3018, #11616, #147, .T. ) ;
#25663=CARTESIAN_POINT ( 'NONE',  ( 0.000000000000000000, 0.000000000000000000, -6.500000000000000000 ) ) ;
#25664=ADVANCED_FACE ( 'NONE', ( #1452 ), #17526, .T. ) ;
#25667=EDGE_CURVE ( 'NONE', #21691, #25423, #21846, .T. ) ;
#25670=DIRECTION ( 'NONE',  ( 0.000000000000000000, 0.000000000000000000, 1.000000000000000000 ) ) ;
#25672=CARTESIAN_POINT ( 'NONE',  ( -30.54913349766215802, 5.827558883616378083, -6.500000000000000000 ) ) ;
#25676=DIRECTION ( 'NONE',  ( 1.000000000000000000, 0.000000000000000000, 0.000000000000000000 ) ) ;
#25677=CARTESIAN_POINT ( 'NONE',  ( 17.08421000182759997, -25.98730014090448392, -2.750000000000000000 ) ) ;
#25678=ORIENTED_EDGE ( 'NONE', *, *, #1575, .F. ) ;
#25687=EDGE_LOOP ( 'NONE', ( #13266, #9535, #24518, #18255 ) ) ;
#25689=DIRECTION ( 'NONE',  ( 0.000000000000000000, 0.000000000000000000, 1.000000000000000000 ) ) ;
#25700=VECTOR ( 'NONE', #4320, 1000.000000000000000 ) ;
#25701=AXIS2_PLACEMENT_3D ( 'NONE', #18850, #24734, #4736 ) ;
#25705=CYLINDRICAL_SURFACE ( 'NONE', #21777, 0.5000000000000004441 ) ;
#25706=CARTESIAN_POINT ( 'NONE',  ( 31.09598070739550479, -0.4999838450260850053, -2.750000000000000000 ) ) ;
#25710=ORIENTED_EDGE ( 'NONE', *, *, #18126, .T. ) ;
#25713=ORIENTED_EDGE ( 'NONE', *, *, #5842, .F. ) ;
#25715=CARTESIAN_POINT ( 'NONE',  ( -9.610428525060479288, 29.57785765677940404, -6.500000000000000000 ) ) ;
#25717=ORIENTED_EDGE ( 'NONE', *, *, #13013, .F. ) ;
#25718=DIRECTION ( 'NONE',  ( 0.000000000000000000, 0.000000000000000000, 1.000000000000000000 ) ) ;
#25721=LINE ( 'NONE', #17875, #18094 ) ;
#25723=EDGE_CURVE ( 'NONE', #485, #10079, #23936, .T. ) ;
#25727=DIRECTION ( 'NONE',  ( 0.000000000000000000, 0.000000000000000000, 1.000000000000000000 ) ) ;
#25744=ORIENTED_EDGE ( 'NONE', *, *, #4489, .T. ) ;
#25745=ORIENTED_EDGE ( 'NONE', *, *, #1122, .T. ) ;
#25750=DIRECTION ( 'NONE',  ( -0.000000000000000000, -0.000000000000000000, 1.000000000000000000 ) ) ;
#25751=EDGE_CURVE ( 'NONE', #23155, #7696, #1390, .T. ) ;
#25757=LINE ( 'NONE', #19225, #24796 ) ;
#25758=ADVANCED_FACE ( 'NONE', ( #18627 ), #12348, .F. ) ;
#25761=DIRECTION ( 'NONE',  ( 1.000000000000000000, 0.000000000000000000, 0.000000000000000000 ) ) ;
#25763=LINE ( 'NONE', #9814, #12103 ) ;
#25766=CYLINDRICAL_SURFACE ( 'NONE', #21805, 0.5000000000000004441 ) ;
#25769=DIRECTION ( 'NONE',  ( -0.3090169943749382919, 0.9510565162951566398, 0.000000000000000000 ) ) ;
#25771=FACE_OUTER_BOUND ( 'NONE', #700, .T. ) ;
#25774=ORIENTED_EDGE ( 'NONE', *, *, #22938, .T. ) ;
#25777=ORIENTED_EDGE ( 'NONE', *, *, #14835, .T. ) ;
#25779=ORIENTED_EDGE ( 'NONE', *, *, #9801, .F. ) ;
#25783=DIRECTION ( 'NONE',  ( 1.000000000000000000, 0.000000000000000000, 0.000000000000000000 ) ) ;
#25785=CARTESIAN_POINT ( 'NONE',  ( 30.10000000000000142, 0.000000000000000000, -6.500000000000000000 ) ) ;
#25787=ADVANCED_FACE ( 'NONE', ( #24597 ), #16771, .F. ) ;
#25789=DIRECTION ( 'NONE',  ( 1.000000000000000000, 0.000000000000000000, 0.000000000000000000 ) ) ;
#25800=ORIENTED_EDGE ( 'NONE', *, *, #5762, .T. ) ;
#25801=EDGE_LOOP ( 'NONE', ( #22769, #15298, #22331, #24128 ) ) ;
#25803=ORIENTED_EDGE ( 'NONE', *, *, #5630, .T. ) ;
#25804=DIRECTION ( 'NONE',  ( -0.000000000000000000, -0.000000000000000000, 1.000000000000000000 ) ) ;
#25806=DIRECTION ( 'NONE',  ( 1.000000000000000000, 0.000000000000000000, 0.000000000000000000 ) ) ;
#25807=CARTESIAN_POINT ( 'NONE',  ( 28.34936733434196299, -12.78762572734067149, -6.500000000000000000 ) ) ;
#25808=ORIENTED_EDGE ( 'NONE', *, *, #21422, .T. ) ;
#25810=AXIS2_PLACEMENT_3D ( 'NONE', #13502, #14008, #25769 ) ;
#25811=CARTESIAN_POINT ( 'NONE',  ( -11.44867358849371541, -28.91604871112453168, -6.500000000000000000 ) ) ;
#25814=FACE_OUTER_BOUND ( 'NONE', #17428, .T. ) ;
#25817=FACE_OUTER_BOUND ( 'NONE', #2984, .T. ) ;
#25818=CARTESIAN_POINT ( 'NONE',  ( 0.000000000000000000, 0.000000000000000000, -6.500000000000000000 ) ) ;
#25824=FACE_OUTER_BOUND ( 'NONE', #25801, .T. ) ;
#25836=ORIENTED_EDGE ( 'NONE', *, *, #3390, .T. ) ;
#25842=DIRECTION ( 'NONE',  ( 0.000000000000000000, 0.000000000000000000, 1.000000000000000000 ) ) ;
#25846=ORIENTED_EDGE ( 'NONE', *, *, #10581, .T. ) ;
#25850=CIRCLE ( 'NONE', #21258, 31.10000000000000142 ) ;
#25851=CIRCLE ( 'NONE', #807, 0.4999999999999997780 ) ;
#25852=CARTESIAN_POINT ( 'NONE',  ( 14.98253926456337837, 27.25313774936414291, -6.500000000000000000 ) ) ;
#25853=EDGE_CURVE ( 'NONE', #23233, #3781, #7334, .T. ) ;
#25855=DIRECTION ( 'NONE',  ( 0.000000000000000000, 0.000000000000000000, 1.000000000000000000 ) ) ;
#25856=FACE_OUTER_BOUND ( 'NONE', #17839, .T. ) ;
#25857=CARTESIAN_POINT ( 'NONE',  ( -25.16042852506064165, 18.28012134629622309, -6.500000000000000000 ) ) ;
#25866=EDGE_CURVE ( 'NONE', #14853, #1951, #25757, .T. ) ;
#25868=AXIS2_PLACEMENT_3D ( 'NONE', #11108, #1442, #2875 ) ;
#25874=CARTESIAN_POINT ( 'NONE',  ( -27.64012133169306296, 13.24173596767408867, -6.500000000000000000 ) ) ;
#25875=DIRECTION ( 'NONE',  ( 1.000000000000000000, 0.000000000000000000, 0.000000000000000000 ) ) ;
#25894=COLOUR_RGB('Light Blue',0.38,0.62,0.78);
#25895=FILL_AREA_STYLE_COLOUR('',#25894);
#25896=FILL_AREA_STYLE('',(#25895));
#25897=SURFACE_STYLE_FILL_AREA(#25896);
#25898=SURFACE_SIDE_STYLE('',(#25897));
#25899=SURFACE_STYLE_USAGE(.BOTH.,#25898);
#25900=PRESENTATION_STYLE_ASSIGNMENT((#25899));
ENDSEC;
END-ISO-10303-21;
